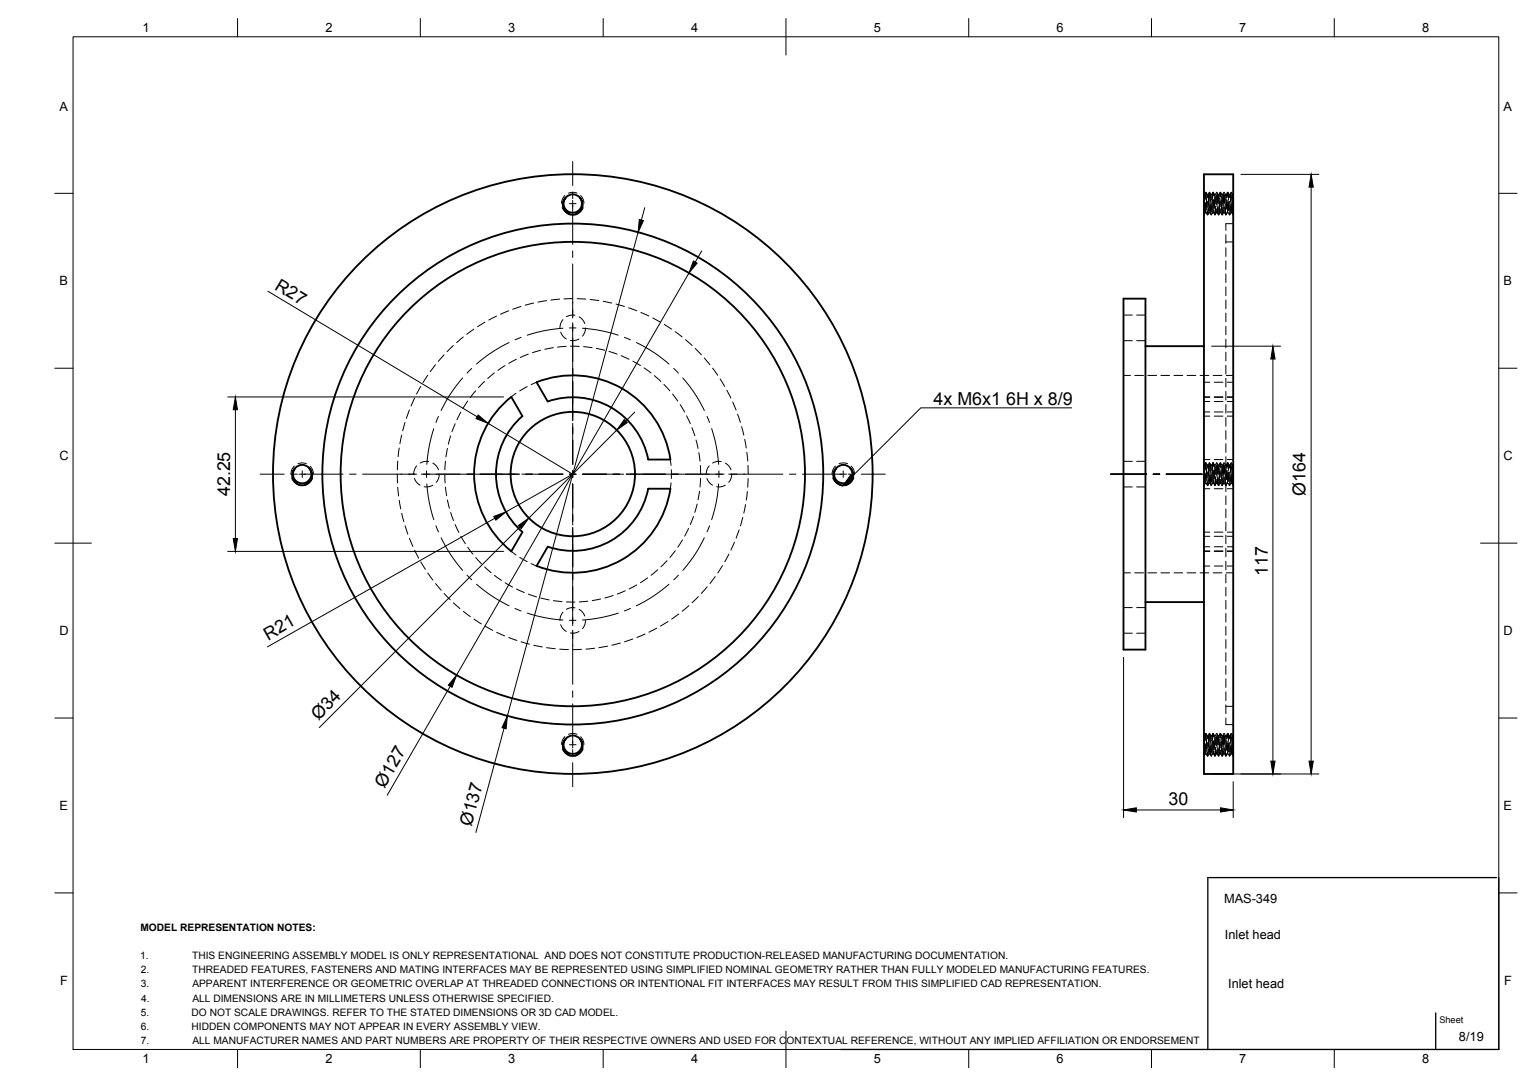
ISO-10303-21;
HEADER;
/* Generated by software containing ST-Developer
 * from STEP Tools, Inc. (www.steptools.com) 
 */

FILE_DESCRIPTION(
/* description */ ('Independent two-stage semi-open centrifugal-pump CAD. Shared impeller
s, open-machinable return casings, removable diaphragms, bronze wear/j
ournal rings, volume-preserving seal instances, retained keyed shaft, 
opposed mechanical face rings and partly threaded tie hardware. Native
 shaft rotation. Geometric topology/clearance only; flow/head/efficien
cy, pressure, cavitation, balance, preload, face loading and secondary
 seal fits/bonds, material/thermal/tolerance selection and life unassi
gned. External drive, coupling, anchors and piping bolts omitted.'),
/* implementation_level */ '2;1');

FILE_NAME(
/* name */ 'Inlet head.step',
/* time_stamp */ '2026-11-08T18:06:32-08:00',
/* author */ (''),
/* organization */ (''),
/* preprocessor_version */ 'ST-DEVELOPER v20.2',
/* originating_system */ 'Autodesk Translation Framework v15.17.0.0',
/* authorisation */ '');

FILE_SCHEMA (('AUTOMOTIVE_DESIGN { 1 0 10303 214 3 1 1 }'));
ENDSEC;

DATA;
#10=MECHANICAL_DESIGN_GEOMETRIC_PRESENTATION_REPRESENTATION('',(#397),#16687);
#138=B_SPLINE_SURFACE_WITH_KNOTS('',3,3,((#11457,#11458,#11459,#11460,#11461,
#11462,#11463,#11464,#11465,#11466,#11467,#11468,#11469,#11470,#11471,#11472,
#11473,#11474,#11475,#11476,#11477,#11478,#11479,#11480,#11481,#11482,#11483,
#11484,#11485,#11486,#11487,#11488,#11489,#11490,#11491,#11492,#11493,#11494,
#11495,#11496,#11497,#11498,#11499,#11500,#11501,#11502,#11503,#11504,#11505,
#11506,#11507,#11508,#11509,#11510,#11511,#11512),(#11513,#11514,#11515,
#11516,#11517,#11518,#11519,#11520,#11521,#11522,#11523,#11524,#11525,#11526,
#11527,#11528,#11529,#11530,#11531,#11532,#11533,#11534,#11535,#11536,#11537,
#11538,#11539,#11540,#11541,#11542,#11543,#11544,#11545,#11546,#11547,#11548,
#11549,#11550,#11551,#11552,#11553,#11554,#11555,#11556,#11557,#11558,#11559,
#11560,#11561,#11562,#11563,#11564,#11565,#11566,#11567,#11568),(#11569,
#11570,#11571,#11572,#11573,#11574,#11575,#11576,#11577,#11578,#11579,#11580,
#11581,#11582,#11583,#11584,#11585,#11586,#11587,#11588,#11589,#11590,#11591,
#11592,#11593,#11594,#11595,#11596,#11597,#11598,#11599,#11600,#11601,#11602,
#11603,#11604,#11605,#11606,#11607,#11608,#11609,#11610,#11611,#11612,#11613,
#11614,#11615,#11616,#11617,#11618,#11619,#11620,#11621,#11622,#11623,#11624),
(#11625,#11626,#11627,#11628,#11629,#11630,#11631,#11632,#11633,#11634,
#11635,#11636,#11637,#11638,#11639,#11640,#11641,#11642,#11643,#11644,#11645,
#11646,#11647,#11648,#11649,#11650,#11651,#11652,#11653,#11654,#11655,#11656,
#11657,#11658,#11659,#11660,#11661,#11662,#11663,#11664,#11665,#11666,#11667,
#11668,#11669,#11670,#11671,#11672,#11673,#11674,#11675,#11676,#11677,#11678,
#11679,#11680)),.UNSPECIFIED.,.F.,.F.,.F.,(4,4),(4,1,1,1,1,1,1,1,1,1,1,
1,1,1,1,1,1,1,1,1,1,1,1,1,1,1,1,1,1,1,1,1,1,1,1,1,1,1,1,1,1,1,1,1,1,1,1,
1,1,1,1,1,1,4),(0.,0.0642013499338864),(11.8589888623078,12.8454497557128,
13.8319106491178,14.8183715425228,15.8048324359278,16.7912933293328,17.7777542227378,
18.7642151161428,19.7506760095478,20.7371369029528,21.7235977963578,22.7100586897628,
23.6965195831678,24.6829804765729,25.6694413699779,26.6559022633829,27.6423631567879,
28.6288240501929,29.6152849435979,30.6017458370029,31.5882067304079,32.5746676238129,
33.5611285172179,34.5475894106229,35.5340503040279,36.5205111974329,37.5069720908379,
38.4934329842429,39.4798938776479,40.4663547710529,41.4528156644579,42.4392765578629,
43.4257374512679,44.4121983446729,45.3986592380779,46.3851201314829,47.3715810248879,
48.3580419182929,49.3445028116979,50.3309637051029,51.3174245985079,52.3038854919129,
53.2903463853179,54.2768072787229,55.2632681721279,56.2497290655329,57.2361899589379,
58.222650852343,59.209111745748,60.195572639153,61.182033532558,62.168494425963,
63.154955319368,64.141416212773),.UNSPECIFIED.);
#139=B_SPLINE_SURFACE_WITH_KNOTS('',3,3,((#11822,#11823,#11824,#11825,#11826,
#11827,#11828,#11829,#11830,#11831,#11832,#11833,#11834,#11835,#11836,#11837,
#11838,#11839,#11840,#11841,#11842,#11843,#11844,#11845,#11846,#11847,#11848,
#11849,#11850,#11851,#11852,#11853,#11854,#11855,#11856,#11857,#11858,#11859,
#11860,#11861,#11862,#11863,#11864,#11865,#11866,#11867,#11868,#11869,#11870,
#11871,#11872,#11873,#11874,#11875,#11876,#11877),(#11878,#11879,#11880,
#11881,#11882,#11883,#11884,#11885,#11886,#11887,#11888,#11889,#11890,#11891,
#11892,#11893,#11894,#11895,#11896,#11897,#11898,#11899,#11900,#11901,#11902,
#11903,#11904,#11905,#11906,#11907,#11908,#11909,#11910,#11911,#11912,#11913,
#11914,#11915,#11916,#11917,#11918,#11919,#11920,#11921,#11922,#11923,#11924,
#11925,#11926,#11927,#11928,#11929,#11930,#11931,#11932,#11933),(#11934,
#11935,#11936,#11937,#11938,#11939,#11940,#11941,#11942,#11943,#11944,#11945,
#11946,#11947,#11948,#11949,#11950,#11951,#11952,#11953,#11954,#11955,#11956,
#11957,#11958,#11959,#11960,#11961,#11962,#11963,#11964,#11965,#11966,#11967,
#11968,#11969,#11970,#11971,#11972,#11973,#11974,#11975,#11976,#11977,#11978,
#11979,#11980,#11981,#11982,#11983,#11984,#11985,#11986,#11987,#11988,#11989),
(#11990,#11991,#11992,#11993,#11994,#11995,#11996,#11997,#11998,#11999,
#12000,#12001,#12002,#12003,#12004,#12005,#12006,#12007,#12008,#12009,#12010,
#12011,#12012,#12013,#12014,#12015,#12016,#12017,#12018,#12019,#12020,#12021,
#12022,#12023,#12024,#12025,#12026,#12027,#12028,#12029,#12030,#12031,#12032,
#12033,#12034,#12035,#12036,#12037,#12038,#12039,#12040,#12041,#12042,#12043,
#12044,#12045)),.UNSPECIFIED.,.F.,.F.,.F.,(4,4),(4,1,1,1,1,1,1,1,1,1,1,
1,1,1,1,1,1,1,1,1,1,1,1,1,1,1,1,1,1,1,1,1,1,1,1,1,1,1,1,1,1,1,1,1,1,1,1,
1,1,1,1,1,1,4),(0.,0.0642013499338864),(14.3984001269718,15.3848610203768,
16.3713219137818,17.3577828071869,18.3442437005919,19.3307045939969,20.3171654874019,
21.3036263808069,22.2900872742119,23.2765481676169,24.2630090610219,25.2494699544269,
26.2359308478319,27.2223917412369,28.2088526346419,29.1953135280469,30.1817744214519,
31.1682353148569,32.1546962082619,33.1411571016669,34.1276179950719,35.1140788884769,
36.1005397818819,37.0870006752869,38.0734615686919,39.0599224620969,40.0463833555019,
41.0328442489069,42.0193051423119,43.0057660357169,43.9922269291219,44.9786878225269,
45.9651487159319,46.9516096093369,47.9380705027419,48.9245313961469,49.9109922895519,
50.8974531829569,51.8839140763619,52.8703749697669,53.856835863172,54.843296756577,
55.829757649982,56.816218543387,57.802679436792,58.789140330197,59.775601223602,
60.762062117007,61.748523010412,62.734983903817,63.721444797222,64.707905690627,
65.694366584032,66.680827477437),.UNSPECIFIED.);
#140=B_SPLINE_SURFACE_WITH_KNOTS('',3,3,((#12562,#12563,#12564,#12565,#12566,
#12567,#12568,#12569,#12570,#12571,#12572,#12573,#12574,#12575,#12576,#12577,
#12578,#12579,#12580,#12581,#12582,#12583,#12584,#12585,#12586,#12587,#12588,
#12589,#12590,#12591,#12592,#12593,#12594,#12595,#12596,#12597,#12598,#12599,
#12600,#12601,#12602,#12603,#12604,#12605,#12606,#12607,#12608,#12609,#12610,
#12611,#12612,#12613,#12614,#12615,#12616,#12617),(#12618,#12619,#12620,
#12621,#12622,#12623,#12624,#12625,#12626,#12627,#12628,#12629,#12630,#12631,
#12632,#12633,#12634,#12635,#12636,#12637,#12638,#12639,#12640,#12641,#12642,
#12643,#12644,#12645,#12646,#12647,#12648,#12649,#12650,#12651,#12652,#12653,
#12654,#12655,#12656,#12657,#12658,#12659,#12660,#12661,#12662,#12663,#12664,
#12665,#12666,#12667,#12668,#12669,#12670,#12671,#12672,#12673),(#12674,
#12675,#12676,#12677,#12678,#12679,#12680,#12681,#12682,#12683,#12684,#12685,
#12686,#12687,#12688,#12689,#12690,#12691,#12692,#12693,#12694,#12695,#12696,
#12697,#12698,#12699,#12700,#12701,#12702,#12703,#12704,#12705,#12706,#12707,
#12708,#12709,#12710,#12711,#12712,#12713,#12714,#12715,#12716,#12717,#12718,
#12719,#12720,#12721,#12722,#12723,#12724,#12725,#12726,#12727,#12728,#12729),
(#12730,#12731,#12732,#12733,#12734,#12735,#12736,#12737,#12738,#12739,
#12740,#12741,#12742,#12743,#12744,#12745,#12746,#12747,#12748,#12749,#12750,
#12751,#12752,#12753,#12754,#12755,#12756,#12757,#12758,#12759,#12760,#12761,
#12762,#12763,#12764,#12765,#12766,#12767,#12768,#12769,#12770,#12771,#12772,
#12773,#12774,#12775,#12776,#12777,#12778,#12779,#12780,#12781,#12782,#12783,
#12784,#12785)),.UNSPECIFIED.,.F.,.F.,.F.,(4,4),(4,1,1,1,1,1,1,1,1,1,1,
1,1,1,1,1,1,1,1,1,1,1,1,1,1,1,1,1,1,1,1,1,1,1,1,1,1,1,1,1,1,1,1,1,1,1,1,
1,1,1,1,1,1,4),(0.,0.0642013499338865),(11.8589888623078,12.8454497557128,
13.8319106491178,14.8183715425228,15.8048324359278,16.7912933293328,17.7777542227378,
18.7642151161428,19.7506760095478,20.7371369029528,21.7235977963578,22.7100586897628,
23.6965195831678,24.6829804765728,25.6694413699778,26.6559022633828,27.6423631567879,
28.6288240501929,29.6152849435979,30.6017458370029,31.5882067304079,32.5746676238129,
33.5611285172179,34.5475894106229,35.5340503040279,36.5205111974329,37.5069720908379,
38.4934329842429,39.4798938776479,40.4663547710529,41.4528156644579,42.4392765578629,
43.4257374512679,44.4121983446729,45.3986592380779,46.3851201314829,47.3715810248879,
48.3580419182929,49.3445028116979,50.3309637051029,51.3174245985079,52.3038854919129,
53.2903463853179,54.2768072787229,55.2632681721279,56.2497290655329,57.2361899589379,
58.2226508523429,59.2091117457479,60.1955726391529,61.1820335325579,62.1684944259629,
63.154955319368,64.141416212773),.UNSPECIFIED.);
#141=B_SPLINE_SURFACE_WITH_KNOTS('',3,3,((#12869,#12870,#12871,#12872,#12873,
#12874,#12875,#12876,#12877,#12878,#12879,#12880,#12881,#12882,#12883,#12884,
#12885,#12886,#12887,#12888,#12889,#12890,#12891,#12892,#12893,#12894,#12895,
#12896,#12897,#12898,#12899,#12900,#12901,#12902,#12903,#12904,#12905,#12906,
#12907,#12908,#12909,#12910,#12911,#12912,#12913,#12914,#12915,#12916,#12917,
#12918,#12919,#12920,#12921,#12922,#12923,#12924),(#12925,#12926,#12927,
#12928,#12929,#12930,#12931,#12932,#12933,#12934,#12935,#12936,#12937,#12938,
#12939,#12940,#12941,#12942,#12943,#12944,#12945,#12946,#12947,#12948,#12949,
#12950,#12951,#12952,#12953,#12954,#12955,#12956,#12957,#12958,#12959,#12960,
#12961,#12962,#12963,#12964,#12965,#12966,#12967,#12968,#12969,#12970,#12971,
#12972,#12973,#12974,#12975,#12976,#12977,#12978,#12979,#12980),(#12981,
#12982,#12983,#12984,#12985,#12986,#12987,#12988,#12989,#12990,#12991,#12992,
#12993,#12994,#12995,#12996,#12997,#12998,#12999,#13000,#13001,#13002,#13003,
#13004,#13005,#13006,#13007,#13008,#13009,#13010,#13011,#13012,#13013,#13014,
#13015,#13016,#13017,#13018,#13019,#13020,#13021,#13022,#13023,#13024,#13025,
#13026,#13027,#13028,#13029,#13030,#13031,#13032,#13033,#13034,#13035,#13036),
(#13037,#13038,#13039,#13040,#13041,#13042,#13043,#13044,#13045,#13046,
#13047,#13048,#13049,#13050,#13051,#13052,#13053,#13054,#13055,#13056,#13057,
#13058,#13059,#13060,#13061,#13062,#13063,#13064,#13065,#13066,#13067,#13068,
#13069,#13070,#13071,#13072,#13073,#13074,#13075,#13076,#13077,#13078,#13079,
#13080,#13081,#13082,#13083,#13084,#13085,#13086,#13087,#13088,#13089,#13090,
#13091,#13092)),.UNSPECIFIED.,.F.,.F.,.F.,(4,4),(4,1,1,1,1,1,1,1,1,1,1,
1,1,1,1,1,1,1,1,1,1,1,1,1,1,1,1,1,1,1,1,1,1,1,1,1,1,1,1,1,1,1,1,1,1,1,1,
1,1,1,1,1,1,4),(0.,0.0642013499338865),(14.3984001269718,15.3848610203768,
16.3713219137818,17.3577828071869,18.3442437005919,19.3307045939969,20.3171654874019,
21.3036263808069,22.2900872742119,23.2765481676169,24.2630090610219,25.2494699544269,
26.2359308478319,27.2223917412369,28.2088526346419,29.1953135280469,30.1817744214519,
31.1682353148569,32.1546962082619,33.1411571016669,34.1276179950719,35.1140788884769,
36.1005397818819,37.0870006752869,38.0734615686919,39.0599224620969,40.0463833555019,
41.0328442489069,42.0193051423119,43.0057660357169,43.9922269291219,44.9786878225269,
45.9651487159319,46.9516096093369,47.9380705027419,48.9245313961469,49.9109922895519,
50.8974531829569,51.8839140763619,52.8703749697669,53.8568358631719,54.8432967565769,
55.8297576499819,56.816218543387,57.802679436792,58.789140330197,59.775601223602,
60.762062117007,61.748523010412,62.734983903817,63.721444797222,64.707905690627,
65.694366584032,66.680827477437),.UNSPECIFIED.);
#142=B_SPLINE_SURFACE_WITH_KNOTS('',3,3,((#13198,#13199,#13200,#13201,#13202,
#13203,#13204,#13205,#13206,#13207,#13208,#13209,#13210,#13211,#13212,#13213,
#13214,#13215,#13216,#13217,#13218,#13219,#13220,#13221,#13222,#13223,#13224,
#13225,#13226,#13227,#13228,#13229,#13230,#13231,#13232,#13233,#13234,#13235,
#13236,#13237,#13238,#13239,#13240,#13241,#13242,#13243,#13244,#13245,#13246,
#13247,#13248,#13249,#13250,#13251,#13252,#13253),(#13254,#13255,#13256,
#13257,#13258,#13259,#13260,#13261,#13262,#13263,#13264,#13265,#13266,#13267,
#13268,#13269,#13270,#13271,#13272,#13273,#13274,#13275,#13276,#13277,#13278,
#13279,#13280,#13281,#13282,#13283,#13284,#13285,#13286,#13287,#13288,#13289,
#13290,#13291,#13292,#13293,#13294,#13295,#13296,#13297,#13298,#13299,#13300,
#13301,#13302,#13303,#13304,#13305,#13306,#13307,#13308,#13309),(#13310,
#13311,#13312,#13313,#13314,#13315,#13316,#13317,#13318,#13319,#13320,#13321,
#13322,#13323,#13324,#13325,#13326,#13327,#13328,#13329,#13330,#13331,#13332,
#13333,#13334,#13335,#13336,#13337,#13338,#13339,#13340,#13341,#13342,#13343,
#13344,#13345,#13346,#13347,#13348,#13349,#13350,#13351,#13352,#13353,#13354,
#13355,#13356,#13357,#13358,#13359,#13360,#13361,#13362,#13363,#13364,#13365),
(#13366,#13367,#13368,#13369,#13370,#13371,#13372,#13373,#13374,#13375,
#13376,#13377,#13378,#13379,#13380,#13381,#13382,#13383,#13384,#13385,#13386,
#13387,#13388,#13389,#13390,#13391,#13392,#13393,#13394,#13395,#13396,#13397,
#13398,#13399,#13400,#13401,#13402,#13403,#13404,#13405,#13406,#13407,#13408,
#13409,#13410,#13411,#13412,#13413,#13414,#13415,#13416,#13417,#13418,#13419,
#13420,#13421)),.UNSPECIFIED.,.F.,.F.,.F.,(4,4),(4,1,1,1,1,1,1,1,1,1,1,
1,1,1,1,1,1,1,1,1,1,1,1,1,1,1,1,1,1,1,1,1,1,1,1,1,1,1,1,1,1,1,1,1,1,1,1,
1,1,1,1,1,1,4),(0.,0.0642013499338865),(11.8589888623078,12.8454497557128,
13.8319106491178,14.8183715425228,15.8048324359278,16.7912933293328,17.7777542227378,
18.7642151161428,19.7506760095478,20.7371369029528,21.7235977963578,22.7100586897628,
23.6965195831678,24.6829804765728,25.6694413699778,26.6559022633828,27.6423631567879,
28.6288240501929,29.6152849435979,30.6017458370029,31.5882067304079,32.5746676238129,
33.5611285172179,34.5475894106229,35.5340503040279,36.5205111974329,37.5069720908379,
38.4934329842429,39.4798938776479,40.4663547710529,41.4528156644579,42.4392765578629,
43.4257374512679,44.4121983446729,45.3986592380779,46.3851201314829,47.3715810248879,
48.3580419182929,49.3445028116979,50.3309637051029,51.3174245985079,52.3038854919129,
53.2903463853179,54.2768072787229,55.2632681721279,56.2497290655329,57.2361899589379,
58.2226508523429,59.2091117457479,60.1955726391529,61.1820335325579,62.1684944259629,
63.154955319368,64.141416212773),.UNSPECIFIED.);
#143=B_SPLINE_SURFACE_WITH_KNOTS('',3,3,((#13505,#13506,#13507,#13508,#13509,
#13510,#13511,#13512,#13513,#13514,#13515,#13516,#13517,#13518,#13519,#13520,
#13521,#13522,#13523,#13524,#13525,#13526,#13527,#13528,#13529,#13530,#13531,
#13532,#13533,#13534,#13535,#13536,#13537,#13538,#13539,#13540,#13541,#13542,
#13543,#13544,#13545,#13546,#13547,#13548,#13549,#13550,#13551,#13552,#13553,
#13554,#13555,#13556,#13557,#13558,#13559,#13560),(#13561,#13562,#13563,
#13564,#13565,#13566,#13567,#13568,#13569,#13570,#13571,#13572,#13573,#13574,
#13575,#13576,#13577,#13578,#13579,#13580,#13581,#13582,#13583,#13584,#13585,
#13586,#13587,#13588,#13589,#13590,#13591,#13592,#13593,#13594,#13595,#13596,
#13597,#13598,#13599,#13600,#13601,#13602,#13603,#13604,#13605,#13606,#13607,
#13608,#13609,#13610,#13611,#13612,#13613,#13614,#13615,#13616),(#13617,
#13618,#13619,#13620,#13621,#13622,#13623,#13624,#13625,#13626,#13627,#13628,
#13629,#13630,#13631,#13632,#13633,#13634,#13635,#13636,#13637,#13638,#13639,
#13640,#13641,#13642,#13643,#13644,#13645,#13646,#13647,#13648,#13649,#13650,
#13651,#13652,#13653,#13654,#13655,#13656,#13657,#13658,#13659,#13660,#13661,
#13662,#13663,#13664,#13665,#13666,#13667,#13668,#13669,#13670,#13671,#13672),
(#13673,#13674,#13675,#13676,#13677,#13678,#13679,#13680,#13681,#13682,
#13683,#13684,#13685,#13686,#13687,#13688,#13689,#13690,#13691,#13692,#13693,
#13694,#13695,#13696,#13697,#13698,#13699,#13700,#13701,#13702,#13703,#13704,
#13705,#13706,#13707,#13708,#13709,#13710,#13711,#13712,#13713,#13714,#13715,
#13716,#13717,#13718,#13719,#13720,#13721,#13722,#13723,#13724,#13725,#13726,
#13727,#13728)),.UNSPECIFIED.,.F.,.F.,.F.,(4,4),(4,1,1,1,1,1,1,1,1,1,1,
1,1,1,1,1,1,1,1,1,1,1,1,1,1,1,1,1,1,1,1,1,1,1,1,1,1,1,1,1,1,1,1,1,1,1,1,
1,1,1,1,1,1,4),(0.,0.0642013499338865),(14.3984001269718,15.3848610203768,
16.3713219137818,17.3577828071869,18.3442437005919,19.3307045939969,20.3171654874019,
21.3036263808069,22.2900872742119,23.2765481676169,24.2630090610219,25.2494699544269,
26.2359308478319,27.2223917412369,28.2088526346419,29.1953135280469,30.1817744214519,
31.1682353148569,32.1546962082619,33.1411571016669,34.1276179950719,35.1140788884769,
36.1005397818819,37.0870006752869,38.0734615686919,39.0599224620969,40.0463833555019,
41.0328442489069,42.0193051423119,43.0057660357169,43.9922269291219,44.9786878225269,
45.9651487159319,46.9516096093369,47.9380705027419,48.9245313961469,49.9109922895519,
50.8974531829569,51.8839140763619,52.8703749697669,53.856835863172,54.843296756577,
55.829757649982,56.816218543387,57.802679436792,58.789140330197,59.775601223602,
60.762062117007,61.748523010412,62.734983903817,63.721444797222,64.707905690627,
65.694366584032,66.680827477437),.UNSPECIFIED.);
#144=B_SPLINE_SURFACE_WITH_KNOTS('',3,3,((#13834,#13835,#13836,#13837,#13838,
#13839,#13840,#13841,#13842,#13843,#13844,#13845,#13846,#13847,#13848,#13849,
#13850,#13851,#13852,#13853,#13854,#13855,#13856,#13857,#13858,#13859,#13860,
#13861,#13862,#13863,#13864,#13865,#13866,#13867,#13868,#13869,#13870,#13871,
#13872,#13873,#13874,#13875,#13876,#13877,#13878,#13879,#13880,#13881,#13882,
#13883,#13884,#13885,#13886,#13887,#13888,#13889),(#13890,#13891,#13892,
#13893,#13894,#13895,#13896,#13897,#13898,#13899,#13900,#13901,#13902,#13903,
#13904,#13905,#13906,#13907,#13908,#13909,#13910,#13911,#13912,#13913,#13914,
#13915,#13916,#13917,#13918,#13919,#13920,#13921,#13922,#13923,#13924,#13925,
#13926,#13927,#13928,#13929,#13930,#13931,#13932,#13933,#13934,#13935,#13936,
#13937,#13938,#13939,#13940,#13941,#13942,#13943,#13944,#13945),(#13946,
#13947,#13948,#13949,#13950,#13951,#13952,#13953,#13954,#13955,#13956,#13957,
#13958,#13959,#13960,#13961,#13962,#13963,#13964,#13965,#13966,#13967,#13968,
#13969,#13970,#13971,#13972,#13973,#13974,#13975,#13976,#13977,#13978,#13979,
#13980,#13981,#13982,#13983,#13984,#13985,#13986,#13987,#13988,#13989,#13990,
#13991,#13992,#13993,#13994,#13995,#13996,#13997,#13998,#13999,#14000,#14001),
(#14002,#14003,#14004,#14005,#14006,#14007,#14008,#14009,#14010,#14011,
#14012,#14013,#14014,#14015,#14016,#14017,#14018,#14019,#14020,#14021,#14022,
#14023,#14024,#14025,#14026,#14027,#14028,#14029,#14030,#14031,#14032,#14033,
#14034,#14035,#14036,#14037,#14038,#14039,#14040,#14041,#14042,#14043,#14044,
#14045,#14046,#14047,#14048,#14049,#14050,#14051,#14052,#14053,#14054,#14055,
#14056,#14057)),.UNSPECIFIED.,.F.,.F.,.F.,(4,4),(4,1,1,1,1,1,1,1,1,1,1,
1,1,1,1,1,1,1,1,1,1,1,1,1,1,1,1,1,1,1,1,1,1,1,1,1,1,1,1,1,1,1,1,1,1,1,1,
1,1,1,1,1,1,4),(0.,0.0642013499338864),(11.8589888623078,12.8454497557128,
13.8319106491178,14.8183715425228,15.8048324359278,16.7912933293328,17.7777542227378,
18.7642151161428,19.7506760095478,20.7371369029528,21.7235977963578,22.7100586897628,
23.6965195831678,24.6829804765729,25.6694413699779,26.6559022633829,27.6423631567879,
28.6288240501929,29.6152849435979,30.6017458370029,31.5882067304079,32.5746676238129,
33.5611285172179,34.5475894106229,35.5340503040279,36.5205111974329,37.5069720908379,
38.4934329842429,39.4798938776479,40.4663547710529,41.4528156644579,42.4392765578629,
43.4257374512679,44.4121983446729,45.3986592380779,46.3851201314829,47.3715810248879,
48.3580419182929,49.3445028116979,50.3309637051029,51.3174245985079,52.3038854919129,
53.2903463853179,54.2768072787229,55.2632681721279,56.2497290655329,57.2361899589379,
58.222650852343,59.209111745748,60.195572639153,61.182033532558,62.168494425963,
63.154955319368,64.141416212773),.UNSPECIFIED.);
#145=B_SPLINE_SURFACE_WITH_KNOTS('',3,3,((#14141,#14142,#14143,#14144,#14145,
#14146,#14147,#14148,#14149,#14150,#14151,#14152,#14153,#14154,#14155,#14156,
#14157,#14158,#14159,#14160,#14161,#14162,#14163,#14164,#14165,#14166,#14167,
#14168,#14169,#14170,#14171,#14172,#14173,#14174,#14175,#14176,#14177,#14178,
#14179,#14180,#14181,#14182,#14183,#14184,#14185,#14186,#14187,#14188,#14189,
#14190,#14191,#14192,#14193,#14194,#14195,#14196),(#14197,#14198,#14199,
#14200,#14201,#14202,#14203,#14204,#14205,#14206,#14207,#14208,#14209,#14210,
#14211,#14212,#14213,#14214,#14215,#14216,#14217,#14218,#14219,#14220,#14221,
#14222,#14223,#14224,#14225,#14226,#14227,#14228,#14229,#14230,#14231,#14232,
#14233,#14234,#14235,#14236,#14237,#14238,#14239,#14240,#14241,#14242,#14243,
#14244,#14245,#14246,#14247,#14248,#14249,#14250,#14251,#14252),(#14253,
#14254,#14255,#14256,#14257,#14258,#14259,#14260,#14261,#14262,#14263,#14264,
#14265,#14266,#14267,#14268,#14269,#14270,#14271,#14272,#14273,#14274,#14275,
#14276,#14277,#14278,#14279,#14280,#14281,#14282,#14283,#14284,#14285,#14286,
#14287,#14288,#14289,#14290,#14291,#14292,#14293,#14294,#14295,#14296,#14297,
#14298,#14299,#14300,#14301,#14302,#14303,#14304,#14305,#14306,#14307,#14308),
(#14309,#14310,#14311,#14312,#14313,#14314,#14315,#14316,#14317,#14318,
#14319,#14320,#14321,#14322,#14323,#14324,#14325,#14326,#14327,#14328,#14329,
#14330,#14331,#14332,#14333,#14334,#14335,#14336,#14337,#14338,#14339,#14340,
#14341,#14342,#14343,#14344,#14345,#14346,#14347,#14348,#14349,#14350,#14351,
#14352,#14353,#14354,#14355,#14356,#14357,#14358,#14359,#14360,#14361,#14362,
#14363,#14364)),.UNSPECIFIED.,.F.,.F.,.F.,(4,4),(4,1,1,1,1,1,1,1,1,1,1,
1,1,1,1,1,1,1,1,1,1,1,1,1,1,1,1,1,1,1,1,1,1,1,1,1,1,1,1,1,1,1,1,1,1,1,1,
1,1,1,1,1,1,4),(0.,0.0642013499338864),(14.3984001269718,15.3848610203768,
16.3713219137818,17.3577828071869,18.3442437005919,19.3307045939969,20.3171654874019,
21.3036263808069,22.2900872742119,23.2765481676169,24.2630090610219,25.2494699544269,
26.2359308478319,27.2223917412369,28.2088526346419,29.1953135280469,30.1817744214519,
31.1682353148569,32.1546962082619,33.1411571016669,34.1276179950719,35.1140788884769,
36.1005397818819,37.0870006752869,38.0734615686919,39.0599224620969,40.0463833555019,
41.0328442489069,42.0193051423119,43.0057660357169,43.9922269291219,44.9786878225269,
45.9651487159319,46.9516096093369,47.9380705027419,48.9245313961469,49.9109922895519,
50.8974531829569,51.8839140763619,52.8703749697669,53.856835863172,54.843296756577,
55.829757649982,56.816218543387,57.802679436792,58.789140330197,59.775601223602,
60.762062117007,61.748523010412,62.734983903817,63.721444797222,64.707905690627,
65.694366584032,66.680827477437),.UNSPECIFIED.);
#148=B_SPLINE_CURVE_WITH_KNOTS('',3,(#9202,#9203,#9204,#9205),
 .UNSPECIFIED.,.F.,.F.,(4,4),(51.5750455984138,52.2824273504652),
 .UNSPECIFIED.);
#149=B_SPLINE_CURVE_WITH_KNOTS('',3,(#9208,#9209,#9210,#9211,#9212,#9213,
#9214,#9215,#9216,#9217),.UNSPECIFIED.,.F.,.F.,(4,3,3,4),(-50.2654824574367,
-49.3230446702501,-48.3365837768451,-47.8312715558983),.UNSPECIFIED.);
#150=B_SPLINE_CURVE_WITH_KNOTS('',3,(#9222,#9223,#9224,#9225,#9226,#9227,
#9228,#9229,#9230,#9231,#9232,#9233,#9234,#9235,#9236,#9237,#9238,#9239,
#9240,#9241,#9242,#9243,#9244,#9245,#9246),.UNSPECIFIED.,.F.,.F.,(4,3,3,
3,3,3,3,3,4),(45.2918602912342,45.3772010966301,46.3636619900351,47.3501228834401,
48.3365837768451,49.3230446702501,50.3095055636551,51.2959664570601,51.5750455984138),
 .UNSPECIFIED.);
#151=B_SPLINE_CURVE_WITH_KNOTS('',3,(#9247,#9248,#9249,#9250,#9251,#9252,
#9253,#9254,#9255,#9256,#9257,#9258,#9259,#9260,#9261,#9262,#9263,#9264,
#9265,#9266,#9267,#9268),.UNSPECIFIED.,.F.,.F.,(4,3,3,3,3,3,3,4),(-47.8312715558983,
-47.3501228834401,-46.3636619900351,-45.3772010966301,-44.3907402032251,
-43.4042793098201,-42.4178184164151,-41.5480862487187),.UNSPECIFIED.);
#152=B_SPLINE_CURVE_WITH_KNOTS('',3,(#9273,#9274,#9275,#9276,#9277,#9278,
#9279,#9280,#9281,#9282,#9283,#9284,#9285,#9286,#9287,#9288,#9289,#9290,
#9291,#9292,#9293,#9294),.UNSPECIFIED.,.F.,.F.,(4,3,3,3,3,3,3,4),(39.0086749840546,
39.4584357362001,40.4448966296051,41.4313575230101,42.4178184164151,43.4042793098201,
44.3907402032251,45.2918602912342),.UNSPECIFIED.);
#153=B_SPLINE_CURVE_WITH_KNOTS('',3,(#9295,#9296,#9297,#9298,#9299,#9300,
#9301,#9302,#9303,#9304,#9305,#9306,#9307,#9308,#9309,#9310,#9311,#9312,
#9313,#9314,#9315,#9316,#9317,#9318,#9319),.UNSPECIFIED.,.F.,.F.,(4,3,3,
3,3,3,3,3,4),(-41.5480862487187,-41.4313575230101,-40.4448966296051,-39.4584357362001,
-38.4719748427951,-37.4855139493901,-36.4990530559851,-35.5125921625801,
-35.2649009415391),.UNSPECIFIED.);
#154=B_SPLINE_CURVE_WITH_KNOTS('',3,(#9324,#9325,#9326,#9327,#9328,#9329,
#9330,#9331,#9332,#9333,#9334,#9335,#9336,#9337,#9338,#9339,#9340,#9341,
#9342,#9343,#9344,#9345),.UNSPECIFIED.,.F.,.F.,(4,3,3,3,3,3,3,4),(32.725489676875,
33.5396703757701,34.5261312691751,35.5125921625801,36.4990530559851,37.4855139493901,
38.4719748427951,39.0086749840546),.UNSPECIFIED.);
#155=B_SPLINE_CURVE_WITH_KNOTS('',3,(#9346,#9347,#9348,#9349,#9350,#9351,
#9352,#9353,#9354,#9355,#9356,#9357,#9358,#9359,#9360,#9361,#9362,#9363,
#9364,#9365,#9366,#9367),.UNSPECIFIED.,.F.,.F.,(4,3,3,3,3,3,3,4),(-35.2649009415391,
-34.5261312691751,-33.5396703757701,-32.5532094823651,-31.5667485889601,
-30.5802876955551,-29.5938268021501,-28.9817156343595),.UNSPECIFIED.);
#156=B_SPLINE_CURVE_WITH_KNOTS('',3,(#9372,#9373,#9374,#9375,#9376,#9377,
#9378,#9379,#9380,#9381,#9382,#9383,#9384,#9385,#9386,#9387,#9388,#9389,
#9390,#9391,#9392,#9393,#9394,#9395,#9396),.UNSPECIFIED.,.F.,.F.,(4,3,3,
3,3,3,3,3,4),(26.4423043696954,26.6344441219351,27.6209050153401,28.6073659087451,
29.5938268021501,30.5802876955551,31.5667485889601,32.5532094823651,32.725489676875),
 .UNSPECIFIED.);
#157=B_SPLINE_CURVE_WITH_KNOTS('',3,(#9397,#9398,#9399,#9400,#9401,#9402,
#9403,#9404,#9405,#9406,#9407,#9408,#9409,#9410,#9411,#9412,#9413,#9414,
#9415,#9416,#9417,#9418),.UNSPECIFIED.,.F.,.F.,(4,3,3,3,3,3,3,4),(-28.9817156343595,
-28.6073659087451,-27.6209050153401,-26.6344441219351,-25.6479832285301,
-24.6615223351251,-23.6750614417201,-22.6985303271799),.UNSPECIFIED.);
#158=B_SPLINE_CURVE_WITH_KNOTS('',3,(#9423,#9424,#9425,#9426,#9427,#9428,
#9429,#9430,#9431,#9432,#9433,#9434,#9435,#9436,#9437,#9438,#9439,#9440,
#9441,#9442,#9443,#9444),.UNSPECIFIED.,.F.,.F.,(4,3,3,3,3,3,3,4),(20.1591190625159,
20.7156787615051,21.7021396549101,22.6886005483151,23.6750614417201,24.6615223351251,
25.6479832285301,26.4423043696954),.UNSPECIFIED.);
#159=B_SPLINE_CURVE_WITH_KNOTS('',3,(#9445,#9446,#9447,#9448,#9449,#9450,
#9451,#9452,#9453,#9454,#9455,#9456,#9457,#9458,#9459,#9460,#9461,#9462,
#9463,#9464,#9465,#9466,#9467,#9468,#9469),.UNSPECIFIED.,.F.,.F.,(4,3,3,
3,3,3,3,3,4),(-22.6985303271799,-22.6886005483151,-21.7021396549101,-20.7156787615051,
-19.7292178681001,-18.7427569746951,-17.75629608129,-16.7698351878851,-16.4153450200003),
 .UNSPECIFIED.);
#160=B_SPLINE_CURVE_WITH_KNOTS('',3,(#9474,#9475,#9476,#9477,#9478,#9479,
#9480,#9481,#9482,#9483,#9484,#9485,#9486,#9487,#9488,#9489,#9490,#9491,
#9492,#9493,#9494,#9495),.UNSPECIFIED.,.F.,.F.,(4,3,3,3,3,3,3,4),(13.8759337553363,
14.796913401075,15.78337429448,16.769835187885,17.75629608129,18.7427569746951,
19.7292178681001,20.1591190625159),.UNSPECIFIED.);
#161=B_SPLINE_CURVE_WITH_KNOTS('',3,(#9496,#9497,#9498,#9499,#9500,#9501,
#9502,#9503,#9504,#9505,#9506,#9507,#9508,#9509,#9510,#9511,#9512,#9513,
#9514,#9515,#9516,#9517),.UNSPECIFIED.,.F.,.F.,(4,3,3,3,3,3,3,4),(-16.4153450200003,
-15.78337429448,-14.796913401075,-13.81045250767,-12.823991614265,-11.83753072086,
-10.851069827455,-10.1321597128207),.UNSPECIFIED.);
#162=B_SPLINE_CURVE_WITH_KNOTS('',3,(#9523,#9524,#9525,#9526,#9527,#9528,
#9529,#9530,#9531,#9532,#9533,#9534,#9535),.UNSPECIFIED.,.F.,.F.,(4,3,3,
3,4),(-3.84897440564114,-2.95938268021501,-1.97292178681,-0.986460893405002,
0.),.UNSPECIFIED.);
#163=B_SPLINE_CURVE_WITH_KNOTS('',3,(#9538,#9539,#9540,#9541,#9542,#9543,
#9544,#9545,#9546,#9547,#9548,#9549,#9550,#9551,#9552,#9553,#9554,#9555,
#9556),.UNSPECIFIED.,.F.,.F.,(4,3,3,3,3,3,4),(2.01694489302845,2.95938268021501,
3.94584357362001,4.93230446702502,5.91876536043002,6.90522625383502,7.59274844815668),
 .UNSPECIFIED.);
#164=B_SPLINE_CURVE_WITH_KNOTS('',3,(#9562,#9563,#9564,#9565),
 .UNSPECIFIED.,.F.,.F.,(4,4),(51.5750455984138,52.2824273504652),
 .UNSPECIFIED.);
#165=B_SPLINE_CURVE_WITH_KNOTS('',3,(#9568,#9569,#9570,#9571,#9572,#9573,
#9574,#9575,#9576,#9577),.UNSPECIFIED.,.F.,.F.,(4,3,3,4),(-50.2654824574367,
-49.3230446702501,-48.3365837768451,-47.8312715558982),.UNSPECIFIED.);
#166=B_SPLINE_CURVE_WITH_KNOTS('',3,(#9582,#9583,#9584,#9585,#9586,#9587,
#9588,#9589,#9590,#9591,#9592,#9593,#9594,#9595,#9596,#9597,#9598,#9599,
#9600,#9601,#9602,#9603,#9604,#9605,#9606),.UNSPECIFIED.,.F.,.F.,(4,3,3,
3,3,3,3,3,4),(45.2918602912342,45.3772010966301,46.3636619900351,47.3501228834401,
48.3365837768451,49.3230446702501,50.3095055636551,51.2959664570602,51.5750455984138),
 .UNSPECIFIED.);
#167=B_SPLINE_CURVE_WITH_KNOTS('',3,(#9607,#9608,#9609,#9610,#9611,#9612,
#9613,#9614,#9615,#9616,#9617,#9618,#9619,#9620,#9621,#9622,#9623,#9624,
#9625,#9626,#9627,#9628),.UNSPECIFIED.,.F.,.F.,(4,3,3,3,3,3,3,4),(-47.8312715558982,
-47.3501228834401,-46.3636619900351,-45.3772010966301,-44.3907402032251,
-43.4042793098201,-42.4178184164151,-41.5480862487187),.UNSPECIFIED.);
#168=B_SPLINE_CURVE_WITH_KNOTS('',3,(#9633,#9634,#9635,#9636,#9637,#9638,
#9639,#9640,#9641,#9642,#9643,#9644,#9645,#9646,#9647,#9648,#9649,#9650,
#9651,#9652,#9653,#9654),.UNSPECIFIED.,.F.,.F.,(4,3,3,3,3,3,3,4),(39.0086749840546,
39.4584357362001,40.4448966296051,41.4313575230101,42.4178184164151,43.4042793098201,
44.3907402032251,45.2918602912342),.UNSPECIFIED.);
#169=B_SPLINE_CURVE_WITH_KNOTS('',3,(#9655,#9656,#9657,#9658,#9659,#9660,
#9661,#9662,#9663,#9664,#9665,#9666,#9667,#9668,#9669,#9670,#9671,#9672,
#9673,#9674,#9675,#9676,#9677,#9678,#9679),.UNSPECIFIED.,.F.,.F.,(4,3,3,
3,3,3,3,3,4),(-41.5480862487187,-41.4313575230101,-40.4448966296051,-39.4584357362001,
-38.4719748427951,-37.4855139493901,-36.4990530559851,-35.5125921625801,
-35.2649009415391),.UNSPECIFIED.);
#170=B_SPLINE_CURVE_WITH_KNOTS('',3,(#9684,#9685,#9686,#9687,#9688,#9689,
#9690,#9691,#9692,#9693,#9694,#9695,#9696,#9697,#9698,#9699,#9700,#9701,
#9702,#9703,#9704,#9705),.UNSPECIFIED.,.F.,.F.,(4,3,3,3,3,3,3,4),(32.725489676875,
33.5396703757701,34.5261312691751,35.5125921625801,36.4990530559851,37.4855139493901,
38.4719748427951,39.0086749840546),.UNSPECIFIED.);
#171=B_SPLINE_CURVE_WITH_KNOTS('',3,(#9706,#9707,#9708,#9709,#9710,#9711,
#9712,#9713,#9714,#9715,#9716,#9717,#9718,#9719,#9720,#9721,#9722,#9723,
#9724,#9725,#9726,#9727),.UNSPECIFIED.,.F.,.F.,(4,3,3,3,3,3,3,4),(-35.2649009415391,
-34.5261312691751,-33.5396703757701,-32.5532094823651,-31.5667485889601,
-30.5802876955551,-29.5938268021501,-28.9817156343595),.UNSPECIFIED.);
#172=B_SPLINE_CURVE_WITH_KNOTS('',3,(#9732,#9733,#9734,#9735,#9736,#9737,
#9738,#9739,#9740,#9741,#9742,#9743,#9744,#9745,#9746,#9747,#9748,#9749,
#9750,#9751,#9752,#9753,#9754,#9755,#9756),.UNSPECIFIED.,.F.,.F.,(4,3,3,
3,3,3,3,3,4),(26.4423043696954,26.6344441219351,27.6209050153401,28.6073659087451,
29.5938268021501,30.5802876955551,31.5667485889601,32.5532094823651,32.725489676875),
 .UNSPECIFIED.);
#173=B_SPLINE_CURVE_WITH_KNOTS('',3,(#9757,#9758,#9759,#9760,#9761,#9762,
#9763,#9764,#9765,#9766,#9767,#9768,#9769,#9770,#9771,#9772,#9773,#9774,
#9775,#9776,#9777,#9778),.UNSPECIFIED.,.F.,.F.,(4,3,3,3,3,3,3,4),(-28.9817156343595,
-28.6073659087451,-27.6209050153401,-26.6344441219351,-25.6479832285301,
-24.6615223351251,-23.6750614417201,-22.6985303271799),.UNSPECIFIED.);
#174=B_SPLINE_CURVE_WITH_KNOTS('',3,(#9783,#9784,#9785,#9786,#9787,#9788,
#9789,#9790,#9791,#9792,#9793,#9794,#9795,#9796,#9797,#9798,#9799,#9800,
#9801,#9802,#9803,#9804),.UNSPECIFIED.,.F.,.F.,(4,3,3,3,3,3,3,4),(20.1591190625158,
20.7156787615051,21.7021396549101,22.6886005483151,23.6750614417201,24.6615223351251,
25.6479832285301,26.4423043696954),.UNSPECIFIED.);
#175=B_SPLINE_CURVE_WITH_KNOTS('',3,(#9805,#9806,#9807,#9808,#9809,#9810,
#9811,#9812,#9813,#9814,#9815,#9816,#9817,#9818,#9819,#9820,#9821,#9822,
#9823,#9824,#9825,#9826,#9827,#9828,#9829),.UNSPECIFIED.,.F.,.F.,(4,3,3,
3,3,3,3,3,4),(-22.6985303271799,-22.6886005483151,-21.7021396549101,-20.7156787615051,
-19.7292178681001,-18.7427569746951,-17.75629608129,-16.7698351878851,-16.4153450200003),
 .UNSPECIFIED.);
#176=B_SPLINE_CURVE_WITH_KNOTS('',3,(#9834,#9835,#9836,#9837,#9838,#9839,
#9840,#9841,#9842,#9843,#9844,#9845,#9846,#9847,#9848,#9849,#9850,#9851,
#9852,#9853,#9854,#9855),.UNSPECIFIED.,.F.,.F.,(4,3,3,3,3,3,3,4),(13.8759337553363,
14.796913401075,15.78337429448,16.769835187885,17.7562960812901,18.742756974695,
19.7292178681001,20.1591190625158),.UNSPECIFIED.);
#177=B_SPLINE_CURVE_WITH_KNOTS('',3,(#9856,#9857,#9858,#9859,#9860,#9861,
#9862,#9863,#9864,#9865,#9866,#9867,#9868,#9869,#9870,#9871,#9872,#9873,
#9874,#9875,#9876,#9877),.UNSPECIFIED.,.F.,.F.,(4,3,3,3,3,3,3,4),(-16.4153450200003,
-15.78337429448,-14.796913401075,-13.81045250767,-12.823991614265,-11.83753072086,
-10.851069827455,-10.1321597128207),.UNSPECIFIED.);
#178=B_SPLINE_CURVE_WITH_KNOTS('',3,(#9883,#9884,#9885,#9886,#9887,#9888,
#9889,#9890,#9891,#9892,#9893,#9894,#9895),.UNSPECIFIED.,.F.,.F.,(4,3,3,
3,4),(-3.84897440564113,-2.95938268021501,-1.97292178681,-0.986460893405001,
0.),.UNSPECIFIED.);
#179=B_SPLINE_CURVE_WITH_KNOTS('',3,(#9898,#9899,#9900,#9901,#9902,#9903,
#9904,#9905,#9906,#9907,#9908,#9909,#9910,#9911,#9912,#9913,#9914,#9915,
#9916),.UNSPECIFIED.,.F.,.F.,(4,3,3,3,3,3,4),(2.01694489302843,2.95938268021501,
3.94584357362001,4.93230446702501,5.91876536043002,6.90522625383502,7.59274844815667),
 .UNSPECIFIED.);
#180=B_SPLINE_CURVE_WITH_KNOTS('',3,(#9922,#9923,#9924,#9925),
 .UNSPECIFIED.,.F.,.F.,(4,4),(51.5750455984138,52.2824273504651),
 .UNSPECIFIED.);
#181=B_SPLINE_CURVE_WITH_KNOTS('',3,(#9928,#9929,#9930,#9931,#9932,#9933,
#9934,#9935,#9936,#9937),.UNSPECIFIED.,.F.,.F.,(4,3,3,4),(-50.2654824574367,
-49.3230446702501,-48.3365837768451,-47.8312715558982),.UNSPECIFIED.);
#182=B_SPLINE_CURVE_WITH_KNOTS('',3,(#9942,#9943,#9944,#9945,#9946,#9947,
#9948,#9949,#9950,#9951,#9952,#9953,#9954,#9955,#9956,#9957,#9958,#9959,
#9960,#9961,#9962,#9963,#9964,#9965,#9966),.UNSPECIFIED.,.F.,.F.,(4,3,3,
3,3,3,3,3,4),(45.2918602912342,45.3772010966301,46.3636619900351,47.3501228834401,
48.3365837768451,49.3230446702501,50.3095055636552,51.2959664570602,51.5750455984138),
 .UNSPECIFIED.);
#183=B_SPLINE_CURVE_WITH_KNOTS('',3,(#9967,#9968,#9969,#9970,#9971,#9972,
#9973,#9974,#9975,#9976,#9977,#9978,#9979,#9980,#9981,#9982,#9983,#9984,
#9985,#9986,#9987,#9988),.UNSPECIFIED.,.F.,.F.,(4,3,3,3,3,3,3,4),(-47.8312715558982,
-47.3501228834401,-46.3636619900351,-45.3772010966301,-44.3907402032251,
-43.4042793098201,-42.4178184164151,-41.5480862487187),.UNSPECIFIED.);
#184=B_SPLINE_CURVE_WITH_KNOTS('',3,(#9993,#9994,#9995,#9996,#9997,#9998,
#9999,#10000,#10001,#10002,#10003,#10004,#10005,#10006,#10007,#10008,#10009,
#10010,#10011,#10012,#10013,#10014),.UNSPECIFIED.,.F.,.F.,(4,3,3,3,3,3,
3,4),(39.0086749840546,39.4584357362001,40.4448966296051,41.4313575230101,
42.4178184164151,43.4042793098201,44.3907402032251,45.2918602912342),
 .UNSPECIFIED.);
#185=B_SPLINE_CURVE_WITH_KNOTS('',3,(#10015,#10016,#10017,#10018,#10019,
#10020,#10021,#10022,#10023,#10024,#10025,#10026,#10027,#10028,#10029,#10030,
#10031,#10032,#10033,#10034,#10035,#10036,#10037,#10038,#10039),
 .UNSPECIFIED.,.F.,.F.,(4,3,3,3,3,3,3,3,4),(-41.5480862487187,-41.4313575230101,
-40.4448966296051,-39.4584357362001,-38.4719748427951,-37.4855139493901,
-36.4990530559851,-35.5125921625801,-35.2649009415391),.UNSPECIFIED.);
#186=B_SPLINE_CURVE_WITH_KNOTS('',3,(#10044,#10045,#10046,#10047,#10048,
#10049,#10050,#10051,#10052,#10053,#10054,#10055,#10056,#10057,#10058,#10059,
#10060,#10061,#10062,#10063,#10064,#10065),.UNSPECIFIED.,.F.,.F.,(4,3,3,
3,3,3,3,4),(32.725489676875,33.5396703757701,34.5261312691751,35.5125921625801,
36.4990530559851,37.4855139493901,38.4719748427951,39.0086749840546),
 .UNSPECIFIED.);
#187=B_SPLINE_CURVE_WITH_KNOTS('',3,(#10066,#10067,#10068,#10069,#10070,
#10071,#10072,#10073,#10074,#10075,#10076,#10077,#10078,#10079,#10080,#10081,
#10082,#10083,#10084,#10085,#10086,#10087),.UNSPECIFIED.,.F.,.F.,(4,3,3,
3,3,3,3,4),(-35.2649009415391,-34.5261312691751,-33.5396703757701,-32.5532094823651,
-31.5667485889601,-30.5802876955551,-29.5938268021501,-28.9817156343595),
 .UNSPECIFIED.);
#188=B_SPLINE_CURVE_WITH_KNOTS('',3,(#10092,#10093,#10094,#10095,#10096,
#10097,#10098,#10099,#10100,#10101,#10102,#10103,#10104,#10105,#10106,#10107,
#10108,#10109,#10110,#10111,#10112,#10113,#10114,#10115,#10116),
 .UNSPECIFIED.,.F.,.F.,(4,3,3,3,3,3,3,3,4),(26.4423043696954,26.6344441219351,
27.6209050153401,28.6073659087451,29.5938268021501,30.5802876955551,31.5667485889601,
32.5532094823651,32.725489676875),.UNSPECIFIED.);
#189=B_SPLINE_CURVE_WITH_KNOTS('',3,(#10117,#10118,#10119,#10120,#10121,
#10122,#10123,#10124,#10125,#10126,#10127,#10128,#10129,#10130,#10131,#10132,
#10133,#10134,#10135,#10136,#10137,#10138),.UNSPECIFIED.,.F.,.F.,(4,3,3,
3,3,3,3,4),(-28.9817156343595,-28.6073659087451,-27.6209050153401,-26.6344441219351,
-25.6479832285301,-24.6615223351251,-23.6750614417201,-22.6985303271799),
 .UNSPECIFIED.);
#190=B_SPLINE_CURVE_WITH_KNOTS('',3,(#10143,#10144,#10145,#10146,#10147,
#10148,#10149,#10150,#10151,#10152,#10153,#10154,#10155,#10156,#10157,#10158,
#10159,#10160,#10161,#10162,#10163,#10164),.UNSPECIFIED.,.F.,.F.,(4,3,3,
3,3,3,3,4),(20.1591190625158,20.7156787615051,21.7021396549101,22.6886005483151,
23.6750614417201,24.6615223351251,25.6479832285301,26.4423043696954),
 .UNSPECIFIED.);
#191=B_SPLINE_CURVE_WITH_KNOTS('',3,(#10165,#10166,#10167,#10168,#10169,
#10170,#10171,#10172,#10173,#10174,#10175,#10176,#10177,#10178,#10179,#10180,
#10181,#10182,#10183,#10184,#10185,#10186,#10187,#10188,#10189),
 .UNSPECIFIED.,.F.,.F.,(4,3,3,3,3,3,3,3,4),(-22.6985303271799,-22.6886005483151,
-21.7021396549101,-20.7156787615051,-19.7292178681001,-18.7427569746951,
-17.75629608129,-16.769835187885,-16.4153450200003),.UNSPECIFIED.);
#192=B_SPLINE_CURVE_WITH_KNOTS('',3,(#10194,#10195,#10196,#10197,#10198,
#10199,#10200,#10201,#10202,#10203,#10204,#10205,#10206,#10207,#10208,#10209,
#10210,#10211,#10212,#10213,#10214,#10215),.UNSPECIFIED.,.F.,.F.,(4,3,3,
3,3,3,3,4),(13.8759337553363,14.796913401075,15.78337429448,16.769835187885,
17.7562960812901,18.742756974695,19.7292178681001,20.1591190625158),
 .UNSPECIFIED.);
#193=B_SPLINE_CURVE_WITH_KNOTS('',3,(#10216,#10217,#10218,#10219,#10220,
#10221,#10222,#10223,#10224,#10225,#10226,#10227,#10228,#10229,#10230,#10231,
#10232,#10233,#10234,#10235,#10236,#10237),.UNSPECIFIED.,.F.,.F.,(4,3,3,
3,3,3,3,4),(-16.4153450200003,-15.78337429448,-14.796913401075,-13.81045250767,
-12.823991614265,-11.83753072086,-10.851069827455,-10.1321597128207),
 .UNSPECIFIED.);
#194=B_SPLINE_CURVE_WITH_KNOTS('',3,(#10243,#10244,#10245,#10246,#10247,
#10248,#10249,#10250,#10251,#10252,#10253,#10254,#10255),.UNSPECIFIED.,
 .F.,.F.,(4,3,3,3,4),(-3.84897440564114,-2.95938268021501,-1.97292178681001,
-0.986460893405003,0.),.UNSPECIFIED.);
#195=B_SPLINE_CURVE_WITH_KNOTS('',3,(#10258,#10259,#10260,#10261,#10262,
#10263,#10264,#10265,#10266,#10267,#10268,#10269,#10270,#10271,#10272,#10273,
#10274,#10275,#10276),.UNSPECIFIED.,.F.,.F.,(4,3,3,3,3,3,4),(2.01694489302845,
2.95938268021501,3.94584357362001,4.93230446702501,5.91876536043002,6.90522625383502,
7.59274844815667),.UNSPECIFIED.);
#196=B_SPLINE_CURVE_WITH_KNOTS('',3,(#10282,#10283,#10284,#10285),
 .UNSPECIFIED.,.F.,.F.,(4,4),(51.5750455984138,52.2824273504651),
 .UNSPECIFIED.);
#197=B_SPLINE_CURVE_WITH_KNOTS('',3,(#10288,#10289,#10290,#10291,#10292,
#10293,#10294,#10295,#10296,#10297),.UNSPECIFIED.,.F.,.F.,(4,3,3,4),(-50.2654824574367,
-49.3230446702501,-48.3365837768451,-47.8312715558982),.UNSPECIFIED.);
#198=B_SPLINE_CURVE_WITH_KNOTS('',3,(#10302,#10303,#10304,#10305,#10306,
#10307,#10308,#10309,#10310,#10311,#10312,#10313,#10314,#10315,#10316,#10317,
#10318,#10319,#10320,#10321,#10322,#10323,#10324,#10325,#10326),
 .UNSPECIFIED.,.F.,.F.,(4,3,3,3,3,3,3,3,4),(45.2918602912342,45.3772010966301,
46.3636619900351,47.3501228834401,48.3365837768451,49.3230446702501,50.3095055636551,
51.2959664570601,51.5750455984138),.UNSPECIFIED.);
#199=B_SPLINE_CURVE_WITH_KNOTS('',3,(#10327,#10328,#10329,#10330,#10331,
#10332,#10333,#10334,#10335,#10336,#10337,#10338,#10339,#10340,#10341,#10342,
#10343,#10344,#10345,#10346,#10347,#10348),.UNSPECIFIED.,.F.,.F.,(4,3,3,
3,3,3,3,4),(-47.8312715558982,-47.3501228834401,-46.3636619900351,-45.3772010966301,
-44.3907402032251,-43.4042793098201,-42.4178184164151,-41.5480862487187),
 .UNSPECIFIED.);
#200=B_SPLINE_CURVE_WITH_KNOTS('',3,(#10353,#10354,#10355,#10356,#10357,
#10358,#10359,#10360,#10361,#10362,#10363,#10364,#10365,#10366,#10367,#10368,
#10369,#10370,#10371,#10372,#10373,#10374),.UNSPECIFIED.,.F.,.F.,(4,3,3,
3,3,3,3,4),(39.0086749840546,39.4584357362001,40.4448966296051,41.4313575230101,
42.4178184164151,43.4042793098201,44.3907402032251,45.2918602912342),
 .UNSPECIFIED.);
#201=B_SPLINE_CURVE_WITH_KNOTS('',3,(#10375,#10376,#10377,#10378,#10379,
#10380,#10381,#10382,#10383,#10384,#10385,#10386,#10387,#10388,#10389,#10390,
#10391,#10392,#10393,#10394,#10395,#10396,#10397,#10398,#10399),
 .UNSPECIFIED.,.F.,.F.,(4,3,3,3,3,3,3,3,4),(-41.5480862487187,-41.4313575230101,
-40.4448966296051,-39.4584357362001,-38.4719748427951,-37.4855139493901,
-36.4990530559851,-35.5125921625801,-35.2649009415391),.UNSPECIFIED.);
#202=B_SPLINE_CURVE_WITH_KNOTS('',3,(#10404,#10405,#10406,#10407,#10408,
#10409,#10410,#10411,#10412,#10413,#10414,#10415,#10416,#10417,#10418,#10419,
#10420,#10421,#10422,#10423,#10424,#10425),.UNSPECIFIED.,.F.,.F.,(4,3,3,
3,3,3,3,4),(32.725489676875,33.5396703757701,34.5261312691751,35.5125921625801,
36.4990530559851,37.4855139493901,38.4719748427951,39.0086749840546),
 .UNSPECIFIED.);
#203=B_SPLINE_CURVE_WITH_KNOTS('',3,(#10426,#10427,#10428,#10429,#10430,
#10431,#10432,#10433,#10434,#10435,#10436,#10437,#10438,#10439,#10440,#10441,
#10442,#10443,#10444,#10445,#10446,#10447),.UNSPECIFIED.,.F.,.F.,(4,3,3,
3,3,3,3,4),(-35.2649009415391,-34.5261312691751,-33.5396703757701,-32.5532094823651,
-31.5667485889601,-30.5802876955551,-29.5938268021501,-28.9817156343595),
 .UNSPECIFIED.);
#204=B_SPLINE_CURVE_WITH_KNOTS('',3,(#10452,#10453,#10454,#10455,#10456,
#10457,#10458,#10459,#10460,#10461,#10462,#10463,#10464,#10465,#10466,#10467,
#10468,#10469,#10470,#10471,#10472,#10473,#10474,#10475,#10476),
 .UNSPECIFIED.,.F.,.F.,(4,3,3,3,3,3,3,3,4),(26.4423043696954,26.6344441219351,
27.6209050153401,28.6073659087451,29.5938268021501,30.5802876955551,31.5667485889601,
32.5532094823651,32.725489676875),.UNSPECIFIED.);
#205=B_SPLINE_CURVE_WITH_KNOTS('',3,(#10477,#10478,#10479,#10480,#10481,
#10482,#10483,#10484,#10485,#10486,#10487,#10488,#10489,#10490,#10491,#10492,
#10493,#10494,#10495,#10496,#10497,#10498),.UNSPECIFIED.,.F.,.F.,(4,3,3,
3,3,3,3,4),(-28.9817156343595,-28.6073659087451,-27.6209050153401,-26.6344441219351,
-25.6479832285301,-24.6615223351251,-23.6750614417201,-22.6985303271799),
 .UNSPECIFIED.);
#206=B_SPLINE_CURVE_WITH_KNOTS('',3,(#10503,#10504,#10505,#10506,#10507,
#10508,#10509,#10510,#10511,#10512,#10513,#10514,#10515,#10516,#10517,#10518,
#10519,#10520,#10521,#10522,#10523,#10524),.UNSPECIFIED.,.F.,.F.,(4,3,3,
3,3,3,3,4),(20.1591190625158,20.7156787615051,21.7021396549101,22.6886005483151,
23.6750614417201,24.6615223351251,25.6479832285301,26.4423043696954),
 .UNSPECIFIED.);
#207=B_SPLINE_CURVE_WITH_KNOTS('',3,(#10525,#10526,#10527,#10528,#10529,
#10530,#10531,#10532,#10533,#10534,#10535,#10536,#10537,#10538,#10539,#10540,
#10541,#10542,#10543,#10544,#10545,#10546,#10547,#10548,#10549),
 .UNSPECIFIED.,.F.,.F.,(4,3,3,3,3,3,3,3,4),(-22.6985303271799,-22.6886005483151,
-21.7021396549101,-20.7156787615051,-19.7292178681001,-18.7427569746951,
-17.75629608129,-16.769835187885,-16.4153450200003),.UNSPECIFIED.);
#208=B_SPLINE_CURVE_WITH_KNOTS('',3,(#10554,#10555,#10556,#10557,#10558,
#10559,#10560,#10561,#10562,#10563,#10564,#10565,#10566,#10567,#10568,#10569,
#10570,#10571,#10572,#10573,#10574,#10575),.UNSPECIFIED.,.F.,.F.,(4,3,3,
3,3,3,3,4),(13.8759337553363,14.796913401075,15.78337429448,16.769835187885,
17.7562960812901,18.742756974695,19.7292178681001,20.1591190625158),
 .UNSPECIFIED.);
#209=B_SPLINE_CURVE_WITH_KNOTS('',3,(#10576,#10577,#10578,#10579,#10580,
#10581,#10582,#10583,#10584,#10585,#10586,#10587,#10588,#10589,#10590,#10591,
#10592,#10593,#10594,#10595,#10596,#10597),.UNSPECIFIED.,.F.,.F.,(4,3,3,
3,3,3,3,4),(-16.4153450200003,-15.78337429448,-14.796913401075,-13.81045250767,
-12.823991614265,-11.83753072086,-10.851069827455,-10.1321597128207),
 .UNSPECIFIED.);
#210=B_SPLINE_CURVE_WITH_KNOTS('',3,(#10603,#10604,#10605,#10606,#10607,
#10608,#10609,#10610,#10611,#10612,#10613,#10614,#10615),.UNSPECIFIED.,
 .F.,.F.,(4,3,3,3,4),(-3.84897440564114,-2.95938268021501,-1.97292178681001,
-0.986460893405003,0.),.UNSPECIFIED.);
#211=B_SPLINE_CURVE_WITH_KNOTS('',3,(#10618,#10619,#10620,#10621,#10622,
#10623,#10624,#10625,#10626,#10627,#10628,#10629,#10630,#10631,#10632,#10633,
#10634,#10635,#10636),.UNSPECIFIED.,.F.,.F.,(4,3,3,3,3,3,4),(2.01694489302845,
2.95938268021501,3.94584357362001,4.93230446702501,5.91876536043002,6.90522625383502,
7.59274844815667),.UNSPECIFIED.);
#212=B_SPLINE_CURVE_WITH_KNOTS('',3,(#10642,#10643,#10644,#10645,#10646,
#10647,#10648,#10649),.UNSPECIFIED.,.F.,.F.,(4,1,1,1,1,4),(59.6902604182061,
60.195572639153,61.182033532558,62.168494425963,63.154955319368,64.141416212773),
 .UNSPECIFIED.);
#213=B_SPLINE_CURVE_WITH_KNOTS('',3,(#10652,#10653,#10654,#10655,#10656,
#10657,#10658,#10659,#10660),.UNSPECIFIED.,.F.,.F.,(4,1,1,1,1,1,4),(59.6902604182061,
59.775601223602,60.762062117007,61.748523010412,62.734983903817,63.721444797222,
64.6638825844085),.UNSPECIFIED.);
#214=B_SPLINE_CURVE_WITH_KNOTS('',3,(#10665,#10666,#10667,#10668,#10669,
#10670,#10671,#10672,#10673,#10674),.UNSPECIFIED.,.F.,.F.,(4,1,1,1,1,1,
1,4),(53.4070751110265,54.2768072787229,55.2632681721279,56.2497290655329,
57.2361899589379,58.222650852343,59.209111745748,59.6902604182061),
 .UNSPECIFIED.);
#215=B_SPLINE_CURVE_WITH_KNOTS('',3,(#10675,#10676,#10677,#10678,#10679,
#10680,#10681,#10682,#10683,#10684),.UNSPECIFIED.,.F.,.F.,(4,1,1,1,1,1,
1,4),(53.4070751110265,53.856835863172,54.843296756577,55.829757649982,
56.816218543387,57.802679436792,58.789140330197,59.6902604182061),
 .UNSPECIFIED.);
#216=B_SPLINE_CURVE_WITH_KNOTS('',3,(#10689,#10690,#10691,#10692,#10693,
#10694,#10695,#10696,#10697,#10698,#10699),.UNSPECIFIED.,.F.,.F.,(4,1,1,
1,1,1,1,1,4),(47.1238898038469,47.3715810248879,48.3580419182929,49.3445028116979,
50.3309637051029,51.3174245985079,52.3038854919129,53.2903463853179,53.4070751110265),
 .UNSPECIFIED.);
#217=B_SPLINE_CURVE_WITH_KNOTS('',3,(#10700,#10701,#10702,#10703,#10704,
#10705,#10706,#10707,#10708,#10709),.UNSPECIFIED.,.F.,.F.,(4,1,1,1,1,1,
1,4),(47.1238898038469,47.9380705027419,48.9245313961469,49.9109922895519,
50.8974531829569,51.8839140763619,52.8703749697669,53.4070751110265),
 .UNSPECIFIED.);
#218=B_SPLINE_CURVE_WITH_KNOTS('',3,(#10714,#10715,#10716,#10717,#10718,
#10719,#10720,#10721,#10722,#10723),.UNSPECIFIED.,.F.,.F.,(4,1,1,1,1,1,
1,4),(40.8407044966673,41.4528156644579,42.4392765578629,43.4257374512679,
44.4121983446729,45.3986592380779,46.3851201314829,47.1238898038469),
 .UNSPECIFIED.);
#219=B_SPLINE_CURVE_WITH_KNOTS('',3,(#10724,#10725,#10726,#10727,#10728,
#10729,#10730,#10731,#10732,#10733,#10734),.UNSPECIFIED.,.F.,.F.,(4,1,1,
1,1,1,1,1,4),(40.8407044966673,41.0328442489069,42.0193051423119,43.0057660357169,
43.9922269291219,44.9786878225269,45.9651487159319,46.9516096093369,47.1238898038469),
 .UNSPECIFIED.);
#220=B_SPLINE_CURVE_WITH_KNOTS('',3,(#10739,#10740,#10741,#10742,#10743,
#10744,#10745,#10746,#10747,#10748),.UNSPECIFIED.,.F.,.F.,(4,1,1,1,1,1,
1,4),(34.5575191894877,35.5340503040279,36.5205111974329,37.5069720908379,
38.4934329842429,39.4798938776479,40.4663547710529,40.8407044966673),
 .UNSPECIFIED.);
#221=B_SPLINE_CURVE_WITH_KNOTS('',3,(#10749,#10750,#10751,#10752,#10753,
#10754,#10755,#10756,#10757,#10758),.UNSPECIFIED.,.F.,.F.,(4,1,1,1,1,1,
1,4),(34.5575191894877,35.1140788884769,36.1005397818819,37.0870006752869,
38.0734615686919,39.0599224620969,40.0463833555019,40.8407044966673),
 .UNSPECIFIED.);
#222=B_SPLINE_CURVE_WITH_KNOTS('',3,(#10763,#10764,#10765,#10766,#10767,
#10768,#10769,#10770,#10771,#10772,#10773),.UNSPECIFIED.,.F.,.F.,(4,1,1,
1,1,1,1,1,4),(28.2743338823081,28.6288240501929,29.6152849435979,30.6017458370029,
31.5882067304079,32.5746676238129,33.5611285172179,34.5475894106229,34.5575191894877),
 .UNSPECIFIED.);
#223=B_SPLINE_CURVE_WITH_KNOTS('',3,(#10774,#10775,#10776,#10777,#10778,
#10779,#10780,#10781,#10782,#10783),.UNSPECIFIED.,.F.,.F.,(4,1,1,1,1,1,
1,4),(28.2743338823081,29.1953135280469,30.1817744214519,31.1682353148569,
32.1546962082619,33.1411571016669,34.1276179950719,34.5575191894877),
 .UNSPECIFIED.);
#224=B_SPLINE_CURVE_WITH_KNOTS('',3,(#10788,#10789,#10790,#10791,#10792,
#10793,#10794,#10795,#10796,#10797),.UNSPECIFIED.,.F.,.F.,(4,1,1,1,1,1,
1,4),(21.9911485751285,22.7100586897628,23.6965195831678,24.6829804765729,
25.6694413699779,26.6559022633829,27.6423631567879,28.2743338823081),
 .UNSPECIFIED.);
#225=B_SPLINE_CURVE_WITH_KNOTS('',3,(#10798,#10799,#10800,#10801,#10802,
#10803,#10804,#10805,#10806,#10807,#10808),.UNSPECIFIED.,.F.,.F.,(4,1,1,
1,1,1,1,1,4),(21.9911485751285,22.2900872742119,23.2765481676169,24.2630090610219,
25.2494699544269,26.2359308478319,27.2223917412369,28.2088526346419,28.2743338823081),
 .UNSPECIFIED.);
#226=B_SPLINE_CURVE_WITH_KNOTS('',3,(#10814,#10815,#10816,#10817,#10818),
 .UNSPECIFIED.,.F.,.F.,(4,1,4),(14.3984001269718,15.3848610203768,15.7079632679489),
 .UNSPECIFIED.);
#227=B_SPLINE_CURVE_WITH_KNOTS('',3,(#10821,#10822,#10823,#10824,#10825),
 .UNSPECIFIED.,.F.,.F.,(4,1,4),(13.8759337553363,14.8183715425228,15.7079632679489),
 .UNSPECIFIED.);
#228=B_SPLINE_CURVE_WITH_KNOTS('',3,(#10831,#10832,#10833,#10834,#10835,
#10836,#10837,#10838),.UNSPECIFIED.,.F.,.F.,(4,1,1,1,1,4),(59.6902604182061,
60.1955726391529,61.1820335325579,62.1684944259629,63.154955319368,64.141416212773),
 .UNSPECIFIED.);
#229=B_SPLINE_CURVE_WITH_KNOTS('',3,(#10841,#10842,#10843,#10844,#10845,
#10846,#10847,#10848,#10849),.UNSPECIFIED.,.F.,.F.,(4,1,1,1,1,1,4),(59.6902604182061,
59.775601223602,60.762062117007,61.748523010412,62.734983903817,63.721444797222,
64.6638825844085),.UNSPECIFIED.);
#230=B_SPLINE_CURVE_WITH_KNOTS('',3,(#10854,#10855,#10856,#10857,#10858,
#10859,#10860,#10861,#10862,#10863),.UNSPECIFIED.,.F.,.F.,(4,1,1,1,1,1,
1,4),(53.4070751110265,54.2768072787229,55.2632681721279,56.2497290655329,
57.2361899589379,58.2226508523429,59.2091117457479,59.6902604182061),
 .UNSPECIFIED.);
#231=B_SPLINE_CURVE_WITH_KNOTS('',3,(#10864,#10865,#10866,#10867,#10868,
#10869,#10870,#10871,#10872,#10873),.UNSPECIFIED.,.F.,.F.,(4,1,1,1,1,1,
1,4),(53.4070751110265,53.856835863172,54.843296756577,55.829757649982,
56.816218543387,57.802679436792,58.789140330197,59.6902604182061),
 .UNSPECIFIED.);
#232=B_SPLINE_CURVE_WITH_KNOTS('',3,(#10878,#10879,#10880,#10881,#10882,
#10883,#10884,#10885,#10886,#10887,#10888),.UNSPECIFIED.,.F.,.F.,(4,1,1,
1,1,1,1,1,4),(47.1238898038469,47.3715810248879,48.3580419182929,49.3445028116979,
50.3309637051029,51.3174245985079,52.3038854919129,53.2903463853179,53.4070751110265),
 .UNSPECIFIED.);
#233=B_SPLINE_CURVE_WITH_KNOTS('',3,(#10889,#10890,#10891,#10892,#10893,
#10894,#10895,#10896,#10897,#10898),.UNSPECIFIED.,.F.,.F.,(4,1,1,1,1,1,
1,4),(47.1238898038469,47.9380705027419,48.9245313961469,49.9109922895519,
50.8974531829569,51.8839140763619,52.8703749697669,53.4070751110265),
 .UNSPECIFIED.);
#234=B_SPLINE_CURVE_WITH_KNOTS('',3,(#10903,#10904,#10905,#10906,#10907,
#10908,#10909,#10910,#10911,#10912),.UNSPECIFIED.,.F.,.F.,(4,1,1,1,1,1,
1,4),(40.8407044966673,41.4528156644579,42.4392765578629,43.4257374512679,
44.4121983446729,45.3986592380779,46.3851201314829,47.1238898038469),
 .UNSPECIFIED.);
#235=B_SPLINE_CURVE_WITH_KNOTS('',3,(#10913,#10914,#10915,#10916,#10917,
#10918,#10919,#10920,#10921,#10922,#10923),.UNSPECIFIED.,.F.,.F.,(4,1,1,
1,1,1,1,1,4),(40.8407044966673,41.0328442489069,42.0193051423119,43.0057660357169,
43.9922269291219,44.9786878225269,45.9651487159319,46.9516096093369,47.1238898038469),
 .UNSPECIFIED.);
#236=B_SPLINE_CURVE_WITH_KNOTS('',3,(#10928,#10929,#10930,#10931,#10932,
#10933,#10934,#10935,#10936,#10937),.UNSPECIFIED.,.F.,.F.,(4,1,1,1,1,1,
1,4),(34.5575191894877,35.5340503040279,36.5205111974329,37.5069720908379,
38.4934329842429,39.4798938776479,40.4663547710529,40.8407044966673),
 .UNSPECIFIED.);
#237=B_SPLINE_CURVE_WITH_KNOTS('',3,(#10938,#10939,#10940,#10941,#10942,
#10943,#10944,#10945,#10946,#10947),.UNSPECIFIED.,.F.,.F.,(4,1,1,1,1,1,
1,4),(34.5575191894877,35.1140788884769,36.1005397818819,37.0870006752869,
38.0734615686919,39.0599224620969,40.0463833555019,40.8407044966673),
 .UNSPECIFIED.);
#238=B_SPLINE_CURVE_WITH_KNOTS('',3,(#10952,#10953,#10954,#10955,#10956,
#10957,#10958,#10959,#10960,#10961,#10962),.UNSPECIFIED.,.F.,.F.,(4,1,1,
1,1,1,1,1,4),(28.2743338823081,28.6288240501929,29.6152849435979,30.6017458370029,
31.5882067304079,32.5746676238129,33.5611285172179,34.5475894106229,34.5575191894877),
 .UNSPECIFIED.);
#239=B_SPLINE_CURVE_WITH_KNOTS('',3,(#10963,#10964,#10965,#10966,#10967,
#10968,#10969,#10970,#10971,#10972),.UNSPECIFIED.,.F.,.F.,(4,1,1,1,1,1,
1,4),(28.2743338823081,29.1953135280469,30.1817744214519,31.1682353148569,
32.1546962082619,33.1411571016669,34.1276179950719,34.5575191894877),
 .UNSPECIFIED.);
#240=B_SPLINE_CURVE_WITH_KNOTS('',3,(#10977,#10978,#10979,#10980,#10981,
#10982,#10983,#10984,#10985,#10986),.UNSPECIFIED.,.F.,.F.,(4,1,1,1,1,1,
1,4),(21.9911485751285,22.7100586897628,23.6965195831678,24.6829804765728,
25.6694413699778,26.6559022633828,27.6423631567879,28.2743338823081),
 .UNSPECIFIED.);
#241=B_SPLINE_CURVE_WITH_KNOTS('',3,(#10987,#10988,#10989,#10990,#10991,
#10992,#10993,#10994,#10995,#10996,#10997),.UNSPECIFIED.,.F.,.F.,(4,1,1,
1,1,1,1,1,4),(21.9911485751285,22.2900872742119,23.2765481676169,24.2630090610219,
25.2494699544269,26.2359308478319,27.2223917412369,28.2088526346419,28.2743338823081),
 .UNSPECIFIED.);
#242=B_SPLINE_CURVE_WITH_KNOTS('',3,(#11003,#11004,#11005,#11006,#11007),
 .UNSPECIFIED.,.F.,.F.,(4,1,4),(14.3984001269718,15.3848610203768,15.7079632679489),
 .UNSPECIFIED.);
#243=B_SPLINE_CURVE_WITH_KNOTS('',3,(#11010,#11011,#11012,#11013,#11014),
 .UNSPECIFIED.,.F.,.F.,(4,1,4),(13.8759337553363,14.8183715425228,15.7079632679489),
 .UNSPECIFIED.);
#244=B_SPLINE_CURVE_WITH_KNOTS('',3,(#11020,#11021,#11022,#11023,#11024,
#11025,#11026,#11027),.UNSPECIFIED.,.F.,.F.,(4,1,1,1,1,4),(59.6902604182061,
60.1955726391529,61.1820335325579,62.1684944259629,63.154955319368,64.141416212773),
 .UNSPECIFIED.);
#245=B_SPLINE_CURVE_WITH_KNOTS('',3,(#11030,#11031,#11032,#11033,#11034,
#11035,#11036,#11037,#11038),.UNSPECIFIED.,.F.,.F.,(4,1,1,1,1,1,4),(59.6902604182061,
59.775601223602,60.762062117007,61.748523010412,62.734983903817,63.721444797222,
64.6638825844085),.UNSPECIFIED.);
#246=B_SPLINE_CURVE_WITH_KNOTS('',3,(#11043,#11044,#11045,#11046,#11047,
#11048,#11049,#11050,#11051,#11052),.UNSPECIFIED.,.F.,.F.,(4,1,1,1,1,1,
1,4),(53.4070751110265,54.2768072787229,55.2632681721279,56.2497290655329,
57.2361899589379,58.2226508523429,59.2091117457479,59.6902604182061),
 .UNSPECIFIED.);
#247=B_SPLINE_CURVE_WITH_KNOTS('',3,(#11053,#11054,#11055,#11056,#11057,
#11058,#11059,#11060,#11061,#11062),.UNSPECIFIED.,.F.,.F.,(4,1,1,1,1,1,
1,4),(53.4070751110265,53.8568358631719,54.8432967565769,55.8297576499819,
56.816218543387,57.802679436792,58.789140330197,59.6902604182061),
 .UNSPECIFIED.);
#248=B_SPLINE_CURVE_WITH_KNOTS('',3,(#11067,#11068,#11069,#11070,#11071,
#11072,#11073,#11074,#11075,#11076,#11077),.UNSPECIFIED.,.F.,.F.,(4,1,1,
1,1,1,1,1,4),(47.1238898038469,47.3715810248879,48.3580419182929,49.3445028116979,
50.3309637051029,51.3174245985079,52.3038854919129,53.2903463853179,53.4070751110265),
 .UNSPECIFIED.);
#249=B_SPLINE_CURVE_WITH_KNOTS('',3,(#11078,#11079,#11080,#11081,#11082,
#11083,#11084,#11085,#11086,#11087),.UNSPECIFIED.,.F.,.F.,(4,1,1,1,1,1,
1,4),(47.1238898038469,47.9380705027419,48.9245313961469,49.9109922895519,
50.8974531829569,51.8839140763619,52.8703749697669,53.4070751110265),
 .UNSPECIFIED.);
#250=B_SPLINE_CURVE_WITH_KNOTS('',3,(#11092,#11093,#11094,#11095,#11096,
#11097,#11098,#11099,#11100,#11101),.UNSPECIFIED.,.F.,.F.,(4,1,1,1,1,1,
1,4),(40.8407044966673,41.4528156644579,42.4392765578629,43.4257374512679,
44.4121983446729,45.3986592380779,46.3851201314829,47.1238898038469),
 .UNSPECIFIED.);
#251=B_SPLINE_CURVE_WITH_KNOTS('',3,(#11102,#11103,#11104,#11105,#11106,
#11107,#11108,#11109,#11110,#11111,#11112),.UNSPECIFIED.,.F.,.F.,(4,1,1,
1,1,1,1,1,4),(40.8407044966673,41.0328442489069,42.0193051423119,43.0057660357169,
43.9922269291219,44.9786878225269,45.9651487159319,46.9516096093369,47.1238898038469),
 .UNSPECIFIED.);
#252=B_SPLINE_CURVE_WITH_KNOTS('',3,(#11117,#11118,#11119,#11120,#11121,
#11122,#11123,#11124,#11125,#11126),.UNSPECIFIED.,.F.,.F.,(4,1,1,1,1,1,
1,4),(34.5575191894877,35.5340503040279,36.5205111974329,37.5069720908379,
38.4934329842429,39.4798938776479,40.4663547710529,40.8407044966673),
 .UNSPECIFIED.);
#253=B_SPLINE_CURVE_WITH_KNOTS('',3,(#11127,#11128,#11129,#11130,#11131,
#11132,#11133,#11134,#11135,#11136),.UNSPECIFIED.,.F.,.F.,(4,1,1,1,1,1,
1,4),(34.5575191894877,35.1140788884769,36.1005397818819,37.0870006752869,
38.0734615686919,39.0599224620969,40.0463833555019,40.8407044966673),
 .UNSPECIFIED.);
#254=B_SPLINE_CURVE_WITH_KNOTS('',3,(#11141,#11142,#11143,#11144,#11145,
#11146,#11147,#11148,#11149,#11150,#11151),.UNSPECIFIED.,.F.,.F.,(4,1,1,
1,1,1,1,1,4),(28.2743338823081,28.6288240501929,29.6152849435979,30.6017458370029,
31.5882067304079,32.5746676238129,33.5611285172179,34.5475894106229,34.5575191894877),
 .UNSPECIFIED.);
#255=B_SPLINE_CURVE_WITH_KNOTS('',3,(#11152,#11153,#11154,#11155,#11156,
#11157,#11158,#11159,#11160,#11161),.UNSPECIFIED.,.F.,.F.,(4,1,1,1,1,1,
1,4),(28.2743338823081,29.1953135280469,30.1817744214519,31.1682353148569,
32.1546962082619,33.1411571016669,34.1276179950719,34.5575191894877),
 .UNSPECIFIED.);
#256=B_SPLINE_CURVE_WITH_KNOTS('',3,(#11166,#11167,#11168,#11169,#11170,
#11171,#11172,#11173,#11174,#11175),.UNSPECIFIED.,.F.,.F.,(4,1,1,1,1,1,
1,4),(21.9911485751285,22.7100586897628,23.6965195831678,24.6829804765728,
25.6694413699778,26.6559022633828,27.6423631567879,28.2743338823081),
 .UNSPECIFIED.);
#257=B_SPLINE_CURVE_WITH_KNOTS('',3,(#11176,#11177,#11178,#11179,#11180,
#11181,#11182,#11183,#11184,#11185,#11186),.UNSPECIFIED.,.F.,.F.,(4,1,1,
1,1,1,1,1,4),(21.9911485751285,22.2900872742119,23.2765481676169,24.2630090610219,
25.2494699544269,26.2359308478319,27.2223917412369,28.2088526346419,28.2743338823081),
 .UNSPECIFIED.);
#258=B_SPLINE_CURVE_WITH_KNOTS('',3,(#11192,#11193,#11194,#11195,#11196),
 .UNSPECIFIED.,.F.,.F.,(4,1,4),(14.3984001269718,15.3848610203768,15.7079632679489),
 .UNSPECIFIED.);
#259=B_SPLINE_CURVE_WITH_KNOTS('',3,(#11199,#11200,#11201,#11202,#11203),
 .UNSPECIFIED.,.F.,.F.,(4,1,4),(13.8759337553363,14.8183715425228,15.7079632679489),
 .UNSPECIFIED.);
#260=B_SPLINE_CURVE_WITH_KNOTS('',3,(#11209,#11210,#11211,#11212,#11213,
#11214,#11215,#11216),.UNSPECIFIED.,.F.,.F.,(4,1,1,1,1,4),(59.6902604182061,
60.195572639153,61.182033532558,62.168494425963,63.154955319368,64.141416212773),
 .UNSPECIFIED.);
#261=B_SPLINE_CURVE_WITH_KNOTS('',3,(#11219,#11220,#11221,#11222,#11223,
#11224,#11225,#11226,#11227),.UNSPECIFIED.,.F.,.F.,(4,1,1,1,1,1,4),(59.6902604182061,
59.775601223602,60.762062117007,61.748523010412,62.734983903817,63.721444797222,
64.6638825844085),.UNSPECIFIED.);
#262=B_SPLINE_CURVE_WITH_KNOTS('',3,(#11232,#11233,#11234,#11235,#11236,
#11237,#11238,#11239,#11240,#11241),.UNSPECIFIED.,.F.,.F.,(4,1,1,1,1,1,
1,4),(53.4070751110265,54.2768072787229,55.2632681721279,56.2497290655329,
57.2361899589379,58.222650852343,59.209111745748,59.6902604182061),
 .UNSPECIFIED.);
#263=B_SPLINE_CURVE_WITH_KNOTS('',3,(#11242,#11243,#11244,#11245,#11246,
#11247,#11248,#11249,#11250,#11251),.UNSPECIFIED.,.F.,.F.,(4,1,1,1,1,1,
1,4),(53.4070751110265,53.856835863172,54.843296756577,55.829757649982,
56.816218543387,57.802679436792,58.789140330197,59.6902604182061),
 .UNSPECIFIED.);
#264=B_SPLINE_CURVE_WITH_KNOTS('',3,(#11256,#11257,#11258,#11259,#11260,
#11261,#11262,#11263,#11264,#11265,#11266),.UNSPECIFIED.,.F.,.F.,(4,1,1,
1,1,1,1,1,4),(47.1238898038469,47.3715810248879,48.3580419182929,49.3445028116979,
50.3309637051029,51.3174245985079,52.3038854919129,53.2903463853179,53.4070751110265),
 .UNSPECIFIED.);
#265=B_SPLINE_CURVE_WITH_KNOTS('',3,(#11267,#11268,#11269,#11270,#11271,
#11272,#11273,#11274,#11275,#11276),.UNSPECIFIED.,.F.,.F.,(4,1,1,1,1,1,
1,4),(47.1238898038469,47.9380705027419,48.9245313961469,49.9109922895519,
50.8974531829569,51.8839140763619,52.8703749697669,53.4070751110265),
 .UNSPECIFIED.);
#266=B_SPLINE_CURVE_WITH_KNOTS('',3,(#11281,#11282,#11283,#11284,#11285,
#11286,#11287,#11288,#11289,#11290),.UNSPECIFIED.,.F.,.F.,(4,1,1,1,1,1,
1,4),(40.8407044966673,41.4528156644579,42.4392765578629,43.4257374512679,
44.4121983446729,45.3986592380779,46.3851201314829,47.1238898038469),
 .UNSPECIFIED.);
#267=B_SPLINE_CURVE_WITH_KNOTS('',3,(#11291,#11292,#11293,#11294,#11295,
#11296,#11297,#11298,#11299,#11300,#11301),.UNSPECIFIED.,.F.,.F.,(4,1,1,
1,1,1,1,1,4),(40.8407044966673,41.0328442489069,42.0193051423119,43.0057660357169,
43.9922269291219,44.9786878225269,45.9651487159319,46.9516096093369,47.1238898038469),
 .UNSPECIFIED.);
#268=B_SPLINE_CURVE_WITH_KNOTS('',3,(#11306,#11307,#11308,#11309,#11310,
#11311,#11312,#11313,#11314,#11315),.UNSPECIFIED.,.F.,.F.,(4,1,1,1,1,1,
1,4),(34.5575191894877,35.5340503040279,36.5205111974329,37.5069720908379,
38.4934329842429,39.4798938776479,40.4663547710529,40.8407044966673),
 .UNSPECIFIED.);
#269=B_SPLINE_CURVE_WITH_KNOTS('',3,(#11316,#11317,#11318,#11319,#11320,
#11321,#11322,#11323,#11324,#11325),.UNSPECIFIED.,.F.,.F.,(4,1,1,1,1,1,
1,4),(34.5575191894877,35.1140788884769,36.1005397818819,37.0870006752869,
38.0734615686919,39.0599224620969,40.0463833555019,40.8407044966673),
 .UNSPECIFIED.);
#270=B_SPLINE_CURVE_WITH_KNOTS('',3,(#11330,#11331,#11332,#11333,#11334,
#11335,#11336,#11337,#11338,#11339,#11340),.UNSPECIFIED.,.F.,.F.,(4,1,1,
1,1,1,1,1,4),(28.2743338823081,28.6288240501929,29.6152849435979,30.6017458370029,
31.5882067304079,32.5746676238129,33.5611285172179,34.5475894106229,34.5575191894877),
 .UNSPECIFIED.);
#271=B_SPLINE_CURVE_WITH_KNOTS('',3,(#11341,#11342,#11343,#11344,#11345,
#11346,#11347,#11348,#11349,#11350),.UNSPECIFIED.,.F.,.F.,(4,1,1,1,1,1,
1,4),(28.2743338823081,29.1953135280469,30.1817744214519,31.1682353148569,
32.1546962082619,33.1411571016669,34.1276179950719,34.5575191894877),
 .UNSPECIFIED.);
#272=B_SPLINE_CURVE_WITH_KNOTS('',3,(#11355,#11356,#11357,#11358,#11359,
#11360,#11361,#11362,#11363,#11364),.UNSPECIFIED.,.F.,.F.,(4,1,1,1,1,1,
1,4),(21.9911485751285,22.7100586897628,23.6965195831678,24.6829804765729,
25.6694413699779,26.6559022633829,27.6423631567879,28.2743338823081),
 .UNSPECIFIED.);
#273=B_SPLINE_CURVE_WITH_KNOTS('',3,(#11365,#11366,#11367,#11368,#11369,
#11370,#11371,#11372,#11373,#11374,#11375),.UNSPECIFIED.,.F.,.F.,(4,1,1,
1,1,1,1,1,4),(21.9911485751285,22.2900872742119,23.2765481676169,24.2630090610219,
25.2494699544269,26.2359308478319,27.2223917412369,28.2088526346419,28.2743338823081),
 .UNSPECIFIED.);
#274=B_SPLINE_CURVE_WITH_KNOTS('',3,(#11381,#11382,#11383,#11384,#11385),
 .UNSPECIFIED.,.F.,.F.,(4,1,4),(14.3984001269718,15.3848610203768,15.7079632679489),
 .UNSPECIFIED.);
#275=B_SPLINE_CURVE_WITH_KNOTS('',3,(#11388,#11389,#11390,#11391,#11392),
 .UNSPECIFIED.,.F.,.F.,(4,1,4),(13.8759337553363,14.8183715425228,15.7079632679489),
 .UNSPECIFIED.);
#276=B_SPLINE_CURVE_WITH_KNOTS('',3,(#11436,#11437,#11438,#11439,#11440,
#11441,#11442,#11443,#11444,#11445,#11446),.UNSPECIFIED.,.F.,.F.,(4,1,1,
1,1,1,1,1,4),(15.7079632679489,15.8048324359278,16.7912933293328,17.7777542227378,
18.7642151161428,19.7506760095478,20.7371369029528,21.7235977963578,21.9911485751285),
 .UNSPECIFIED.);
#277=B_SPLINE_CURVE_WITH_KNOTS('',3,(#11447,#11448,#11449,#11450,#11451,
#11452,#11453,#11454,#11455,#11456),.UNSPECIFIED.,.F.,.F.,(4,1,1,1,1,1,
1,4),(15.7079632679489,16.3713219137818,17.3577828071869,18.3442437005919,
19.3307045939969,20.3171654874019,21.3036263808069,21.9911485751285),
 .UNSPECIFIED.);
#278=B_SPLINE_CURVE_WITH_KNOTS('',3,(#11681,#11682,#11683,#11684,#11685,
#11686,#11687,#11688,#11689,#11690,#11691,#11692,#11693,#11694,#11695,#11696,
#11697,#11698,#11699,#11700,#11701,#11702,#11703,#11704,#11705,#11706,#11707,
#11708,#11709,#11710,#11711,#11712,#11713,#11714,#11715,#11716,#11717,#11718,
#11719,#11720,#11721,#11722,#11723,#11724,#11725,#11726,#11727,#11728,#11729,
#11730,#11731,#11732,#11733,#11734,#11735,#11736,#11737,#11738),
 .UNSPECIFIED.,.F.,.F.,(4,3,3,3,3,3,3,3,3,3,3,3,3,3,3,3,3,3,3,4),(0.,0.0537021066009618,
0.0886282712367795,0.116609657471856,0.130919531620276,0.183454585359957,
0.216479690566366,0.230600805996023,0.244062534102707,0.292277144780104,
0.326690169730343,0.340044241140144,0.353800608199824,0.404857015795524,
0.431543783542484,0.447172905557772,0.495211581766649,0.520020647218237,
0.558026238582625,0.569248610399476),.UNSPECIFIED.);
#279=B_SPLINE_CURVE_WITH_KNOTS('',3,(#11739,#11740,#11741,#11742,#11743,
#11744,#11745,#11746,#11747,#11748,#11749,#11750,#11751,#11752,#11753,#11754,
#11755,#11756,#11757,#11758,#11759,#11760,#11761,#11762,#11763,#11764,#11765,
#11766,#11767,#11768,#11769,#11770,#11771,#11772,#11773,#11774,#11775,#11776,
#11777,#11778,#11779,#11780,#11781,#11782,#11783,#11784,#11785,#11786,#11787,
#11788,#11789,#11790,#11791,#11792,#11793,#11794,#11795,#11796),
 .UNSPECIFIED.,.F.,.F.,(4,3,3,3,3,3,3,3,3,3,3,3,3,3,3,3,3,3,3,4),(0.,0.0459570110526893,
0.0870590917386331,0.100825848951598,0.150050223978594,0.184086031790598,
0.203261017512761,0.21625650674859,0.263711469126828,0.302873338429799,
0.321032900850433,0.372046336254313,0.401845514967729,0.421231290172383,
0.435656368584207,0.474812416163248,0.492789265029642,0.5115498830849,0.553331205445793,
0.566847306048074),.UNSPECIFIED.);
#280=B_SPLINE_CURVE_WITH_KNOTS('',3,(#11797,#11798,#11799,#11800,#11801,
#11802,#11803,#11804,#11805,#11806,#11807,#11808,#11809,#11810,#11811,#11812,
#11813,#11814,#11815,#11816,#11817,#11818,#11819,#11820,#11821),
 .UNSPECIFIED.,.F.,.F.,(4,3,3,3,3,3,3,3,4),(-10.1321597128207,-9.86460893405003,
-8.87814804064502,-7.89168714724002,-6.90522625383502,-5.91876536043002,
-4.93230446702501,-3.94584357362001,-3.84897440564114),.UNSPECIFIED.);
#281=B_SPLINE_CURVE_WITH_KNOTS('',3,(#12046,#12047,#12048,#12049,#12050,
#12051,#12052,#12053,#12054,#12055,#12056,#12057,#12058,#12059,#12060,#12061,
#12062,#12063,#12064,#12065,#12066,#12067,#12068,#12069,#12070,#12071,#12072,
#12073,#12074,#12075,#12076,#12077,#12078,#12079,#12080,#12081,#12082,#12083,
#12084,#12085,#12086,#12087,#12088,#12089,#12090,#12091,#12092,#12093,#12094,
#12095,#12096,#12097,#12098,#12099,#12100,#12101,#12102,#12103),
 .UNSPECIFIED.,.F.,.F.,(4,3,3,3,3,3,3,3,3,3,3,3,3,3,3,3,3,3,3,4),(0.,0.0459569891390547,
0.0870591697117697,0.100825884142283,0.15005024998693,0.18408602471011,
0.203261079338359,0.216256514601739,0.263711469126829,0.302873340900277,
0.321032901451889,0.372046348770768,0.401845543858265,0.421231416110189,
0.435656634965766,0.474812764874804,0.492785320751935,0.511549417457807,
0.553331205445803,0.566847306048085),.UNSPECIFIED.);
#282=B_SPLINE_CURVE_WITH_KNOTS('',3,(#12104,#12105,#12106,#12107,#12108,
#12109,#12110,#12111,#12112,#12113,#12114,#12115,#12116,#12117,#12118,#12119,
#12120,#12121,#12122,#12123,#12124,#12125,#12126,#12127,#12128),
 .UNSPECIFIED.,.F.,.F.,(4,3,3,3,3,3,3,3,4),(7.59274844815668,7.89168714724002,
8.87814804064503,9.86460893405003,10.851069827455,11.83753072086,12.823991614265,
13.81045250767,13.8759337553363),.UNSPECIFIED.);
#283=B_SPLINE_CURVE_WITH_KNOTS('',3,(#12129,#12130,#12131,#12132,#12133,
#12134,#12135,#12136,#12137,#12138,#12139,#12140,#12141,#12142,#12143,#12144,
#12145,#12146,#12147,#12148,#12149,#12150,#12151,#12152,#12153,#12154,#12155,
#12156,#12157,#12158,#12159,#12160,#12161,#12162,#12163,#12164,#12165,#12166,
#12167,#12168,#12169,#12170,#12171,#12172,#12173,#12174,#12175,#12176,#12177,
#12178,#12179,#12180,#12181,#12182,#12183,#12184,#12185,#12186),
 .UNSPECIFIED.,.F.,.F.,(4,3,3,3,3,3,3,3,3,3,3,3,3,3,3,3,3,3,3,4),(0.,0.0537020933595249,
0.0886282312348469,0.116609505884768,0.130919504019768,0.183454564110696,
0.216479685514756,0.230600804284864,0.244062532276618,0.292277144780091,
0.326690174005652,0.34004425312577,0.353800612122922,0.404857018737847,
0.43154388809724,0.447172964606455,0.495211643185621,0.520020637237826,
0.558026238582621,0.569248610399474),.UNSPECIFIED.);
#284=B_SPLINE_CURVE_WITH_KNOTS('',3,(#12192,#12193,#12194,#12195,#12196,
#12197,#12198,#12199,#12200,#12201,#12202,#12203,#12204,#12205,#12206,#12207,
#12208,#12209,#12210,#12211,#12212,#12213,#12214,#12215,#12216,#12217,#12218,
#12219,#12220,#12221,#12222,#12223,#12224,#12225,#12226,#12227,#12228,#12229,
#12230,#12231,#12232,#12233,#12234,#12235,#12236,#12237,#12238,#12239,#12240,
#12241,#12242,#12243,#12244,#12245,#12246,#12247,#12248,#12249),
 .UNSPECIFIED.,.F.,.F.,(4,3,3,3,3,3,3,3,3,3,3,3,3,3,3,3,3,3,3,4),(0.,0.0459569597282421,
0.0870592743507417,0.100825931397392,0.150050284916509,0.184086015212499,
0.203261162306881,0.216256525140977,0.26371146912684,0.302873344212067,
0.321032902271426,0.372046365582263,0.401845582658033,0.421231585204367,
0.435656992651154,0.474813233102554,0.492780040699884,0.511548795880393,
0.553331205445832,0.566847306048113),.UNSPECIFIED.);
#285=B_SPLINE_CURVE_WITH_KNOTS('',3,(#12250,#12251,#12252,#12253,#12254,
#12255,#12256,#12257,#12258,#12259,#12260,#12261,#12262,#12263,#12264,#12265,
#12266,#12267,#12268,#12269,#12270,#12271,#12272,#12273,#12274,#12275,#12276,
#12277,#12278,#12279,#12280,#12281,#12282,#12283,#12284,#12285,#12286,#12287,
#12288,#12289,#12290,#12291,#12292,#12293,#12294,#12295,#12296,#12297,#12298,
#12299,#12300,#12301,#12302,#12303,#12304,#12305,#12306,#12307),
 .UNSPECIFIED.,.F.,.F.,(4,3,3,3,3,3,3,3,3,3,3,3,3,3,3,3,3,3,3,4),(0.,0.0537021278608587,
0.0886283354605565,0.116609900845683,0.130919575937586,0.183454619477383,
0.216479698675332,0.230600808889542,0.244062537057827,0.29227714478008,
0.326690162862484,0.340044221965521,0.353800601915901,0.404857011082572,
0.431543615670486,0.447172810805832,0.495211483201289,0.520020663253885,
0.558026238582585,0.569248610399439),.UNSPECIFIED.);
#286=B_SPLINE_CURVE_WITH_KNOTS('',3,(#12308,#12309,#12310,#12311,#12312,
#12313,#12314,#12315,#12316,#12317,#12318,#12319,#12320,#12321,#12322,#12323,
#12324,#12325,#12326,#12327,#12328,#12329,#12330,#12331,#12332,#12333,#12334,
#12335,#12336,#12337,#12338,#12339,#12340,#12341,#12342,#12343,#12344,#12345,
#12346,#12347,#12348,#12349,#12350,#12351,#12352,#12353,#12354,#12355,#12356,
#12357,#12358,#12359,#12360,#12361,#12362,#12363,#12364,#12365),
 .UNSPECIFIED.,.F.,.F.,(4,3,3,3,3,3,3,3,3,3,3,3,3,3,3,3,3,3,3,4),(0.,0.0459570233578969,
0.0870590479590349,0.100825829183884,0.150050209366866,0.184086035766608,
0.203260982741087,0.216256502330382,0.263711469126837,0.302873337041598,
0.321032900518168,0.372046329231869,0.40184549875999,0.421231219525568,
0.435656219182855,0.474812220578677,0.49279148193987,0.511550145279393,
0.553331205445819,0.566847306048101),.UNSPECIFIED.);
#287=B_SPLINE_CURVE_WITH_KNOTS('',3,(#12366,#12367,#12368,#12369,#12370,
#12371,#12372,#12373,#12374,#12375,#12376,#12377,#12378,#12379,#12380,#12381,
#12382,#12383,#12384,#12385,#12386,#12387,#12388,#12389,#12390,#12391,#12392,
#12393,#12394,#12395,#12396,#12397,#12398,#12399,#12400,#12401,#12402,#12403,
#12404,#12405,#12406,#12407,#12408,#12409,#12410,#12411,#12412,#12413,#12414,
#12415,#12416,#12417,#12418,#12419,#12420,#12421,#12422,#12423),
 .UNSPECIFIED.,.F.,.F.,(4,3,3,3,3,3,3,3,3,3,3,3,3,3,3,3,3,3,3,4),(0.,0.0537021066010595,
0.0886282712341201,0.116609657460836,0.130919531618635,0.18345458535817,
0.2164796905666,0.230600806130634,0.244062534124687,0.292277144780059,0.32669016973023,
0.340044241170799,0.35380060820706,0.40485701580094,0.431543783567626,0.447172905584617,
0.495211581792678,0.520020647237742,0.558026238582582,0.569248610399435),
 .UNSPECIFIED.);
#288=B_SPLINE_CURVE_WITH_KNOTS('',3,(#12424,#12425,#12426,#12427,#12428,
#12429,#12430,#12431,#12432,#12433,#12434,#12435,#12436,#12437,#12438,#12439,
#12440,#12441,#12442,#12443,#12444,#12445,#12446,#12447,#12448,#12449,#12450,
#12451,#12452,#12453,#12454,#12455,#12456,#12457,#12458,#12459,#12460,#12461,
#12462,#12463,#12464,#12465,#12466,#12467,#12468,#12469,#12470,#12471,#12472,
#12473,#12474,#12475,#12476,#12477,#12478,#12479,#12480,#12481),
 .UNSPECIFIED.,.F.,.F.,(4,3,3,3,3,3,3,3,3,3,3,3,3,3,3,3,3,3,3,4),(0.,0.0459569597282773,
0.0870592743559632,0.100825931391171,0.150050284910477,0.184086015212479,
0.203261162453712,0.216256525163335,0.263711469126836,0.302873344213503,
0.321032902268873,0.372046365578727,0.401845582651689,0.42123158516634,
0.435656992617324,0.474813233058503,0.492780041036963,0.511548795921555,
0.553331205445815,0.566847306048093),.UNSPECIFIED.);
#289=B_SPLINE_CURVE_WITH_KNOTS('',3,(#12482,#12483,#12484,#12485,#12486,
#12487,#12488,#12489,#12490,#12491,#12492,#12493,#12494,#12495,#12496,#12497,
#12498,#12499,#12500,#12501,#12502,#12503,#12504,#12505,#12506,#12507,#12508,
#12509,#12510,#12511,#12512,#12513,#12514,#12515,#12516,#12517,#12518,#12519,
#12520,#12521,#12522,#12523,#12524,#12525,#12526,#12527,#12528,#12529,#12530,
#12531,#12532,#12533,#12534,#12535,#12536,#12537,#12538,#12539),
 .UNSPECIFIED.,.F.,.F.,(4,3,3,3,3,3,3,3,3,3,3,3,3,3,3,3,3,3,3,4),(0.,0.0537021520206258,
0.0886284084442469,0.11661017742178,0.130919626307606,0.183454658252522,
0.216479707884859,0.230600812010997,0.244062540387362,0.292277144780059,
0.326690155053379,0.340044200114974,0.353800594757874,0.404857005714051,
0.43154342480673,0.447172703114038,0.495211371169167,0.520020681489528,
0.558026238582582,0.569248610399435),.UNSPECIFIED.);
#290=B_SPLINE_CURVE_WITH_KNOTS('',3,(#12541,#12542,#12543,#12544,#12545,
#12546,#12547,#12548,#12549,#12550,#12551),.UNSPECIFIED.,.F.,.F.,(4,1,1,
1,1,1,1,1,4),(15.7079632679489,15.8048324359278,16.7912933293328,17.7777542227378,
18.7642151161428,19.7506760095478,20.7371369029528,21.7235977963578,21.9911485751285),
 .UNSPECIFIED.);
#291=B_SPLINE_CURVE_WITH_KNOTS('',3,(#12552,#12553,#12554,#12555,#12556,
#12557,#12558,#12559,#12560,#12561),.UNSPECIFIED.,.F.,.F.,(4,1,1,1,1,1,
1,4),(15.7079632679489,16.3713219137818,17.3577828071869,18.3442437005919,
19.3307045939969,20.3171654874019,21.3036263808069,21.9911485751285),
 .UNSPECIFIED.);
#292=B_SPLINE_CURVE_WITH_KNOTS('',3,(#12786,#12787,#12788,#12789,#12790,
#12791,#12792,#12793,#12794,#12795,#12796,#12797,#12798,#12799,#12800,#12801,
#12802,#12803,#12804,#12805,#12806,#12807,#12808,#12809,#12810,#12811,#12812,
#12813,#12814,#12815,#12816,#12817,#12818,#12819,#12820,#12821,#12822,#12823,
#12824,#12825,#12826,#12827,#12828,#12829,#12830,#12831,#12832,#12833,#12834,
#12835,#12836,#12837,#12838,#12839,#12840,#12841,#12842,#12843),
 .UNSPECIFIED.,.F.,.F.,(4,3,3,3,3,3,3,3,3,3,3,3,3,3,3,3,3,3,3,4),(0.,0.0459570862230108,
0.087058824279425,0.100825728205661,0.150050134723767,0.184086056072108,
0.203260805225187,0.216256479777388,0.263711469126848,0.302873329947912,
0.321032898752379,0.372046293267176,0.401845415752178,0.421230857758822,
0.435655454101214,0.474811219031992,0.492802884326938,0.511551499405496,
0.553331205445843,0.566847306048125),.UNSPECIFIED.);
#293=B_SPLINE_CURVE_WITH_KNOTS('',3,(#12844,#12845,#12846,#12847,#12848,
#12849,#12850,#12851,#12852,#12853,#12854,#12855,#12856,#12857,#12858,#12859,
#12860,#12861,#12862,#12863,#12864,#12865,#12866,#12867,#12868),
 .UNSPECIFIED.,.F.,.F.,(4,3,3,3,3,3,3,3,4),(-10.1321597128207,-9.86460893405003,
-8.87814804064502,-7.89168714724002,-6.90522625383502,-5.91876536043002,
-4.93230446702501,-3.94584357362001,-3.84897440564114),.UNSPECIFIED.);
#294=B_SPLINE_CURVE_WITH_KNOTS('',3,(#13093,#13094,#13095,#13096,#13097,
#13098,#13099,#13100,#13101,#13102,#13103,#13104,#13105,#13106,#13107,#13108,
#13109,#13110,#13111,#13112,#13113,#13114,#13115,#13116,#13117),
 .UNSPECIFIED.,.F.,.F.,(4,3,3,3,3,3,3,3,4),(7.59274844815667,7.89168714724002,
8.87814804064503,9.86460893405003,10.851069827455,11.83753072086,12.823991614265,
13.81045250767,13.8759337553363),.UNSPECIFIED.);
#295=B_SPLINE_CURVE_WITH_KNOTS('',3,(#13118,#13119,#13120,#13121,#13122,
#13123,#13124,#13125,#13126,#13127,#13128,#13129,#13130,#13131,#13132,#13133,
#13134,#13135,#13136,#13137,#13138,#13139,#13140,#13141,#13142,#13143,#13144,
#13145,#13146,#13147,#13148,#13149,#13150,#13151,#13152,#13153,#13154,#13155,
#13156,#13157,#13158,#13159,#13160,#13161,#13162,#13163,#13164,#13165,#13166,
#13167,#13168,#13169,#13170,#13171,#13172,#13173,#13174,#13175),
 .UNSPECIFIED.,.F.,.F.,(4,3,3,3,3,3,3,3,3,3,3,3,3,3,3,3,3,3,3,4),(0.,0.0537020755871833,
0.0886281775480827,0.116609302441915,0.130919466980084,0.183454535593745,
0.216479678733881,0.230600801897488,0.244062529810022,0.292277144780066,
0.326690179741516,0.340044269166468,0.353800617376193,0.404857022677782,
0.431544028354177,0.447173043816862,0.495211725573931,0.52002062383812,
0.558026238582546,0.569248610399397),.UNSPECIFIED.);
#296=B_SPLINE_CURVE_WITH_KNOTS('',3,(#13177,#13178,#13179,#13180,#13181,
#13182,#13183,#13184,#13185,#13186,#13187),.UNSPECIFIED.,.F.,.F.,(4,1,1,
1,1,1,1,1,4),(15.7079632679489,15.8048324359278,16.7912933293328,17.7777542227378,
18.7642151161428,19.7506760095478,20.7371369029528,21.7235977963578,21.9911485751285),
 .UNSPECIFIED.);
#297=B_SPLINE_CURVE_WITH_KNOTS('',3,(#13188,#13189,#13190,#13191,#13192,
#13193,#13194,#13195,#13196,#13197),.UNSPECIFIED.,.F.,.F.,(4,1,1,1,1,1,
1,4),(15.7079632679489,16.3713219137818,17.3577828071869,18.3442437005919,
19.3307045939969,20.3171654874019,21.3036263808069,21.9911485751285),
 .UNSPECIFIED.);
#298=B_SPLINE_CURVE_WITH_KNOTS('',3,(#13422,#13423,#13424,#13425,#13426,
#13427,#13428,#13429,#13430,#13431,#13432,#13433,#13434,#13435,#13436,#13437,
#13438,#13439,#13440,#13441,#13442,#13443,#13444,#13445,#13446,#13447,#13448,
#13449,#13450,#13451,#13452,#13453,#13454,#13455,#13456,#13457,#13458,#13459,
#13460,#13461,#13462,#13463,#13464,#13465,#13466,#13467,#13468,#13469,#13470,
#13471,#13472,#13473,#13474,#13475,#13476,#13477,#13478,#13479),
 .UNSPECIFIED.,.F.,.F.,(4,3,3,3,3,3,3,3,3,3,3,3,3,3,3,3,3,3,3,4),(0.,0.0459570110528117,
0.0870590917382537,0.100825848948781,0.150050223975658,0.18408603179036,
0.203261017504252,0.216256506747385,0.263711469126848,0.302873338429924,
0.3210329008499,0.37204633625366,0.401845514966252,0.421231290165854,0.435656368582237,
0.47481241616036,0.492789265129085,0.511549883096662,0.553331205445843,
0.566847306048125),.UNSPECIFIED.);
#299=B_SPLINE_CURVE_WITH_KNOTS('',3,(#13480,#13481,#13482,#13483,#13484,
#13485,#13486,#13487,#13488,#13489,#13490,#13491,#13492,#13493,#13494,#13495,
#13496,#13497,#13498,#13499,#13500,#13501,#13502,#13503,#13504),
 .UNSPECIFIED.,.F.,.F.,(4,3,3,3,3,3,3,3,4),(-10.1321597128207,-9.86460893405003,
-8.87814804064502,-7.89168714724002,-6.90522625383502,-5.91876536043002,
-4.93230446702501,-3.94584357362001,-3.84897440564114),.UNSPECIFIED.);
#300=B_SPLINE_CURVE_WITH_KNOTS('',3,(#13729,#13730,#13731,#13732,#13733,
#13734,#13735,#13736,#13737,#13738,#13739,#13740,#13741,#13742,#13743,#13744,
#13745,#13746,#13747,#13748,#13749,#13750,#13751,#13752,#13753),
 .UNSPECIFIED.,.F.,.F.,(4,3,3,3,3,3,3,3,4),(7.59274844815667,7.89168714724002,
8.87814804064503,9.86460893405003,10.851069827455,11.83753072086,12.823991614265,
13.81045250767,13.8759337553363),.UNSPECIFIED.);
#301=B_SPLINE_CURVE_WITH_KNOTS('',3,(#13754,#13755,#13756,#13757,#13758,
#13759,#13760,#13761,#13762,#13763,#13764,#13765,#13766,#13767,#13768,#13769,
#13770,#13771,#13772,#13773,#13774,#13775,#13776,#13777,#13778,#13779,#13780,
#13781,#13782,#13783,#13784,#13785,#13786,#13787,#13788,#13789,#13790,#13791,
#13792,#13793,#13794,#13795,#13796,#13797,#13798,#13799,#13800,#13801,#13802,
#13803,#13804,#13805,#13806,#13807,#13808,#13809,#13810,#13811),
 .UNSPECIFIED.,.F.,.F.,(4,3,3,3,3,3,3,3,3,3,3,3,3,3,3,3,3,3,3,4),(0.,0.053702114036519,
0.0886282936969937,0.116609742583596,0.130919547118421,0.18345459729122,
0.216479693402787,0.230600807019328,0.244062535138244,0.292277144780066,
0.326690167328717,0.340044234449132,0.353800606005677,0.404857014149894,
0.431543724850428,0.447172872441803,0.495211547318113,0.520020652828403,
0.558026238582546,0.569248610399397),.UNSPECIFIED.);
#302=B_SPLINE_CURVE_WITH_KNOTS('',3,(#13813,#13814,#13815,#13816,#13817,
#13818,#13819,#13820,#13821,#13822,#13823),.UNSPECIFIED.,.F.,.F.,(4,1,1,
1,1,1,1,1,4),(15.7079632679489,15.8048324359278,16.7912933293328,17.7777542227378,
18.7642151161428,19.7506760095478,20.7371369029528,21.7235977963578,21.9911485751285),
 .UNSPECIFIED.);
#303=B_SPLINE_CURVE_WITH_KNOTS('',3,(#13824,#13825,#13826,#13827,#13828,
#13829,#13830,#13831,#13832,#13833),.UNSPECIFIED.,.F.,.F.,(4,1,1,1,1,1,
1,4),(15.7079632679489,16.3713219137818,17.3577828071869,18.3442437005919,
19.3307045939969,20.3171654874019,21.3036263808069,21.9911485751285),
 .UNSPECIFIED.);
#304=B_SPLINE_CURVE_WITH_KNOTS('',3,(#14058,#14059,#14060,#14061,#14062,
#14063,#14064,#14065,#14066,#14067,#14068,#14069,#14070,#14071,#14072,#14073,
#14074,#14075,#14076,#14077,#14078,#14079,#14080,#14081,#14082,#14083,#14084,
#14085,#14086,#14087,#14088,#14089,#14090,#14091,#14092,#14093,#14094,#14095,
#14096,#14097,#14098,#14099,#14100,#14101,#14102,#14103,#14104,#14105,#14106,
#14107,#14108,#14109,#14110,#14111,#14112,#14113,#14114,#14115),
 .UNSPECIFIED.,.F.,.F.,(4,3,3,3,3,3,3,3,3,3,3,3,3,3,3,3,3,3,3,4),(0.,0.0459570462372587,
0.0870589665518601,0.100825792431561,0.150050182199626,0.184086043156091,
0.203260918169112,0.216256494127592,0.263711469126833,0.302873334461669,
0.321032899868711,0.372046316136279,0.401845468535358,0.421231087805859,
0.435655940588184,0.474811855885159,0.492795623998078,0.511550636110964,
0.553331205445823,0.566847306048107),.UNSPECIFIED.);
#305=B_SPLINE_CURVE_WITH_KNOTS('',3,(#14116,#14117,#14118,#14119,#14120,
#14121,#14122,#14123,#14124,#14125,#14126,#14127,#14128,#14129,#14130,#14131,
#14132,#14133,#14134,#14135,#14136,#14137,#14138,#14139,#14140),
 .UNSPECIFIED.,.F.,.F.,(4,3,3,3,3,3,3,3,4),(-10.1321597128207,-9.86460893405003,
-8.87814804064502,-7.89168714724003,-6.90522625383502,-5.91876536043002,
-4.93230446702501,-3.94584357362001,-3.84897440564113),.UNSPECIFIED.);
#306=B_SPLINE_CURVE_WITH_KNOTS('',3,(#14365,#14366,#14367,#14368,#14369,
#14370,#14371,#14372,#14373,#14374,#14375,#14376,#14377,#14378,#14379,#14380,
#14381,#14382,#14383,#14384,#14385,#14386,#14387,#14388,#14389),
 .UNSPECIFIED.,.F.,.F.,(4,3,3,3,3,3,3,3,4),(7.59274844815667,7.89168714724002,
8.87814804064502,9.86460893405003,10.851069827455,11.83753072086,12.823991614265,
13.81045250767,13.8759337553363),.UNSPECIFIED.);
#307=B_SPLINE_CURVE_WITH_KNOTS('',3,(#14390,#14391,#14392,#14393,#14394,
#14395,#14396,#14397,#14398,#14399,#14400,#14401,#14402,#14403,#14404,#14405,
#14406,#14407,#14408,#14409,#14410,#14411,#14412,#14413,#14414,#14415,#14416,
#14417,#14418,#14419,#14420,#14421,#14422,#14423,#14424,#14425,#14426,#14427,
#14428,#14429,#14430,#14431,#14432,#14433,#14434,#14435,#14436,#14437,#14438,
#14439,#14440,#14441,#14442,#14443,#14444,#14445,#14446,#14447),
 .UNSPECIFIED.,.F.,.F.,(4,3,3,3,3,3,3,3,3,3,3,3,3,3,3,3,3,3,3,4),(0.,0.0537020755872334,
0.088628177548111,0.116609302442254,0.130919466980116,0.183454535593798,
0.216479678733695,0.230600801901911,0.244062529810737,0.292277144780056,
0.326690179741613,0.340044269176976,0.353800617378764,0.40485702267971,
0.431544028358992,0.447173043821804,0.495211725577524,0.520020623835711,
0.558026238582547,0.5692486103994),.UNSPECIFIED.);
#359=SHAPE_REPRESENTATION_RELATIONSHIP('SRR','None',#16768,#378);
#378=ADVANCED_BREP_SHAPE_REPRESENTATION('',(#416),#16672);
#397=STYLED_ITEM('',(#16869),#416);
#416=MANIFOLD_SOLID_BREP('Body1',#6116);
#477=FACE_BOUND('',#1256,.T.);
#478=FACE_BOUND('',#1258,.T.);
#479=FACE_BOUND('',#1259,.T.);
#480=FACE_BOUND('',#1260,.T.);
#481=FACE_BOUND('',#1261,.T.);
#482=FACE_BOUND('',#1266,.T.);
#483=FACE_BOUND('',#1267,.T.);
#484=FACE_BOUND('',#1268,.T.);
#485=FACE_BOUND('',#1269,.T.);
#486=FACE_BOUND('',#1270,.T.);
#487=FACE_BOUND('',#1289,.T.);
#488=FACE_BOUND('',#1290,.T.);
#489=FACE_BOUND('',#1291,.T.);
#490=FACE_BOUND('',#1292,.T.);
#491=FACE_BOUND('',#1293,.T.);
#492=FACE_BOUND('',#1296,.T.);
#493=FACE_BOUND('',#1297,.T.);
#494=FACE_BOUND('',#1298,.T.);
#495=FACE_BOUND('',#1299,.T.);
#496=FACE_BOUND('',#1300,.T.);
#497=FACE_BOUND('',#1308,.T.);
#498=FACE_BOUND('',#1315,.T.);
#499=FACE_BOUND('',#1316,.T.);
#500=FACE_BOUND('',#1317,.T.);
#501=FACE_BOUND('',#1318,.T.);
#502=FACE_BOUND('',#1319,.T.);
#614=PLANE('',#6649);
#615=PLANE('',#6650);
#616=PLANE('',#6660);
#617=PLANE('',#6682);
#618=PLANE('',#6687);
#619=PLANE('',#6690);
#620=PLANE('',#6691);
#621=PLANE('',#6692);
#622=PLANE('',#6693);
#623=PLANE('',#6698);
#624=PLANE('',#6707);
#625=PLANE('',#6708);
#626=PLANE('',#6710);
#796=FACE_OUTER_BOUND('',#1189,.T.);
#797=FACE_OUTER_BOUND('',#1190,.T.);
#798=FACE_OUTER_BOUND('',#1191,.T.);
#799=FACE_OUTER_BOUND('',#1192,.T.);
#800=FACE_OUTER_BOUND('',#1193,.T.);
#801=FACE_OUTER_BOUND('',#1194,.T.);
#802=FACE_OUTER_BOUND('',#1195,.T.);
#803=FACE_OUTER_BOUND('',#1196,.T.);
#804=FACE_OUTER_BOUND('',#1197,.T.);
#805=FACE_OUTER_BOUND('',#1198,.T.);
#806=FACE_OUTER_BOUND('',#1199,.T.);
#807=FACE_OUTER_BOUND('',#1200,.T.);
#808=FACE_OUTER_BOUND('',#1201,.T.);
#809=FACE_OUTER_BOUND('',#1202,.T.);
#810=FACE_OUTER_BOUND('',#1203,.T.);
#811=FACE_OUTER_BOUND('',#1204,.T.);
#812=FACE_OUTER_BOUND('',#1205,.T.);
#813=FACE_OUTER_BOUND('',#1206,.T.);
#814=FACE_OUTER_BOUND('',#1207,.T.);
#815=FACE_OUTER_BOUND('',#1208,.T.);
#816=FACE_OUTER_BOUND('',#1209,.T.);
#817=FACE_OUTER_BOUND('',#1210,.T.);
#818=FACE_OUTER_BOUND('',#1211,.T.);
#819=FACE_OUTER_BOUND('',#1212,.T.);
#820=FACE_OUTER_BOUND('',#1213,.T.);
#821=FACE_OUTER_BOUND('',#1214,.T.);
#822=FACE_OUTER_BOUND('',#1215,.T.);
#823=FACE_OUTER_BOUND('',#1216,.T.);
#824=FACE_OUTER_BOUND('',#1217,.T.);
#825=FACE_OUTER_BOUND('',#1218,.T.);
#826=FACE_OUTER_BOUND('',#1219,.T.);
#827=FACE_OUTER_BOUND('',#1220,.T.);
#828=FACE_OUTER_BOUND('',#1221,.T.);
#829=FACE_OUTER_BOUND('',#1222,.T.);
#830=FACE_OUTER_BOUND('',#1223,.T.);
#831=FACE_OUTER_BOUND('',#1224,.T.);
#832=FACE_OUTER_BOUND('',#1225,.T.);
#833=FACE_OUTER_BOUND('',#1226,.T.);
#834=FACE_OUTER_BOUND('',#1227,.T.);
#835=FACE_OUTER_BOUND('',#1228,.T.);
#836=FACE_OUTER_BOUND('',#1229,.T.);
#837=FACE_OUTER_BOUND('',#1230,.T.);
#838=FACE_OUTER_BOUND('',#1231,.T.);
#839=FACE_OUTER_BOUND('',#1232,.T.);
#840=FACE_OUTER_BOUND('',#1233,.T.);
#841=FACE_OUTER_BOUND('',#1234,.T.);
#842=FACE_OUTER_BOUND('',#1235,.T.);
#843=FACE_OUTER_BOUND('',#1236,.T.);
#844=FACE_OUTER_BOUND('',#1237,.T.);
#845=FACE_OUTER_BOUND('',#1238,.T.);
#846=FACE_OUTER_BOUND('',#1239,.T.);
#847=FACE_OUTER_BOUND('',#1240,.T.);
#848=FACE_OUTER_BOUND('',#1241,.T.);
#849=FACE_OUTER_BOUND('',#1242,.T.);
#850=FACE_OUTER_BOUND('',#1243,.T.);
#851=FACE_OUTER_BOUND('',#1244,.T.);
#852=FACE_OUTER_BOUND('',#1245,.T.);
#853=FACE_OUTER_BOUND('',#1246,.T.);
#854=FACE_OUTER_BOUND('',#1247,.T.);
#855=FACE_OUTER_BOUND('',#1248,.T.);
#856=FACE_OUTER_BOUND('',#1249,.T.);
#857=FACE_OUTER_BOUND('',#1250,.T.);
#858=FACE_OUTER_BOUND('',#1251,.T.);
#859=FACE_OUTER_BOUND('',#1252,.T.);
#860=FACE_OUTER_BOUND('',#1253,.T.);
#861=FACE_OUTER_BOUND('',#1254,.T.);
#862=FACE_OUTER_BOUND('',#1255,.T.);
#863=FACE_OUTER_BOUND('',#1257,.T.);
#864=FACE_OUTER_BOUND('',#1262,.T.);
#865=FACE_OUTER_BOUND('',#1263,.T.);
#866=FACE_OUTER_BOUND('',#1264,.T.);
#867=FACE_OUTER_BOUND('',#1265,.T.);
#868=FACE_OUTER_BOUND('',#1271,.T.);
#869=FACE_OUTER_BOUND('',#1272,.T.);
#870=FACE_OUTER_BOUND('',#1273,.T.);
#871=FACE_OUTER_BOUND('',#1274,.T.);
#872=FACE_OUTER_BOUND('',#1275,.T.);
#873=FACE_OUTER_BOUND('',#1276,.T.);
#874=FACE_OUTER_BOUND('',#1277,.T.);
#875=FACE_OUTER_BOUND('',#1278,.T.);
#876=FACE_OUTER_BOUND('',#1279,.T.);
#877=FACE_OUTER_BOUND('',#1280,.T.);
#878=FACE_OUTER_BOUND('',#1281,.T.);
#879=FACE_OUTER_BOUND('',#1282,.T.);
#880=FACE_OUTER_BOUND('',#1283,.T.);
#881=FACE_OUTER_BOUND('',#1284,.T.);
#882=FACE_OUTER_BOUND('',#1285,.T.);
#883=FACE_OUTER_BOUND('',#1286,.T.);
#884=FACE_OUTER_BOUND('',#1287,.T.);
#885=FACE_OUTER_BOUND('',#1288,.T.);
#886=FACE_OUTER_BOUND('',#1294,.T.);
#887=FACE_OUTER_BOUND('',#1295,.T.);
#888=FACE_OUTER_BOUND('',#1301,.T.);
#889=FACE_OUTER_BOUND('',#1302,.T.);
#890=FACE_OUTER_BOUND('',#1303,.T.);
#891=FACE_OUTER_BOUND('',#1304,.T.);
#892=FACE_OUTER_BOUND('',#1305,.T.);
#893=FACE_OUTER_BOUND('',#1306,.T.);
#894=FACE_OUTER_BOUND('',#1307,.T.);
#895=FACE_OUTER_BOUND('',#1309,.T.);
#896=FACE_OUTER_BOUND('',#1310,.T.);
#897=FACE_OUTER_BOUND('',#1311,.T.);
#898=FACE_OUTER_BOUND('',#1312,.T.);
#899=FACE_OUTER_BOUND('',#1313,.T.);
#900=FACE_OUTER_BOUND('',#1314,.T.);
#901=FACE_OUTER_BOUND('',#1320,.T.);
#902=FACE_OUTER_BOUND('',#1321,.T.);
#1189=EDGE_LOOP('',(#4407,#4408,#4409,#4410));
#1190=EDGE_LOOP('',(#4411,#4412,#4413,#4414));
#1191=EDGE_LOOP('',(#4415,#4416,#4417,#4418));
#1192=EDGE_LOOP('',(#4419,#4420,#4421,#4422));
#1193=EDGE_LOOP('',(#4423,#4424,#4425,#4426));
#1194=EDGE_LOOP('',(#4427,#4428,#4429,#4430));
#1195=EDGE_LOOP('',(#4431,#4432,#4433,#4434));
#1196=EDGE_LOOP('',(#4435,#4436,#4437,#4438));
#1197=EDGE_LOOP('',(#4439,#4440,#4441,#4442));
#1198=EDGE_LOOP('',(#4443,#4444,#4445,#4446));
#1199=EDGE_LOOP('',(#4447,#4448,#4449,#4450));
#1200=EDGE_LOOP('',(#4451,#4452,#4453,#4454));
#1201=EDGE_LOOP('',(#4455,#4456,#4457,#4458));
#1202=EDGE_LOOP('',(#4459,#4460,#4461,#4462));
#1203=EDGE_LOOP('',(#4463,#4464,#4465,#4466));
#1204=EDGE_LOOP('',(#4467,#4468,#4469,#4470));
#1205=EDGE_LOOP('',(#4471,#4472,#4473,#4474));
#1206=EDGE_LOOP('',(#4475,#4476,#4477,#4478));
#1207=EDGE_LOOP('',(#4479,#4480,#4481,#4482));
#1208=EDGE_LOOP('',(#4483,#4484,#4485,#4486));
#1209=EDGE_LOOP('',(#4487,#4488,#4489,#4490));
#1210=EDGE_LOOP('',(#4491,#4492,#4493,#4494));
#1211=EDGE_LOOP('',(#4495,#4496,#4497,#4498));
#1212=EDGE_LOOP('',(#4499,#4500,#4501,#4502));
#1213=EDGE_LOOP('',(#4503,#4504,#4505,#4506));
#1214=EDGE_LOOP('',(#4507,#4508,#4509,#4510));
#1215=EDGE_LOOP('',(#4511,#4512,#4513,#4514));
#1216=EDGE_LOOP('',(#4515,#4516,#4517,#4518));
#1217=EDGE_LOOP('',(#4519,#4520,#4521,#4522));
#1218=EDGE_LOOP('',(#4523,#4524,#4525,#4526));
#1219=EDGE_LOOP('',(#4527,#4528,#4529,#4530));
#1220=EDGE_LOOP('',(#4531,#4532,#4533,#4534));
#1221=EDGE_LOOP('',(#4535,#4536,#4537,#4538));
#1222=EDGE_LOOP('',(#4539,#4540,#4541,#4542));
#1223=EDGE_LOOP('',(#4543,#4544,#4545,#4546));
#1224=EDGE_LOOP('',(#4547,#4548,#4549,#4550));
#1225=EDGE_LOOP('',(#4551,#4552,#4553,#4554));
#1226=EDGE_LOOP('',(#4555,#4556,#4557,#4558));
#1227=EDGE_LOOP('',(#4559,#4560,#4561,#4562));
#1228=EDGE_LOOP('',(#4563,#4564,#4565,#4566));
#1229=EDGE_LOOP('',(#4567,#4568,#4569,#4570));
#1230=EDGE_LOOP('',(#4571,#4572,#4573,#4574));
#1231=EDGE_LOOP('',(#4575,#4576,#4577,#4578));
#1232=EDGE_LOOP('',(#4579,#4580,#4581,#4582));
#1233=EDGE_LOOP('',(#4583,#4584,#4585,#4586));
#1234=EDGE_LOOP('',(#4587,#4588,#4589,#4590));
#1235=EDGE_LOOP('',(#4591,#4592,#4593,#4594));
#1236=EDGE_LOOP('',(#4595,#4596,#4597,#4598));
#1237=EDGE_LOOP('',(#4599,#4600,#4601,#4602));
#1238=EDGE_LOOP('',(#4603,#4604,#4605,#4606));
#1239=EDGE_LOOP('',(#4607,#4608,#4609,#4610));
#1240=EDGE_LOOP('',(#4611,#4612,#4613,#4614));
#1241=EDGE_LOOP('',(#4615,#4616,#4617,#4618));
#1242=EDGE_LOOP('',(#4619,#4620,#4621,#4622));
#1243=EDGE_LOOP('',(#4623,#4624,#4625,#4626));
#1244=EDGE_LOOP('',(#4627,#4628,#4629,#4630));
#1245=EDGE_LOOP('',(#4631,#4632,#4633,#4634));
#1246=EDGE_LOOP('',(#4635,#4636,#4637,#4638));
#1247=EDGE_LOOP('',(#4639,#4640,#4641,#4642));
#1248=EDGE_LOOP('',(#4643,#4644,#4645,#4646));
#1249=EDGE_LOOP('',(#4647,#4648,#4649,#4650));
#1250=EDGE_LOOP('',(#4651,#4652,#4653,#4654));
#1251=EDGE_LOOP('',(#4655,#4656,#4657,#4658));
#1252=EDGE_LOOP('',(#4659,#4660,#4661,#4662));
#1253=EDGE_LOOP('',(#4663,#4664,#4665,#4666));
#1254=EDGE_LOOP('',(#4667,#4668,#4669,#4670));
#1255=EDGE_LOOP('',(#4671));
#1256=EDGE_LOOP('',(#4672));
#1257=EDGE_LOOP('',(#4673));
#1258=EDGE_LOOP('',(#4674,#4675,#4676,#4677,#4678));
#1259=EDGE_LOOP('',(#4679,#4680,#4681,#4682));
#1260=EDGE_LOOP('',(#4683,#4684,#4685,#4686));
#1261=EDGE_LOOP('',(#4687));
#1262=EDGE_LOOP('',(#4688,#4689,#4690,#4691));
#1263=EDGE_LOOP('',(#4692,#4693,#4694,#4695,#4696,#4697,#4698,#4699,#4700,
#4701,#4702,#4703,#4704,#4705,#4706,#4707,#4708,#4709,#4710,#4711));
#1264=EDGE_LOOP('',(#4712,#4713,#4714,#4715,#4716,#4717,#4718,#4719,#4720,
#4721,#4722,#4723,#4724,#4725,#4726,#4727,#4728,#4729,#4730,#4731));
#1265=EDGE_LOOP('',(#4732));
#1266=EDGE_LOOP('',(#4733));
#1267=EDGE_LOOP('',(#4734,#4735,#4736,#4737));
#1268=EDGE_LOOP('',(#4738,#4739,#4740,#4741));
#1269=EDGE_LOOP('',(#4742,#4743,#4744,#4745));
#1270=EDGE_LOOP('',(#4746,#4747,#4748,#4749));
#1271=EDGE_LOOP('',(#4750,#4751,#4752,#4753));
#1272=EDGE_LOOP('',(#4754,#4755,#4756,#4757,#4758,#4759,#4760,#4761,#4762,
#4763,#4764,#4765,#4766,#4767,#4768,#4769,#4770,#4771,#4772,#4773));
#1273=EDGE_LOOP('',(#4774,#4775,#4776,#4777,#4778,#4779,#4780,#4781,#4782,
#4783,#4784,#4785,#4786,#4787,#4788,#4789,#4790,#4791,#4792,#4793));
#1274=EDGE_LOOP('',(#4794,#4795,#4796,#4797));
#1275=EDGE_LOOP('',(#4798,#4799,#4800,#4801,#4802,#4803,#4804,#4805,#4806,
#4807,#4808,#4809,#4810,#4811,#4812,#4813,#4814,#4815,#4816,#4817));
#1276=EDGE_LOOP('',(#4818,#4819,#4820,#4821,#4822,#4823,#4824,#4825,#4826,
#4827,#4828,#4829,#4830,#4831,#4832,#4833,#4834,#4835,#4836,#4837));
#1277=EDGE_LOOP('',(#4838,#4839,#4840,#4841));
#1278=EDGE_LOOP('',(#4842,#4843,#4844,#4845,#4846,#4847,#4848,#4849,#4850,
#4851,#4852,#4853,#4854,#4855,#4856,#4857,#4858,#4859,#4860,#4861));
#1279=EDGE_LOOP('',(#4862,#4863,#4864,#4865,#4866,#4867,#4868,#4869,#4870,
#4871,#4872,#4873,#4874,#4875,#4876,#4877,#4878,#4879,#4880,#4881));
#1280=EDGE_LOOP('',(#4882,#4883,#4884,#4885));
#1281=EDGE_LOOP('',(#4886,#4887,#4888,#4889));
#1282=EDGE_LOOP('',(#4890,#4891,#4892,#4893));
#1283=EDGE_LOOP('',(#4894,#4895,#4896,#4897));
#1284=EDGE_LOOP('',(#4898,#4899,#4900,#4901));
#1285=EDGE_LOOP('',(#4902,#4903,#4904,#4905));
#1286=EDGE_LOOP('',(#4906,#4907,#4908,#4909));
#1287=EDGE_LOOP('',(#4910,#4911,#4912,#4913));
#1288=EDGE_LOOP('',(#4914));
#1289=EDGE_LOOP('',(#4915));
#1290=EDGE_LOOP('',(#4916));
#1291=EDGE_LOOP('',(#4917));
#1292=EDGE_LOOP('',(#4918));
#1293=EDGE_LOOP('',(#4919));
#1294=EDGE_LOOP('',(#4920,#4921,#4922,#4923));
#1295=EDGE_LOOP('',(#4924));
#1296=EDGE_LOOP('',(#4925));
#1297=EDGE_LOOP('',(#4926));
#1298=EDGE_LOOP('',(#4927));
#1299=EDGE_LOOP('',(#4928));
#1300=EDGE_LOOP('',(#4929));
#1301=EDGE_LOOP('',(#4930,#4931,#4932,#4933));
#1302=EDGE_LOOP('',(#4934,#4935,#4936,#4937));
#1303=EDGE_LOOP('',(#4938,#4939,#4940,#4941));
#1304=EDGE_LOOP('',(#4942,#4943,#4944,#4945));
#1305=EDGE_LOOP('',(#4946,#4947,#4948,#4949));
#1306=EDGE_LOOP('',(#4950,#4951,#4952,#4953,#4954,#4955,#4956,#4957,#4958,
#4959,#4960,#4961,#4962,#4963,#4964,#4965));
#1307=EDGE_LOOP('',(#4966,#4967,#4968,#4969,#4970,#4971,#4972,#4973,#4974,
#4975,#4976,#4977));
#1308=EDGE_LOOP('',(#4978));
#1309=EDGE_LOOP('',(#4979,#4980,#4981,#4982));
#1310=EDGE_LOOP('',(#4983,#4984,#4985,#4986));
#1311=EDGE_LOOP('',(#4987,#4988,#4989,#4990));
#1312=EDGE_LOOP('',(#4991,#4992,#4993,#4994));
#1313=EDGE_LOOP('',(#4995,#4996,#4997,#4998));
#1314=EDGE_LOOP('',(#4999));
#1315=EDGE_LOOP('',(#5000,#5001,#5002,#5003));
#1316=EDGE_LOOP('',(#5004,#5005,#5006,#5007));
#1317=EDGE_LOOP('',(#5008,#5009,#5010,#5011));
#1318=EDGE_LOOP('',(#5012,#5013,#5014,#5015));
#1319=EDGE_LOOP('',(#5016));
#1320=EDGE_LOOP('',(#5017,#5018,#5019,#5020));
#1321=EDGE_LOOP('',(#5021,#5022,#5023,#5024));
#1654=LINE('',#9200,#2023);
#1655=LINE('',#9221,#2024);
#1656=LINE('',#9272,#2025);
#1657=LINE('',#9323,#2026);
#1658=LINE('',#9371,#2027);
#1659=LINE('',#9422,#2028);
#1660=LINE('',#9473,#2029);
#1661=LINE('',#9521,#2030);
#1662=LINE('',#9560,#2031);
#1663=LINE('',#9581,#2032);
#1664=LINE('',#9632,#2033);
#1665=LINE('',#9683,#2034);
#1666=LINE('',#9731,#2035);
#1667=LINE('',#9782,#2036);
#1668=LINE('',#9833,#2037);
#1669=LINE('',#9881,#2038);
#1670=LINE('',#9920,#2039);
#1671=LINE('',#9941,#2040);
#1672=LINE('',#9992,#2041);
#1673=LINE('',#10043,#2042);
#1674=LINE('',#10091,#2043);
#1675=LINE('',#10142,#2044);
#1676=LINE('',#10193,#2045);
#1677=LINE('',#10241,#2046);
#1678=LINE('',#10280,#2047);
#1679=LINE('',#10301,#2048);
#1680=LINE('',#10352,#2049);
#1681=LINE('',#10403,#2050);
#1682=LINE('',#10451,#2051);
#1683=LINE('',#10502,#2052);
#1684=LINE('',#10553,#2053);
#1685=LINE('',#10601,#2054);
#1686=LINE('',#10640,#2055);
#1687=LINE('',#10664,#2056);
#1688=LINE('',#10688,#2057);
#1689=LINE('',#10713,#2058);
#1690=LINE('',#10738,#2059);
#1691=LINE('',#10762,#2060);
#1692=LINE('',#10787,#2061);
#1693=LINE('',#10812,#2062);
#1694=LINE('',#10829,#2063);
#1695=LINE('',#10853,#2064);
#1696=LINE('',#10877,#2065);
#1697=LINE('',#10902,#2066);
#1698=LINE('',#10927,#2067);
#1699=LINE('',#10951,#2068);
#1700=LINE('',#10976,#2069);
#1701=LINE('',#11001,#2070);
#1702=LINE('',#11018,#2071);
#1703=LINE('',#11042,#2072);
#1704=LINE('',#11066,#2073);
#1705=LINE('',#11091,#2074);
#1706=LINE('',#11116,#2075);
#1707=LINE('',#11140,#2076);
#1708=LINE('',#11165,#2077);
#1709=LINE('',#11190,#2078);
#1710=LINE('',#11207,#2079);
#1711=LINE('',#11231,#2080);
#1712=LINE('',#11255,#2081);
#1713=LINE('',#11280,#2082);
#1714=LINE('',#11305,#2083);
#1715=LINE('',#11329,#2084);
#1716=LINE('',#11354,#2085);
#1717=LINE('',#11379,#2086);
#1718=LINE('',#11397,#2087);
#1719=LINE('',#11403,#2088);
#1720=LINE('',#11413,#2089);
#1721=LINE('',#11416,#2090);
#1722=LINE('',#11421,#2091);
#1723=LINE('',#11424,#2092);
#1724=LINE('',#11427,#2093);
#1725=LINE('',#11431,#2094);
#1726=LINE('',#14456,#2095);
#1727=LINE('',#14462,#2096);
#1728=LINE('',#14468,#2097);
#1729=LINE('',#14474,#2098);
#1730=LINE('',#14483,#2099);
#1731=LINE('',#14489,#2100);
#1732=LINE('',#14492,#2101);
#1733=LINE('',#14494,#2102);
#1734=LINE('',#14495,#2103);
#1735=LINE('',#14498,#2104);
#1736=LINE('',#14500,#2105);
#1737=LINE('',#14501,#2106);
#1738=LINE('',#14504,#2107);
#1739=LINE('',#14506,#2108);
#1740=LINE('',#14507,#2109);
#1741=LINE('',#14510,#2110);
#1742=LINE('',#14512,#2111);
#1743=LINE('',#14513,#2112);
#1744=LINE('',#14516,#2113);
#1745=LINE('',#14519,#2114);
#1746=LINE('',#14521,#2115);
#1747=LINE('',#14525,#2116);
#1748=LINE('',#14530,#2117);
#1749=LINE('',#14534,#2118);
#1750=LINE('',#14537,#2119);
#1751=LINE('',#14539,#2120);
#1752=LINE('',#14546,#2121);
#2023=VECTOR('',#7586,0.3);
#2024=VECTOR('',#7591,0.3);
#2025=VECTOR('',#7594,0.3);
#2026=VECTOR('',#7597,0.3);
#2027=VECTOR('',#7600,0.3);
#2028=VECTOR('',#7603,0.3);
#2029=VECTOR('',#7606,0.3);
#2030=VECTOR('',#7609,0.3);
#2031=VECTOR('',#7614,0.3);
#2032=VECTOR('',#7619,0.3);
#2033=VECTOR('',#7622,0.3);
#2034=VECTOR('',#7625,0.3);
#2035=VECTOR('',#7628,0.3);
#2036=VECTOR('',#7631,0.3);
#2037=VECTOR('',#7634,0.3);
#2038=VECTOR('',#7637,0.3);
#2039=VECTOR('',#7642,0.3);
#2040=VECTOR('',#7647,0.3);
#2041=VECTOR('',#7650,0.3);
#2042=VECTOR('',#7653,0.3);
#2043=VECTOR('',#7656,0.3);
#2044=VECTOR('',#7659,0.3);
#2045=VECTOR('',#7662,0.3);
#2046=VECTOR('',#7665,0.3);
#2047=VECTOR('',#7670,0.3);
#2048=VECTOR('',#7675,0.3);
#2049=VECTOR('',#7678,0.3);
#2050=VECTOR('',#7681,0.3);
#2051=VECTOR('',#7684,0.3);
#2052=VECTOR('',#7687,0.3);
#2053=VECTOR('',#7690,0.3);
#2054=VECTOR('',#7693,0.3);
#2055=VECTOR('',#7698,0.30735);
#2056=VECTOR('',#7703,0.30735);
#2057=VECTOR('',#7706,0.30735);
#2058=VECTOR('',#7709,0.30735);
#2059=VECTOR('',#7712,0.30735);
#2060=VECTOR('',#7715,0.30735);
#2061=VECTOR('',#7718,0.30735);
#2062=VECTOR('',#7721,0.30735);
#2063=VECTOR('',#7726,0.30735);
#2064=VECTOR('',#7731,0.30735);
#2065=VECTOR('',#7734,0.30735);
#2066=VECTOR('',#7737,0.30735);
#2067=VECTOR('',#7740,0.30735);
#2068=VECTOR('',#7743,0.30735);
#2069=VECTOR('',#7746,0.30735);
#2070=VECTOR('',#7749,0.30735);
#2071=VECTOR('',#7754,0.30735);
#2072=VECTOR('',#7759,0.30735);
#2073=VECTOR('',#7762,0.30735);
#2074=VECTOR('',#7765,0.30735);
#2075=VECTOR('',#7768,0.30735);
#2076=VECTOR('',#7771,0.30735);
#2077=VECTOR('',#7774,0.30735);
#2078=VECTOR('',#7777,0.30735);
#2079=VECTOR('',#7782,0.30735);
#2080=VECTOR('',#7787,0.30735);
#2081=VECTOR('',#7790,0.30735);
#2082=VECTOR('',#7793,0.30735);
#2083=VECTOR('',#7796,0.30735);
#2084=VECTOR('',#7799,0.30735);
#2085=VECTOR('',#7802,0.30735);
#2086=VECTOR('',#7805,0.30735);
#2087=VECTOR('',#7812,6.35);
#2088=VECTOR('',#7819,6.85);
#2089=VECTOR('',#7830,1.);
#2090=VECTOR('',#7833,1.);
#2091=VECTOR('',#7836,1.);
#2092=VECTOR('',#7839,1.);
#2093=VECTOR('',#7840,1.);
#2094=VECTOR('',#7843,1.);
#2095=VECTOR('',#7874,0.35);
#2096=VECTOR('',#7881,0.35);
#2097=VECTOR('',#7888,0.35);
#2098=VECTOR('',#7895,0.35);
#2099=VECTOR('',#7906,4.8);
#2100=VECTOR('',#7915,3.5);
#2101=VECTOR('',#7918,1.);
#2102=VECTOR('',#7919,1.);
#2103=VECTOR('',#7920,1.);
#2104=VECTOR('',#7923,1.);
#2105=VECTOR('',#7924,1.);
#2106=VECTOR('',#7925,1.);
#2107=VECTOR('',#7928,1.);
#2108=VECTOR('',#7929,1.);
#2109=VECTOR('',#7930,1.);
#2110=VECTOR('',#7933,1.);
#2111=VECTOR('',#7934,1.);
#2112=VECTOR('',#7935,1.);
#2113=VECTOR('',#7938,1.);
#2114=VECTOR('',#7941,1.);
#2115=VECTOR('',#7944,2.7);
#2116=VECTOR('',#7949,1.);
#2117=VECTOR('',#7956,1.);
#2118=VECTOR('',#7961,1.);
#2119=VECTOR('',#7966,1.7);
#2120=VECTOR('',#7969,1.);
#2121=VECTOR('',#7980,8.2);
#2346=CIRCLE('',#6564,0.25175);
#2347=CIRCLE('',#6572,0.25175);
#2348=CIRCLE('',#6574,0.25175);
#2349=CIRCLE('',#6582,0.25175);
#2350=CIRCLE('',#6584,0.25175);
#2351=CIRCLE('',#6592,0.25175);
#2352=CIRCLE('',#6594,0.25175);
#2353=CIRCLE('',#6602,0.25175);
#2354=CIRCLE('',#6604,0.30735);
#2355=CIRCLE('',#6612,0.30735);
#2356=CIRCLE('',#6614,0.30735);
#2357=CIRCLE('',#6622,0.30735);
#2358=CIRCLE('',#6624,0.30735);
#2359=CIRCLE('',#6632,0.30735);
#2360=CIRCLE('',#6634,0.30735);
#2361=CIRCLE('',#6642,0.30735);
#2362=CIRCLE('',#6644,6.35);
#2363=CIRCLE('',#6645,6.35);
#2364=CIRCLE('',#6647,6.85);
#2365=CIRCLE('',#6648,6.85);
#2366=CIRCLE('',#6651,2.7);
#2367=CIRCLE('',#6652,2.7);
#2368=CIRCLE('',#6653,2.1);
#2369=CIRCLE('',#6654,2.7);
#2370=CIRCLE('',#6655,2.1);
#2371=CIRCLE('',#6656,2.1);
#2372=CIRCLE('',#6657,2.7);
#2373=CIRCLE('',#6658,1.7);
#2374=CIRCLE('',#6661,8.2);
#2375=CIRCLE('',#6662,3.5);
#2376=CIRCLE('',#6671,0.35);
#2377=CIRCLE('',#6672,0.35);
#2378=CIRCLE('',#6674,0.35);
#2379=CIRCLE('',#6675,0.35);
#2380=CIRCLE('',#6677,0.35);
#2381=CIRCLE('',#6678,0.35);
#2382=CIRCLE('',#6680,0.35);
#2383=CIRCLE('',#6681,0.35);
#2384=CIRCLE('',#6683,4.8);
#2385=CIRCLE('',#6684,3.5);
#2386=CIRCLE('',#6686,4.8);
#2387=CIRCLE('',#6688,2.7);
#2388=CIRCLE('',#6695,2.7);
#2389=CIRCLE('',#6696,2.7);
#2390=CIRCLE('',#6697,2.7);
#2391=CIRCLE('',#6699,2.1);
#2392=CIRCLE('',#6700,2.1);
#2393=CIRCLE('',#6701,2.1);
#2394=CIRCLE('',#6702,1.7);
#2395=CIRCLE('',#6709,8.2);
#2671=VERTEX_POINT('',#9198);
#2672=VERTEX_POINT('',#9199);
#2673=VERTEX_POINT('',#9201);
#2674=VERTEX_POINT('',#9206);
#2675=VERTEX_POINT('',#9219);
#2676=VERTEX_POINT('',#9220);
#2677=VERTEX_POINT('',#9270);
#2678=VERTEX_POINT('',#9271);
#2679=VERTEX_POINT('',#9321);
#2680=VERTEX_POINT('',#9322);
#2681=VERTEX_POINT('',#9369);
#2682=VERTEX_POINT('',#9370);
#2683=VERTEX_POINT('',#9420);
#2684=VERTEX_POINT('',#9421);
#2685=VERTEX_POINT('',#9471);
#2686=VERTEX_POINT('',#9472);
#2687=VERTEX_POINT('',#9519);
#2688=VERTEX_POINT('',#9520);
#2689=VERTEX_POINT('',#9522);
#2690=VERTEX_POINT('',#9536);
#2691=VERTEX_POINT('',#9558);
#2692=VERTEX_POINT('',#9559);
#2693=VERTEX_POINT('',#9561);
#2694=VERTEX_POINT('',#9566);
#2695=VERTEX_POINT('',#9579);
#2696=VERTEX_POINT('',#9580);
#2697=VERTEX_POINT('',#9630);
#2698=VERTEX_POINT('',#9631);
#2699=VERTEX_POINT('',#9681);
#2700=VERTEX_POINT('',#9682);
#2701=VERTEX_POINT('',#9729);
#2702=VERTEX_POINT('',#9730);
#2703=VERTEX_POINT('',#9780);
#2704=VERTEX_POINT('',#9781);
#2705=VERTEX_POINT('',#9831);
#2706=VERTEX_POINT('',#9832);
#2707=VERTEX_POINT('',#9879);
#2708=VERTEX_POINT('',#9880);
#2709=VERTEX_POINT('',#9882);
#2710=VERTEX_POINT('',#9896);
#2711=VERTEX_POINT('',#9918);
#2712=VERTEX_POINT('',#9919);
#2713=VERTEX_POINT('',#9921);
#2714=VERTEX_POINT('',#9926);
#2715=VERTEX_POINT('',#9939);
#2716=VERTEX_POINT('',#9940);
#2717=VERTEX_POINT('',#9990);
#2718=VERTEX_POINT('',#9991);
#2719=VERTEX_POINT('',#10041);
#2720=VERTEX_POINT('',#10042);
#2721=VERTEX_POINT('',#10089);
#2722=VERTEX_POINT('',#10090);
#2723=VERTEX_POINT('',#10140);
#2724=VERTEX_POINT('',#10141);
#2725=VERTEX_POINT('',#10191);
#2726=VERTEX_POINT('',#10192);
#2727=VERTEX_POINT('',#10239);
#2728=VERTEX_POINT('',#10240);
#2729=VERTEX_POINT('',#10242);
#2730=VERTEX_POINT('',#10256);
#2731=VERTEX_POINT('',#10278);
#2732=VERTEX_POINT('',#10279);
#2733=VERTEX_POINT('',#10281);
#2734=VERTEX_POINT('',#10286);
#2735=VERTEX_POINT('',#10299);
#2736=VERTEX_POINT('',#10300);
#2737=VERTEX_POINT('',#10350);
#2738=VERTEX_POINT('',#10351);
#2739=VERTEX_POINT('',#10401);
#2740=VERTEX_POINT('',#10402);
#2741=VERTEX_POINT('',#10449);
#2742=VERTEX_POINT('',#10450);
#2743=VERTEX_POINT('',#10500);
#2744=VERTEX_POINT('',#10501);
#2745=VERTEX_POINT('',#10551);
#2746=VERTEX_POINT('',#10552);
#2747=VERTEX_POINT('',#10599);
#2748=VERTEX_POINT('',#10600);
#2749=VERTEX_POINT('',#10602);
#2750=VERTEX_POINT('',#10616);
#2751=VERTEX_POINT('',#10638);
#2752=VERTEX_POINT('',#10639);
#2753=VERTEX_POINT('',#10641);
#2754=VERTEX_POINT('',#10650);
#2755=VERTEX_POINT('',#10662);
#2756=VERTEX_POINT('',#10663);
#2757=VERTEX_POINT('',#10686);
#2758=VERTEX_POINT('',#10687);
#2759=VERTEX_POINT('',#10711);
#2760=VERTEX_POINT('',#10712);
#2761=VERTEX_POINT('',#10736);
#2762=VERTEX_POINT('',#10737);
#2763=VERTEX_POINT('',#10760);
#2764=VERTEX_POINT('',#10761);
#2765=VERTEX_POINT('',#10785);
#2766=VERTEX_POINT('',#10786);
#2767=VERTEX_POINT('',#10810);
#2768=VERTEX_POINT('',#10811);
#2769=VERTEX_POINT('',#10813);
#2770=VERTEX_POINT('',#10819);
#2771=VERTEX_POINT('',#10827);
#2772=VERTEX_POINT('',#10828);
#2773=VERTEX_POINT('',#10830);
#2774=VERTEX_POINT('',#10839);
#2775=VERTEX_POINT('',#10851);
#2776=VERTEX_POINT('',#10852);
#2777=VERTEX_POINT('',#10875);
#2778=VERTEX_POINT('',#10876);
#2779=VERTEX_POINT('',#10900);
#2780=VERTEX_POINT('',#10901);
#2781=VERTEX_POINT('',#10925);
#2782=VERTEX_POINT('',#10926);
#2783=VERTEX_POINT('',#10949);
#2784=VERTEX_POINT('',#10950);
#2785=VERTEX_POINT('',#10974);
#2786=VERTEX_POINT('',#10975);
#2787=VERTEX_POINT('',#10999);
#2788=VERTEX_POINT('',#11000);
#2789=VERTEX_POINT('',#11002);
#2790=VERTEX_POINT('',#11008);
#2791=VERTEX_POINT('',#11016);
#2792=VERTEX_POINT('',#11017);
#2793=VERTEX_POINT('',#11019);
#2794=VERTEX_POINT('',#11028);
#2795=VERTEX_POINT('',#11040);
#2796=VERTEX_POINT('',#11041);
#2797=VERTEX_POINT('',#11064);
#2798=VERTEX_POINT('',#11065);
#2799=VERTEX_POINT('',#11089);
#2800=VERTEX_POINT('',#11090);
#2801=VERTEX_POINT('',#11114);
#2802=VERTEX_POINT('',#11115);
#2803=VERTEX_POINT('',#11138);
#2804=VERTEX_POINT('',#11139);
#2805=VERTEX_POINT('',#11163);
#2806=VERTEX_POINT('',#11164);
#2807=VERTEX_POINT('',#11188);
#2808=VERTEX_POINT('',#11189);
#2809=VERTEX_POINT('',#11191);
#2810=VERTEX_POINT('',#11197);
#2811=VERTEX_POINT('',#11205);
#2812=VERTEX_POINT('',#11206);
#2813=VERTEX_POINT('',#11208);
#2814=VERTEX_POINT('',#11217);
#2815=VERTEX_POINT('',#11229);
#2816=VERTEX_POINT('',#11230);
#2817=VERTEX_POINT('',#11253);
#2818=VERTEX_POINT('',#11254);
#2819=VERTEX_POINT('',#11278);
#2820=VERTEX_POINT('',#11279);
#2821=VERTEX_POINT('',#11303);
#2822=VERTEX_POINT('',#11304);
#2823=VERTEX_POINT('',#11327);
#2824=VERTEX_POINT('',#11328);
#2825=VERTEX_POINT('',#11352);
#2826=VERTEX_POINT('',#11353);
#2827=VERTEX_POINT('',#11377);
#2828=VERTEX_POINT('',#11378);
#2829=VERTEX_POINT('',#11380);
#2830=VERTEX_POINT('',#11386);
#2831=VERTEX_POINT('',#11394);
#2832=VERTEX_POINT('',#11396);
#2833=VERTEX_POINT('',#11400);
#2834=VERTEX_POINT('',#11402);
#2835=VERTEX_POINT('',#11407);
#2836=VERTEX_POINT('',#11408);
#2837=VERTEX_POINT('',#11410);
#2838=VERTEX_POINT('',#11412);
#2839=VERTEX_POINT('',#11414);
#2840=VERTEX_POINT('',#11417);
#2841=VERTEX_POINT('',#11418);
#2842=VERTEX_POINT('',#11420);
#2843=VERTEX_POINT('',#11422);
#2844=VERTEX_POINT('',#11425);
#2845=VERTEX_POINT('',#11426);
#2846=VERTEX_POINT('',#11428);
#2847=VERTEX_POINT('',#11430);
#2848=VERTEX_POINT('',#11433);
#2849=VERTEX_POINT('',#12188);
#2850=VERTEX_POINT('',#12190);
#2851=VERTEX_POINT('',#14453);
#2852=VERTEX_POINT('',#14455);
#2853=VERTEX_POINT('',#14459);
#2854=VERTEX_POINT('',#14461);
#2855=VERTEX_POINT('',#14465);
#2856=VERTEX_POINT('',#14467);
#2857=VERTEX_POINT('',#14471);
#2858=VERTEX_POINT('',#14473);
#2859=VERTEX_POINT('',#14477);
#2860=VERTEX_POINT('',#14479);
#2861=VERTEX_POINT('',#14482);
#2862=VERTEX_POINT('',#14486);
#2863=VERTEX_POINT('',#14491);
#2864=VERTEX_POINT('',#14493);
#2865=VERTEX_POINT('',#14497);
#2866=VERTEX_POINT('',#14499);
#2867=VERTEX_POINT('',#14503);
#2868=VERTEX_POINT('',#14505);
#2869=VERTEX_POINT('',#14509);
#2870=VERTEX_POINT('',#14511);
#2871=VERTEX_POINT('',#14515);
#2872=VERTEX_POINT('',#14517);
#2873=VERTEX_POINT('',#14524);
#2874=VERTEX_POINT('',#14528);
#2875=VERTEX_POINT('',#14531);
#2876=VERTEX_POINT('',#14542);
#3313=EDGE_CURVE('',#2671,#2672,#1654,.T.);
#3314=EDGE_CURVE('',#2672,#2673,#148,.T.);
#3315=EDGE_CURVE('',#2674,#2673,#2346,.F.);
#3316=EDGE_CURVE('',#2674,#2671,#149,.T.);
#3317=EDGE_CURVE('',#2675,#2676,#1655,.T.);
#3318=EDGE_CURVE('',#2676,#2672,#150,.T.);
#3319=EDGE_CURVE('',#2671,#2675,#151,.T.);
#3320=EDGE_CURVE('',#2677,#2678,#1656,.T.);
#3321=EDGE_CURVE('',#2678,#2676,#152,.T.);
#3322=EDGE_CURVE('',#2675,#2677,#153,.T.);
#3323=EDGE_CURVE('',#2679,#2680,#1657,.T.);
#3324=EDGE_CURVE('',#2680,#2678,#154,.T.);
#3325=EDGE_CURVE('',#2677,#2679,#155,.T.);
#3326=EDGE_CURVE('',#2681,#2682,#1658,.T.);
#3327=EDGE_CURVE('',#2682,#2680,#156,.T.);
#3328=EDGE_CURVE('',#2679,#2681,#157,.T.);
#3329=EDGE_CURVE('',#2683,#2684,#1659,.T.);
#3330=EDGE_CURVE('',#2684,#2682,#158,.T.);
#3331=EDGE_CURVE('',#2681,#2683,#159,.T.);
#3332=EDGE_CURVE('',#2685,#2686,#1660,.T.);
#3333=EDGE_CURVE('',#2686,#2684,#160,.T.);
#3334=EDGE_CURVE('',#2683,#2685,#161,.T.);
#3335=EDGE_CURVE('',#2687,#2688,#1661,.T.);
#3336=EDGE_CURVE('',#2687,#2689,#162,.T.);
#3337=EDGE_CURVE('',#2690,#2689,#2347,.T.);
#3338=EDGE_CURVE('',#2690,#2688,#163,.T.);
#3339=EDGE_CURVE('',#2691,#2692,#1662,.T.);
#3340=EDGE_CURVE('',#2692,#2693,#164,.T.);
#3341=EDGE_CURVE('',#2694,#2693,#2348,.F.);
#3342=EDGE_CURVE('',#2694,#2691,#165,.T.);
#3343=EDGE_CURVE('',#2695,#2696,#1663,.T.);
#3344=EDGE_CURVE('',#2696,#2692,#166,.T.);
#3345=EDGE_CURVE('',#2691,#2695,#167,.T.);
#3346=EDGE_CURVE('',#2697,#2698,#1664,.T.);
#3347=EDGE_CURVE('',#2698,#2696,#168,.T.);
#3348=EDGE_CURVE('',#2695,#2697,#169,.T.);
#3349=EDGE_CURVE('',#2699,#2700,#1665,.T.);
#3350=EDGE_CURVE('',#2700,#2698,#170,.T.);
#3351=EDGE_CURVE('',#2697,#2699,#171,.T.);
#3352=EDGE_CURVE('',#2701,#2702,#1666,.T.);
#3353=EDGE_CURVE('',#2702,#2700,#172,.T.);
#3354=EDGE_CURVE('',#2699,#2701,#173,.T.);
#3355=EDGE_CURVE('',#2703,#2704,#1667,.T.);
#3356=EDGE_CURVE('',#2704,#2702,#174,.T.);
#3357=EDGE_CURVE('',#2701,#2703,#175,.T.);
#3358=EDGE_CURVE('',#2705,#2706,#1668,.T.);
#3359=EDGE_CURVE('',#2706,#2704,#176,.T.);
#3360=EDGE_CURVE('',#2703,#2705,#177,.T.);
#3361=EDGE_CURVE('',#2707,#2708,#1669,.T.);
#3362=EDGE_CURVE('',#2707,#2709,#178,.T.);
#3363=EDGE_CURVE('',#2710,#2709,#2349,.T.);
#3364=EDGE_CURVE('',#2710,#2708,#179,.T.);
#3365=EDGE_CURVE('',#2711,#2712,#1670,.T.);
#3366=EDGE_CURVE('',#2712,#2713,#180,.T.);
#3367=EDGE_CURVE('',#2714,#2713,#2350,.F.);
#3368=EDGE_CURVE('',#2714,#2711,#181,.T.);
#3369=EDGE_CURVE('',#2715,#2716,#1671,.T.);
#3370=EDGE_CURVE('',#2716,#2712,#182,.T.);
#3371=EDGE_CURVE('',#2711,#2715,#183,.T.);
#3372=EDGE_CURVE('',#2717,#2718,#1672,.T.);
#3373=EDGE_CURVE('',#2718,#2716,#184,.T.);
#3374=EDGE_CURVE('',#2715,#2717,#185,.T.);
#3375=EDGE_CURVE('',#2719,#2720,#1673,.T.);
#3376=EDGE_CURVE('',#2720,#2718,#186,.T.);
#3377=EDGE_CURVE('',#2717,#2719,#187,.T.);
#3378=EDGE_CURVE('',#2721,#2722,#1674,.T.);
#3379=EDGE_CURVE('',#2722,#2720,#188,.T.);
#3380=EDGE_CURVE('',#2719,#2721,#189,.T.);
#3381=EDGE_CURVE('',#2723,#2724,#1675,.T.);
#3382=EDGE_CURVE('',#2724,#2722,#190,.T.);
#3383=EDGE_CURVE('',#2721,#2723,#191,.T.);
#3384=EDGE_CURVE('',#2725,#2726,#1676,.T.);
#3385=EDGE_CURVE('',#2726,#2724,#192,.T.);
#3386=EDGE_CURVE('',#2723,#2725,#193,.T.);
#3387=EDGE_CURVE('',#2727,#2728,#1677,.T.);
#3388=EDGE_CURVE('',#2727,#2729,#194,.T.);
#3389=EDGE_CURVE('',#2730,#2729,#2351,.T.);
#3390=EDGE_CURVE('',#2730,#2728,#195,.T.);
#3391=EDGE_CURVE('',#2731,#2732,#1678,.T.);
#3392=EDGE_CURVE('',#2732,#2733,#196,.T.);
#3393=EDGE_CURVE('',#2734,#2733,#2352,.F.);
#3394=EDGE_CURVE('',#2734,#2731,#197,.T.);
#3395=EDGE_CURVE('',#2735,#2736,#1679,.T.);
#3396=EDGE_CURVE('',#2736,#2732,#198,.T.);
#3397=EDGE_CURVE('',#2731,#2735,#199,.T.);
#3398=EDGE_CURVE('',#2737,#2738,#1680,.T.);
#3399=EDGE_CURVE('',#2738,#2736,#200,.T.);
#3400=EDGE_CURVE('',#2735,#2737,#201,.T.);
#3401=EDGE_CURVE('',#2739,#2740,#1681,.T.);
#3402=EDGE_CURVE('',#2740,#2738,#202,.T.);
#3403=EDGE_CURVE('',#2737,#2739,#203,.T.);
#3404=EDGE_CURVE('',#2741,#2742,#1682,.T.);
#3405=EDGE_CURVE('',#2742,#2740,#204,.T.);
#3406=EDGE_CURVE('',#2739,#2741,#205,.T.);
#3407=EDGE_CURVE('',#2743,#2744,#1683,.T.);
#3408=EDGE_CURVE('',#2744,#2742,#206,.T.);
#3409=EDGE_CURVE('',#2741,#2743,#207,.T.);
#3410=EDGE_CURVE('',#2745,#2746,#1684,.T.);
#3411=EDGE_CURVE('',#2746,#2744,#208,.T.);
#3412=EDGE_CURVE('',#2743,#2745,#209,.T.);
#3413=EDGE_CURVE('',#2747,#2748,#1685,.T.);
#3414=EDGE_CURVE('',#2747,#2749,#210,.T.);
#3415=EDGE_CURVE('',#2750,#2749,#2353,.T.);
#3416=EDGE_CURVE('',#2750,#2748,#211,.T.);
#3417=EDGE_CURVE('',#2751,#2752,#1686,.T.);
#3418=EDGE_CURVE('',#2752,#2753,#212,.T.);
#3419=EDGE_CURVE('',#2754,#2753,#2354,.T.);
#3420=EDGE_CURVE('',#2751,#2754,#213,.T.);
#3421=EDGE_CURVE('',#2755,#2756,#1687,.T.);
#3422=EDGE_CURVE('',#2756,#2752,#214,.T.);
#3423=EDGE_CURVE('',#2755,#2751,#215,.T.);
#3424=EDGE_CURVE('',#2757,#2758,#1688,.T.);
#3425=EDGE_CURVE('',#2758,#2756,#216,.T.);
#3426=EDGE_CURVE('',#2757,#2755,#217,.T.);
#3427=EDGE_CURVE('',#2759,#2760,#1689,.T.);
#3428=EDGE_CURVE('',#2760,#2758,#218,.T.);
#3429=EDGE_CURVE('',#2759,#2757,#219,.T.);
#3430=EDGE_CURVE('',#2761,#2762,#1690,.T.);
#3431=EDGE_CURVE('',#2762,#2760,#220,.T.);
#3432=EDGE_CURVE('',#2761,#2759,#221,.T.);
#3433=EDGE_CURVE('',#2763,#2764,#1691,.T.);
#3434=EDGE_CURVE('',#2764,#2762,#222,.T.);
#3435=EDGE_CURVE('',#2763,#2761,#223,.T.);
#3436=EDGE_CURVE('',#2765,#2766,#1692,.T.);
#3437=EDGE_CURVE('',#2766,#2764,#224,.T.);
#3438=EDGE_CURVE('',#2765,#2763,#225,.T.);
#3439=EDGE_CURVE('',#2767,#2768,#1693,.T.);
#3440=EDGE_CURVE('',#2769,#2767,#226,.T.);
#3441=EDGE_CURVE('',#2770,#2769,#2355,.T.);
#3442=EDGE_CURVE('',#2770,#2768,#227,.T.);
#3443=EDGE_CURVE('',#2771,#2772,#1694,.T.);
#3444=EDGE_CURVE('',#2772,#2773,#228,.T.);
#3445=EDGE_CURVE('',#2774,#2773,#2356,.T.);
#3446=EDGE_CURVE('',#2771,#2774,#229,.T.);
#3447=EDGE_CURVE('',#2775,#2776,#1695,.T.);
#3448=EDGE_CURVE('',#2776,#2772,#230,.T.);
#3449=EDGE_CURVE('',#2775,#2771,#231,.T.);
#3450=EDGE_CURVE('',#2777,#2778,#1696,.T.);
#3451=EDGE_CURVE('',#2778,#2776,#232,.T.);
#3452=EDGE_CURVE('',#2777,#2775,#233,.T.);
#3453=EDGE_CURVE('',#2779,#2780,#1697,.T.);
#3454=EDGE_CURVE('',#2780,#2778,#234,.T.);
#3455=EDGE_CURVE('',#2779,#2777,#235,.T.);
#3456=EDGE_CURVE('',#2781,#2782,#1698,.T.);
#3457=EDGE_CURVE('',#2782,#2780,#236,.T.);
#3458=EDGE_CURVE('',#2781,#2779,#237,.T.);
#3459=EDGE_CURVE('',#2783,#2784,#1699,.T.);
#3460=EDGE_CURVE('',#2784,#2782,#238,.T.);
#3461=EDGE_CURVE('',#2783,#2781,#239,.T.);
#3462=EDGE_CURVE('',#2785,#2786,#1700,.T.);
#3463=EDGE_CURVE('',#2786,#2784,#240,.T.);
#3464=EDGE_CURVE('',#2785,#2783,#241,.T.);
#3465=EDGE_CURVE('',#2787,#2788,#1701,.T.);
#3466=EDGE_CURVE('',#2789,#2787,#242,.T.);
#3467=EDGE_CURVE('',#2790,#2789,#2357,.T.);
#3468=EDGE_CURVE('',#2790,#2788,#243,.T.);
#3469=EDGE_CURVE('',#2791,#2792,#1702,.T.);
#3470=EDGE_CURVE('',#2792,#2793,#244,.T.);
#3471=EDGE_CURVE('',#2794,#2793,#2358,.T.);
#3472=EDGE_CURVE('',#2791,#2794,#245,.T.);
#3473=EDGE_CURVE('',#2795,#2796,#1703,.T.);
#3474=EDGE_CURVE('',#2796,#2792,#246,.T.);
#3475=EDGE_CURVE('',#2795,#2791,#247,.T.);
#3476=EDGE_CURVE('',#2797,#2798,#1704,.T.);
#3477=EDGE_CURVE('',#2798,#2796,#248,.T.);
#3478=EDGE_CURVE('',#2797,#2795,#249,.T.);
#3479=EDGE_CURVE('',#2799,#2800,#1705,.T.);
#3480=EDGE_CURVE('',#2800,#2798,#250,.T.);
#3481=EDGE_CURVE('',#2799,#2797,#251,.T.);
#3482=EDGE_CURVE('',#2801,#2802,#1706,.T.);
#3483=EDGE_CURVE('',#2802,#2800,#252,.T.);
#3484=EDGE_CURVE('',#2801,#2799,#253,.T.);
#3485=EDGE_CURVE('',#2803,#2804,#1707,.T.);
#3486=EDGE_CURVE('',#2804,#2802,#254,.T.);
#3487=EDGE_CURVE('',#2803,#2801,#255,.T.);
#3488=EDGE_CURVE('',#2805,#2806,#1708,.T.);
#3489=EDGE_CURVE('',#2806,#2804,#256,.T.);
#3490=EDGE_CURVE('',#2805,#2803,#257,.T.);
#3491=EDGE_CURVE('',#2807,#2808,#1709,.T.);
#3492=EDGE_CURVE('',#2809,#2807,#258,.T.);
#3493=EDGE_CURVE('',#2810,#2809,#2359,.T.);
#3494=EDGE_CURVE('',#2810,#2808,#259,.T.);
#3495=EDGE_CURVE('',#2811,#2812,#1710,.T.);
#3496=EDGE_CURVE('',#2812,#2813,#260,.T.);
#3497=EDGE_CURVE('',#2814,#2813,#2360,.T.);
#3498=EDGE_CURVE('',#2811,#2814,#261,.T.);
#3499=EDGE_CURVE('',#2815,#2816,#1711,.T.);
#3500=EDGE_CURVE('',#2816,#2812,#262,.T.);
#3501=EDGE_CURVE('',#2815,#2811,#263,.T.);
#3502=EDGE_CURVE('',#2817,#2818,#1712,.T.);
#3503=EDGE_CURVE('',#2818,#2816,#264,.T.);
#3504=EDGE_CURVE('',#2817,#2815,#265,.T.);
#3505=EDGE_CURVE('',#2819,#2820,#1713,.T.);
#3506=EDGE_CURVE('',#2820,#2818,#266,.T.);
#3507=EDGE_CURVE('',#2819,#2817,#267,.T.);
#3508=EDGE_CURVE('',#2821,#2822,#1714,.T.);
#3509=EDGE_CURVE('',#2822,#2820,#268,.T.);
#3510=EDGE_CURVE('',#2821,#2819,#269,.T.);
#3511=EDGE_CURVE('',#2823,#2824,#1715,.T.);
#3512=EDGE_CURVE('',#2824,#2822,#270,.T.);
#3513=EDGE_CURVE('',#2823,#2821,#271,.T.);
#3514=EDGE_CURVE('',#2825,#2826,#1716,.T.);
#3515=EDGE_CURVE('',#2826,#2824,#272,.T.);
#3516=EDGE_CURVE('',#2825,#2823,#273,.T.);
#3517=EDGE_CURVE('',#2827,#2828,#1717,.T.);
#3518=EDGE_CURVE('',#2829,#2827,#274,.T.);
#3519=EDGE_CURVE('',#2830,#2829,#2361,.T.);
#3520=EDGE_CURVE('',#2830,#2828,#275,.T.);
#3521=EDGE_CURVE('',#2831,#2831,#2362,.T.);
#3522=EDGE_CURVE('',#2831,#2832,#1718,.T.);
#3523=EDGE_CURVE('',#2832,#2832,#2363,.T.);
#3524=EDGE_CURVE('',#2833,#2833,#2364,.T.);
#3525=EDGE_CURVE('',#2833,#2834,#1719,.T.);
#3526=EDGE_CURVE('',#2834,#2834,#2365,.T.);
#3527=EDGE_CURVE('',#2835,#2836,#2366,.T.);
#3528=EDGE_CURVE('',#2836,#2837,#2367,.T.);
#3529=EDGE_CURVE('',#2837,#2838,#1720,.T.);
#3530=EDGE_CURVE('',#2838,#2839,#2368,.T.);
#3531=EDGE_CURVE('',#2839,#2835,#1721,.T.);
#3532=EDGE_CURVE('',#2840,#2841,#2369,.T.);
#3533=EDGE_CURVE('',#2841,#2842,#1722,.T.);
#3534=EDGE_CURVE('',#2842,#2843,#2370,.T.);
#3535=EDGE_CURVE('',#2843,#2840,#1723,.T.);
#3536=EDGE_CURVE('',#2844,#2845,#1724,.T.);
#3537=EDGE_CURVE('',#2845,#2846,#2371,.T.);
#3538=EDGE_CURVE('',#2846,#2847,#1725,.T.);
#3539=EDGE_CURVE('',#2847,#2844,#2372,.T.);
#3540=EDGE_CURVE('',#2848,#2848,#2373,.T.);
#3541=EDGE_CURVE('',#2828,#2826,#276,.T.);
#3542=EDGE_CURVE('',#2827,#2825,#277,.T.);
#3543=EDGE_CURVE('',#2813,#2674,#278,.T.);
#3544=EDGE_CURVE('',#2689,#2830,#279,.T.);
#3545=EDGE_CURVE('',#2685,#2687,#280,.T.);
#3546=EDGE_CURVE('',#2673,#2814,#281,.T.);
#3547=EDGE_CURVE('',#2688,#2686,#282,.T.);
#3548=EDGE_CURVE('',#2829,#2690,#283,.T.);
#3549=EDGE_CURVE('',#2849,#2849,#2374,.T.);
#3550=EDGE_CURVE('',#2850,#2850,#2375,.T.);
#3551=EDGE_CURVE('',#2693,#2754,#284,.T.);
#3552=EDGE_CURVE('',#2753,#2694,#285,.T.);
#3553=EDGE_CURVE('',#2713,#2774,#286,.T.);
#3554=EDGE_CURVE('',#2773,#2714,#287,.T.);
#3555=EDGE_CURVE('',#2733,#2794,#288,.T.);
#3556=EDGE_CURVE('',#2793,#2734,#289,.T.);
#3557=EDGE_CURVE('',#2808,#2806,#290,.T.);
#3558=EDGE_CURVE('',#2807,#2805,#291,.T.);
#3559=EDGE_CURVE('',#2749,#2810,#292,.T.);
#3560=EDGE_CURVE('',#2745,#2747,#293,.T.);
#3561=EDGE_CURVE('',#2748,#2746,#294,.T.);
#3562=EDGE_CURVE('',#2809,#2750,#295,.T.);
#3563=EDGE_CURVE('',#2788,#2786,#296,.T.);
#3564=EDGE_CURVE('',#2787,#2785,#297,.T.);
#3565=EDGE_CURVE('',#2729,#2790,#298,.T.);
#3566=EDGE_CURVE('',#2725,#2727,#299,.T.);
#3567=EDGE_CURVE('',#2728,#2726,#300,.T.);
#3568=EDGE_CURVE('',#2789,#2730,#301,.T.);
#3569=EDGE_CURVE('',#2768,#2766,#302,.T.);
#3570=EDGE_CURVE('',#2767,#2765,#303,.T.);
#3571=EDGE_CURVE('',#2709,#2770,#304,.T.);
#3572=EDGE_CURVE('',#2705,#2707,#305,.T.);
#3573=EDGE_CURVE('',#2708,#2706,#306,.T.);
#3574=EDGE_CURVE('',#2769,#2710,#307,.T.);
#3575=EDGE_CURVE('',#2851,#2851,#2376,.T.);
#3576=EDGE_CURVE('',#2851,#2852,#1726,.T.);
#3577=EDGE_CURVE('',#2852,#2852,#2377,.T.);
#3578=EDGE_CURVE('',#2853,#2853,#2378,.T.);
#3579=EDGE_CURVE('',#2853,#2854,#1727,.T.);
#3580=EDGE_CURVE('',#2854,#2854,#2379,.T.);
#3581=EDGE_CURVE('',#2855,#2855,#2380,.T.);
#3582=EDGE_CURVE('',#2855,#2856,#1728,.T.);
#3583=EDGE_CURVE('',#2856,#2856,#2381,.T.);
#3584=EDGE_CURVE('',#2857,#2857,#2382,.T.);
#3585=EDGE_CURVE('',#2857,#2858,#1729,.T.);
#3586=EDGE_CURVE('',#2858,#2858,#2383,.T.);
#3587=EDGE_CURVE('',#2859,#2859,#2384,.T.);
#3588=EDGE_CURVE('',#2860,#2860,#2385,.T.);
#3589=EDGE_CURVE('',#2859,#2861,#1730,.T.);
#3590=EDGE_CURVE('',#2861,#2861,#2386,.T.);
#3591=EDGE_CURVE('',#2862,#2862,#2387,.T.);
#3592=EDGE_CURVE('',#2850,#2860,#1731,.T.);
#3593=EDGE_CURVE('',#2835,#2863,#1732,.T.);
#3594=EDGE_CURVE('',#2864,#2839,#1733,.T.);
#3595=EDGE_CURVE('',#2864,#2863,#1734,.T.);
#3596=EDGE_CURVE('',#2865,#2844,#1735,.T.);
#3597=EDGE_CURVE('',#2865,#2866,#1736,.T.);
#3598=EDGE_CURVE('',#2845,#2866,#1737,.T.);
#3599=EDGE_CURVE('',#2840,#2867,#1738,.T.);
#3600=EDGE_CURVE('',#2868,#2843,#1739,.T.);
#3601=EDGE_CURVE('',#2868,#2867,#1740,.T.);
#3602=EDGE_CURVE('',#2869,#2837,#1741,.T.);
#3603=EDGE_CURVE('',#2869,#2870,#1742,.T.);
#3604=EDGE_CURVE('',#2838,#2870,#1743,.T.);
#3605=EDGE_CURVE('',#2847,#2871,#1744,.T.);
#3606=EDGE_CURVE('',#2872,#2871,#2388,.T.);
#3607=EDGE_CURVE('',#2872,#2841,#1745,.T.);
#3608=EDGE_CURVE('',#2869,#2867,#2389,.T.);
#3609=EDGE_CURVE('',#2836,#2862,#1746,.T.);
#3610=EDGE_CURVE('',#2865,#2863,#2390,.T.);
#3611=EDGE_CURVE('',#2873,#2871,#1747,.T.);
#3612=EDGE_CURVE('',#2866,#2873,#2391,.T.);
#3613=EDGE_CURVE('',#2870,#2864,#2392,.T.);
#3614=EDGE_CURVE('',#2874,#2868,#2393,.T.);
#3615=EDGE_CURVE('',#2872,#2874,#1748,.T.);
#3616=EDGE_CURVE('',#2875,#2875,#2394,.T.);
#3617=EDGE_CURVE('',#2874,#2842,#1749,.T.);
#3618=EDGE_CURVE('',#2848,#2875,#1750,.T.);
#3619=EDGE_CURVE('',#2846,#2873,#1751,.T.);
#3620=EDGE_CURVE('',#2876,#2876,#2395,.T.);
#3621=EDGE_CURVE('',#2876,#2849,#1752,.T.);
#4407=ORIENTED_EDGE('',*,*,#3313,.T.);
#4408=ORIENTED_EDGE('',*,*,#3314,.T.);
#4409=ORIENTED_EDGE('',*,*,#3315,.F.);
#4410=ORIENTED_EDGE('',*,*,#3316,.T.);
#4411=ORIENTED_EDGE('',*,*,#3317,.T.);
#4412=ORIENTED_EDGE('',*,*,#3318,.T.);
#4413=ORIENTED_EDGE('',*,*,#3313,.F.);
#4414=ORIENTED_EDGE('',*,*,#3319,.T.);
#4415=ORIENTED_EDGE('',*,*,#3320,.T.);
#4416=ORIENTED_EDGE('',*,*,#3321,.T.);
#4417=ORIENTED_EDGE('',*,*,#3317,.F.);
#4418=ORIENTED_EDGE('',*,*,#3322,.T.);
#4419=ORIENTED_EDGE('',*,*,#3323,.T.);
#4420=ORIENTED_EDGE('',*,*,#3324,.T.);
#4421=ORIENTED_EDGE('',*,*,#3320,.F.);
#4422=ORIENTED_EDGE('',*,*,#3325,.T.);
#4423=ORIENTED_EDGE('',*,*,#3326,.T.);
#4424=ORIENTED_EDGE('',*,*,#3327,.T.);
#4425=ORIENTED_EDGE('',*,*,#3323,.F.);
#4426=ORIENTED_EDGE('',*,*,#3328,.T.);
#4427=ORIENTED_EDGE('',*,*,#3329,.T.);
#4428=ORIENTED_EDGE('',*,*,#3330,.T.);
#4429=ORIENTED_EDGE('',*,*,#3326,.F.);
#4430=ORIENTED_EDGE('',*,*,#3331,.T.);
#4431=ORIENTED_EDGE('',*,*,#3332,.T.);
#4432=ORIENTED_EDGE('',*,*,#3333,.T.);
#4433=ORIENTED_EDGE('',*,*,#3329,.F.);
#4434=ORIENTED_EDGE('',*,*,#3334,.T.);
#4435=ORIENTED_EDGE('',*,*,#3335,.F.);
#4436=ORIENTED_EDGE('',*,*,#3336,.T.);
#4437=ORIENTED_EDGE('',*,*,#3337,.F.);
#4438=ORIENTED_EDGE('',*,*,#3338,.T.);
#4439=ORIENTED_EDGE('',*,*,#3339,.T.);
#4440=ORIENTED_EDGE('',*,*,#3340,.T.);
#4441=ORIENTED_EDGE('',*,*,#3341,.F.);
#4442=ORIENTED_EDGE('',*,*,#3342,.T.);
#4443=ORIENTED_EDGE('',*,*,#3343,.T.);
#4444=ORIENTED_EDGE('',*,*,#3344,.T.);
#4445=ORIENTED_EDGE('',*,*,#3339,.F.);
#4446=ORIENTED_EDGE('',*,*,#3345,.T.);
#4447=ORIENTED_EDGE('',*,*,#3346,.T.);
#4448=ORIENTED_EDGE('',*,*,#3347,.T.);
#4449=ORIENTED_EDGE('',*,*,#3343,.F.);
#4450=ORIENTED_EDGE('',*,*,#3348,.T.);
#4451=ORIENTED_EDGE('',*,*,#3349,.T.);
#4452=ORIENTED_EDGE('',*,*,#3350,.T.);
#4453=ORIENTED_EDGE('',*,*,#3346,.F.);
#4454=ORIENTED_EDGE('',*,*,#3351,.T.);
#4455=ORIENTED_EDGE('',*,*,#3352,.T.);
#4456=ORIENTED_EDGE('',*,*,#3353,.T.);
#4457=ORIENTED_EDGE('',*,*,#3349,.F.);
#4458=ORIENTED_EDGE('',*,*,#3354,.T.);
#4459=ORIENTED_EDGE('',*,*,#3355,.T.);
#4460=ORIENTED_EDGE('',*,*,#3356,.T.);
#4461=ORIENTED_EDGE('',*,*,#3352,.F.);
#4462=ORIENTED_EDGE('',*,*,#3357,.T.);
#4463=ORIENTED_EDGE('',*,*,#3358,.T.);
#4464=ORIENTED_EDGE('',*,*,#3359,.T.);
#4465=ORIENTED_EDGE('',*,*,#3355,.F.);
#4466=ORIENTED_EDGE('',*,*,#3360,.T.);
#4467=ORIENTED_EDGE('',*,*,#3361,.F.);
#4468=ORIENTED_EDGE('',*,*,#3362,.T.);
#4469=ORIENTED_EDGE('',*,*,#3363,.F.);
#4470=ORIENTED_EDGE('',*,*,#3364,.T.);
#4471=ORIENTED_EDGE('',*,*,#3365,.T.);
#4472=ORIENTED_EDGE('',*,*,#3366,.T.);
#4473=ORIENTED_EDGE('',*,*,#3367,.F.);
#4474=ORIENTED_EDGE('',*,*,#3368,.T.);
#4475=ORIENTED_EDGE('',*,*,#3369,.T.);
#4476=ORIENTED_EDGE('',*,*,#3370,.T.);
#4477=ORIENTED_EDGE('',*,*,#3365,.F.);
#4478=ORIENTED_EDGE('',*,*,#3371,.T.);
#4479=ORIENTED_EDGE('',*,*,#3372,.T.);
#4480=ORIENTED_EDGE('',*,*,#3373,.T.);
#4481=ORIENTED_EDGE('',*,*,#3369,.F.);
#4482=ORIENTED_EDGE('',*,*,#3374,.T.);
#4483=ORIENTED_EDGE('',*,*,#3375,.T.);
#4484=ORIENTED_EDGE('',*,*,#3376,.T.);
#4485=ORIENTED_EDGE('',*,*,#3372,.F.);
#4486=ORIENTED_EDGE('',*,*,#3377,.T.);
#4487=ORIENTED_EDGE('',*,*,#3378,.T.);
#4488=ORIENTED_EDGE('',*,*,#3379,.T.);
#4489=ORIENTED_EDGE('',*,*,#3375,.F.);
#4490=ORIENTED_EDGE('',*,*,#3380,.T.);
#4491=ORIENTED_EDGE('',*,*,#3381,.T.);
#4492=ORIENTED_EDGE('',*,*,#3382,.T.);
#4493=ORIENTED_EDGE('',*,*,#3378,.F.);
#4494=ORIENTED_EDGE('',*,*,#3383,.T.);
#4495=ORIENTED_EDGE('',*,*,#3384,.T.);
#4496=ORIENTED_EDGE('',*,*,#3385,.T.);
#4497=ORIENTED_EDGE('',*,*,#3381,.F.);
#4498=ORIENTED_EDGE('',*,*,#3386,.T.);
#4499=ORIENTED_EDGE('',*,*,#3387,.F.);
#4500=ORIENTED_EDGE('',*,*,#3388,.T.);
#4501=ORIENTED_EDGE('',*,*,#3389,.F.);
#4502=ORIENTED_EDGE('',*,*,#3390,.T.);
#4503=ORIENTED_EDGE('',*,*,#3391,.T.);
#4504=ORIENTED_EDGE('',*,*,#3392,.T.);
#4505=ORIENTED_EDGE('',*,*,#3393,.F.);
#4506=ORIENTED_EDGE('',*,*,#3394,.T.);
#4507=ORIENTED_EDGE('',*,*,#3395,.T.);
#4508=ORIENTED_EDGE('',*,*,#3396,.T.);
#4509=ORIENTED_EDGE('',*,*,#3391,.F.);
#4510=ORIENTED_EDGE('',*,*,#3397,.T.);
#4511=ORIENTED_EDGE('',*,*,#3398,.T.);
#4512=ORIENTED_EDGE('',*,*,#3399,.T.);
#4513=ORIENTED_EDGE('',*,*,#3395,.F.);
#4514=ORIENTED_EDGE('',*,*,#3400,.T.);
#4515=ORIENTED_EDGE('',*,*,#3401,.T.);
#4516=ORIENTED_EDGE('',*,*,#3402,.T.);
#4517=ORIENTED_EDGE('',*,*,#3398,.F.);
#4518=ORIENTED_EDGE('',*,*,#3403,.T.);
#4519=ORIENTED_EDGE('',*,*,#3404,.T.);
#4520=ORIENTED_EDGE('',*,*,#3405,.T.);
#4521=ORIENTED_EDGE('',*,*,#3401,.F.);
#4522=ORIENTED_EDGE('',*,*,#3406,.T.);
#4523=ORIENTED_EDGE('',*,*,#3407,.T.);
#4524=ORIENTED_EDGE('',*,*,#3408,.T.);
#4525=ORIENTED_EDGE('',*,*,#3404,.F.);
#4526=ORIENTED_EDGE('',*,*,#3409,.T.);
#4527=ORIENTED_EDGE('',*,*,#3410,.T.);
#4528=ORIENTED_EDGE('',*,*,#3411,.T.);
#4529=ORIENTED_EDGE('',*,*,#3407,.F.);
#4530=ORIENTED_EDGE('',*,*,#3412,.T.);
#4531=ORIENTED_EDGE('',*,*,#3413,.F.);
#4532=ORIENTED_EDGE('',*,*,#3414,.T.);
#4533=ORIENTED_EDGE('',*,*,#3415,.F.);
#4534=ORIENTED_EDGE('',*,*,#3416,.T.);
#4535=ORIENTED_EDGE('',*,*,#3417,.T.);
#4536=ORIENTED_EDGE('',*,*,#3418,.T.);
#4537=ORIENTED_EDGE('',*,*,#3419,.F.);
#4538=ORIENTED_EDGE('',*,*,#3420,.F.);
#4539=ORIENTED_EDGE('',*,*,#3421,.T.);
#4540=ORIENTED_EDGE('',*,*,#3422,.T.);
#4541=ORIENTED_EDGE('',*,*,#3417,.F.);
#4542=ORIENTED_EDGE('',*,*,#3423,.F.);
#4543=ORIENTED_EDGE('',*,*,#3424,.T.);
#4544=ORIENTED_EDGE('',*,*,#3425,.T.);
#4545=ORIENTED_EDGE('',*,*,#3421,.F.);
#4546=ORIENTED_EDGE('',*,*,#3426,.F.);
#4547=ORIENTED_EDGE('',*,*,#3427,.T.);
#4548=ORIENTED_EDGE('',*,*,#3428,.T.);
#4549=ORIENTED_EDGE('',*,*,#3424,.F.);
#4550=ORIENTED_EDGE('',*,*,#3429,.F.);
#4551=ORIENTED_EDGE('',*,*,#3430,.T.);
#4552=ORIENTED_EDGE('',*,*,#3431,.T.);
#4553=ORIENTED_EDGE('',*,*,#3427,.F.);
#4554=ORIENTED_EDGE('',*,*,#3432,.F.);
#4555=ORIENTED_EDGE('',*,*,#3433,.T.);
#4556=ORIENTED_EDGE('',*,*,#3434,.T.);
#4557=ORIENTED_EDGE('',*,*,#3430,.F.);
#4558=ORIENTED_EDGE('',*,*,#3435,.F.);
#4559=ORIENTED_EDGE('',*,*,#3436,.T.);
#4560=ORIENTED_EDGE('',*,*,#3437,.T.);
#4561=ORIENTED_EDGE('',*,*,#3433,.F.);
#4562=ORIENTED_EDGE('',*,*,#3438,.F.);
#4563=ORIENTED_EDGE('',*,*,#3439,.F.);
#4564=ORIENTED_EDGE('',*,*,#3440,.F.);
#4565=ORIENTED_EDGE('',*,*,#3441,.F.);
#4566=ORIENTED_EDGE('',*,*,#3442,.T.);
#4567=ORIENTED_EDGE('',*,*,#3443,.T.);
#4568=ORIENTED_EDGE('',*,*,#3444,.T.);
#4569=ORIENTED_EDGE('',*,*,#3445,.F.);
#4570=ORIENTED_EDGE('',*,*,#3446,.F.);
#4571=ORIENTED_EDGE('',*,*,#3447,.T.);
#4572=ORIENTED_EDGE('',*,*,#3448,.T.);
#4573=ORIENTED_EDGE('',*,*,#3443,.F.);
#4574=ORIENTED_EDGE('',*,*,#3449,.F.);
#4575=ORIENTED_EDGE('',*,*,#3450,.T.);
#4576=ORIENTED_EDGE('',*,*,#3451,.T.);
#4577=ORIENTED_EDGE('',*,*,#3447,.F.);
#4578=ORIENTED_EDGE('',*,*,#3452,.F.);
#4579=ORIENTED_EDGE('',*,*,#3453,.T.);
#4580=ORIENTED_EDGE('',*,*,#3454,.T.);
#4581=ORIENTED_EDGE('',*,*,#3450,.F.);
#4582=ORIENTED_EDGE('',*,*,#3455,.F.);
#4583=ORIENTED_EDGE('',*,*,#3456,.T.);
#4584=ORIENTED_EDGE('',*,*,#3457,.T.);
#4585=ORIENTED_EDGE('',*,*,#3453,.F.);
#4586=ORIENTED_EDGE('',*,*,#3458,.F.);
#4587=ORIENTED_EDGE('',*,*,#3459,.T.);
#4588=ORIENTED_EDGE('',*,*,#3460,.T.);
#4589=ORIENTED_EDGE('',*,*,#3456,.F.);
#4590=ORIENTED_EDGE('',*,*,#3461,.F.);
#4591=ORIENTED_EDGE('',*,*,#3462,.T.);
#4592=ORIENTED_EDGE('',*,*,#3463,.T.);
#4593=ORIENTED_EDGE('',*,*,#3459,.F.);
#4594=ORIENTED_EDGE('',*,*,#3464,.F.);
#4595=ORIENTED_EDGE('',*,*,#3465,.F.);
#4596=ORIENTED_EDGE('',*,*,#3466,.F.);
#4597=ORIENTED_EDGE('',*,*,#3467,.F.);
#4598=ORIENTED_EDGE('',*,*,#3468,.T.);
#4599=ORIENTED_EDGE('',*,*,#3469,.T.);
#4600=ORIENTED_EDGE('',*,*,#3470,.T.);
#4601=ORIENTED_EDGE('',*,*,#3471,.F.);
#4602=ORIENTED_EDGE('',*,*,#3472,.F.);
#4603=ORIENTED_EDGE('',*,*,#3473,.T.);
#4604=ORIENTED_EDGE('',*,*,#3474,.T.);
#4605=ORIENTED_EDGE('',*,*,#3469,.F.);
#4606=ORIENTED_EDGE('',*,*,#3475,.F.);
#4607=ORIENTED_EDGE('',*,*,#3476,.T.);
#4608=ORIENTED_EDGE('',*,*,#3477,.T.);
#4609=ORIENTED_EDGE('',*,*,#3473,.F.);
#4610=ORIENTED_EDGE('',*,*,#3478,.F.);
#4611=ORIENTED_EDGE('',*,*,#3479,.T.);
#4612=ORIENTED_EDGE('',*,*,#3480,.T.);
#4613=ORIENTED_EDGE('',*,*,#3476,.F.);
#4614=ORIENTED_EDGE('',*,*,#3481,.F.);
#4615=ORIENTED_EDGE('',*,*,#3482,.T.);
#4616=ORIENTED_EDGE('',*,*,#3483,.T.);
#4617=ORIENTED_EDGE('',*,*,#3479,.F.);
#4618=ORIENTED_EDGE('',*,*,#3484,.F.);
#4619=ORIENTED_EDGE('',*,*,#3485,.T.);
#4620=ORIENTED_EDGE('',*,*,#3486,.T.);
#4621=ORIENTED_EDGE('',*,*,#3482,.F.);
#4622=ORIENTED_EDGE('',*,*,#3487,.F.);
#4623=ORIENTED_EDGE('',*,*,#3488,.T.);
#4624=ORIENTED_EDGE('',*,*,#3489,.T.);
#4625=ORIENTED_EDGE('',*,*,#3485,.F.);
#4626=ORIENTED_EDGE('',*,*,#3490,.F.);
#4627=ORIENTED_EDGE('',*,*,#3491,.F.);
#4628=ORIENTED_EDGE('',*,*,#3492,.F.);
#4629=ORIENTED_EDGE('',*,*,#3493,.F.);
#4630=ORIENTED_EDGE('',*,*,#3494,.T.);
#4631=ORIENTED_EDGE('',*,*,#3495,.T.);
#4632=ORIENTED_EDGE('',*,*,#3496,.T.);
#4633=ORIENTED_EDGE('',*,*,#3497,.F.);
#4634=ORIENTED_EDGE('',*,*,#3498,.F.);
#4635=ORIENTED_EDGE('',*,*,#3499,.T.);
#4636=ORIENTED_EDGE('',*,*,#3500,.T.);
#4637=ORIENTED_EDGE('',*,*,#3495,.F.);
#4638=ORIENTED_EDGE('',*,*,#3501,.F.);
#4639=ORIENTED_EDGE('',*,*,#3502,.T.);
#4640=ORIENTED_EDGE('',*,*,#3503,.T.);
#4641=ORIENTED_EDGE('',*,*,#3499,.F.);
#4642=ORIENTED_EDGE('',*,*,#3504,.F.);
#4643=ORIENTED_EDGE('',*,*,#3505,.T.);
#4644=ORIENTED_EDGE('',*,*,#3506,.T.);
#4645=ORIENTED_EDGE('',*,*,#3502,.F.);
#4646=ORIENTED_EDGE('',*,*,#3507,.F.);
#4647=ORIENTED_EDGE('',*,*,#3508,.T.);
#4648=ORIENTED_EDGE('',*,*,#3509,.T.);
#4649=ORIENTED_EDGE('',*,*,#3505,.F.);
#4650=ORIENTED_EDGE('',*,*,#3510,.F.);
#4651=ORIENTED_EDGE('',*,*,#3511,.T.);
#4652=ORIENTED_EDGE('',*,*,#3512,.T.);
#4653=ORIENTED_EDGE('',*,*,#3508,.F.);
#4654=ORIENTED_EDGE('',*,*,#3513,.F.);
#4655=ORIENTED_EDGE('',*,*,#3514,.T.);
#4656=ORIENTED_EDGE('',*,*,#3515,.T.);
#4657=ORIENTED_EDGE('',*,*,#3511,.F.);
#4658=ORIENTED_EDGE('',*,*,#3516,.F.);
#4659=ORIENTED_EDGE('',*,*,#3517,.F.);
#4660=ORIENTED_EDGE('',*,*,#3518,.F.);
#4661=ORIENTED_EDGE('',*,*,#3519,.F.);
#4662=ORIENTED_EDGE('',*,*,#3520,.T.);
#4663=ORIENTED_EDGE('',*,*,#3521,.F.);
#4664=ORIENTED_EDGE('',*,*,#3522,.T.);
#4665=ORIENTED_EDGE('',*,*,#3523,.T.);
#4666=ORIENTED_EDGE('',*,*,#3522,.F.);
#4667=ORIENTED_EDGE('',*,*,#3524,.F.);
#4668=ORIENTED_EDGE('',*,*,#3525,.T.);
#4669=ORIENTED_EDGE('',*,*,#3526,.T.);
#4670=ORIENTED_EDGE('',*,*,#3525,.F.);
#4671=ORIENTED_EDGE('',*,*,#3526,.F.);
#4672=ORIENTED_EDGE('',*,*,#3523,.F.);
#4673=ORIENTED_EDGE('',*,*,#3521,.T.);
#4674=ORIENTED_EDGE('',*,*,#3527,.T.);
#4675=ORIENTED_EDGE('',*,*,#3528,.T.);
#4676=ORIENTED_EDGE('',*,*,#3529,.T.);
#4677=ORIENTED_EDGE('',*,*,#3530,.T.);
#4678=ORIENTED_EDGE('',*,*,#3531,.T.);
#4679=ORIENTED_EDGE('',*,*,#3532,.T.);
#4680=ORIENTED_EDGE('',*,*,#3533,.T.);
#4681=ORIENTED_EDGE('',*,*,#3534,.T.);
#4682=ORIENTED_EDGE('',*,*,#3535,.T.);
#4683=ORIENTED_EDGE('',*,*,#3536,.T.);
#4684=ORIENTED_EDGE('',*,*,#3537,.T.);
#4685=ORIENTED_EDGE('',*,*,#3538,.T.);
#4686=ORIENTED_EDGE('',*,*,#3539,.T.);
#4687=ORIENTED_EDGE('',*,*,#3540,.T.);
#4688=ORIENTED_EDGE('',*,*,#3517,.T.);
#4689=ORIENTED_EDGE('',*,*,#3541,.T.);
#4690=ORIENTED_EDGE('',*,*,#3514,.F.);
#4691=ORIENTED_EDGE('',*,*,#3542,.F.);
#4692=ORIENTED_EDGE('',*,*,#3543,.F.);
#4693=ORIENTED_EDGE('',*,*,#3496,.F.);
#4694=ORIENTED_EDGE('',*,*,#3500,.F.);
#4695=ORIENTED_EDGE('',*,*,#3503,.F.);
#4696=ORIENTED_EDGE('',*,*,#3506,.F.);
#4697=ORIENTED_EDGE('',*,*,#3509,.F.);
#4698=ORIENTED_EDGE('',*,*,#3512,.F.);
#4699=ORIENTED_EDGE('',*,*,#3515,.F.);
#4700=ORIENTED_EDGE('',*,*,#3541,.F.);
#4701=ORIENTED_EDGE('',*,*,#3520,.F.);
#4702=ORIENTED_EDGE('',*,*,#3544,.F.);
#4703=ORIENTED_EDGE('',*,*,#3336,.F.);
#4704=ORIENTED_EDGE('',*,*,#3545,.F.);
#4705=ORIENTED_EDGE('',*,*,#3334,.F.);
#4706=ORIENTED_EDGE('',*,*,#3331,.F.);
#4707=ORIENTED_EDGE('',*,*,#3328,.F.);
#4708=ORIENTED_EDGE('',*,*,#3325,.F.);
#4709=ORIENTED_EDGE('',*,*,#3322,.F.);
#4710=ORIENTED_EDGE('',*,*,#3319,.F.);
#4711=ORIENTED_EDGE('',*,*,#3316,.F.);
#4712=ORIENTED_EDGE('',*,*,#3546,.F.);
#4713=ORIENTED_EDGE('',*,*,#3314,.F.);
#4714=ORIENTED_EDGE('',*,*,#3318,.F.);
#4715=ORIENTED_EDGE('',*,*,#3321,.F.);
#4716=ORIENTED_EDGE('',*,*,#3324,.F.);
#4717=ORIENTED_EDGE('',*,*,#3327,.F.);
#4718=ORIENTED_EDGE('',*,*,#3330,.F.);
#4719=ORIENTED_EDGE('',*,*,#3333,.F.);
#4720=ORIENTED_EDGE('',*,*,#3547,.F.);
#4721=ORIENTED_EDGE('',*,*,#3338,.F.);
#4722=ORIENTED_EDGE('',*,*,#3548,.F.);
#4723=ORIENTED_EDGE('',*,*,#3518,.T.);
#4724=ORIENTED_EDGE('',*,*,#3542,.T.);
#4725=ORIENTED_EDGE('',*,*,#3516,.T.);
#4726=ORIENTED_EDGE('',*,*,#3513,.T.);
#4727=ORIENTED_EDGE('',*,*,#3510,.T.);
#4728=ORIENTED_EDGE('',*,*,#3507,.T.);
#4729=ORIENTED_EDGE('',*,*,#3504,.T.);
#4730=ORIENTED_EDGE('',*,*,#3501,.T.);
#4731=ORIENTED_EDGE('',*,*,#3498,.T.);
#4732=ORIENTED_EDGE('',*,*,#3549,.F.);
#4733=ORIENTED_EDGE('',*,*,#3550,.T.);
#4734=ORIENTED_EDGE('',*,*,#3546,.T.);
#4735=ORIENTED_EDGE('',*,*,#3497,.T.);
#4736=ORIENTED_EDGE('',*,*,#3543,.T.);
#4737=ORIENTED_EDGE('',*,*,#3315,.T.);
#4738=ORIENTED_EDGE('',*,*,#3551,.T.);
#4739=ORIENTED_EDGE('',*,*,#3419,.T.);
#4740=ORIENTED_EDGE('',*,*,#3552,.T.);
#4741=ORIENTED_EDGE('',*,*,#3341,.T.);
#4742=ORIENTED_EDGE('',*,*,#3553,.T.);
#4743=ORIENTED_EDGE('',*,*,#3445,.T.);
#4744=ORIENTED_EDGE('',*,*,#3554,.T.);
#4745=ORIENTED_EDGE('',*,*,#3367,.T.);
#4746=ORIENTED_EDGE('',*,*,#3555,.T.);
#4747=ORIENTED_EDGE('',*,*,#3471,.T.);
#4748=ORIENTED_EDGE('',*,*,#3556,.T.);
#4749=ORIENTED_EDGE('',*,*,#3393,.T.);
#4750=ORIENTED_EDGE('',*,*,#3491,.T.);
#4751=ORIENTED_EDGE('',*,*,#3557,.T.);
#4752=ORIENTED_EDGE('',*,*,#3488,.F.);
#4753=ORIENTED_EDGE('',*,*,#3558,.F.);
#4754=ORIENTED_EDGE('',*,*,#3556,.F.);
#4755=ORIENTED_EDGE('',*,*,#3470,.F.);
#4756=ORIENTED_EDGE('',*,*,#3474,.F.);
#4757=ORIENTED_EDGE('',*,*,#3477,.F.);
#4758=ORIENTED_EDGE('',*,*,#3480,.F.);
#4759=ORIENTED_EDGE('',*,*,#3483,.F.);
#4760=ORIENTED_EDGE('',*,*,#3486,.F.);
#4761=ORIENTED_EDGE('',*,*,#3489,.F.);
#4762=ORIENTED_EDGE('',*,*,#3557,.F.);
#4763=ORIENTED_EDGE('',*,*,#3494,.F.);
#4764=ORIENTED_EDGE('',*,*,#3559,.F.);
#4765=ORIENTED_EDGE('',*,*,#3414,.F.);
#4766=ORIENTED_EDGE('',*,*,#3560,.F.);
#4767=ORIENTED_EDGE('',*,*,#3412,.F.);
#4768=ORIENTED_EDGE('',*,*,#3409,.F.);
#4769=ORIENTED_EDGE('',*,*,#3406,.F.);
#4770=ORIENTED_EDGE('',*,*,#3403,.F.);
#4771=ORIENTED_EDGE('',*,*,#3400,.F.);
#4772=ORIENTED_EDGE('',*,*,#3397,.F.);
#4773=ORIENTED_EDGE('',*,*,#3394,.F.);
#4774=ORIENTED_EDGE('',*,*,#3555,.F.);
#4775=ORIENTED_EDGE('',*,*,#3392,.F.);
#4776=ORIENTED_EDGE('',*,*,#3396,.F.);
#4777=ORIENTED_EDGE('',*,*,#3399,.F.);
#4778=ORIENTED_EDGE('',*,*,#3402,.F.);
#4779=ORIENTED_EDGE('',*,*,#3405,.F.);
#4780=ORIENTED_EDGE('',*,*,#3408,.F.);
#4781=ORIENTED_EDGE('',*,*,#3411,.F.);
#4782=ORIENTED_EDGE('',*,*,#3561,.F.);
#4783=ORIENTED_EDGE('',*,*,#3416,.F.);
#4784=ORIENTED_EDGE('',*,*,#3562,.F.);
#4785=ORIENTED_EDGE('',*,*,#3492,.T.);
#4786=ORIENTED_EDGE('',*,*,#3558,.T.);
#4787=ORIENTED_EDGE('',*,*,#3490,.T.);
#4788=ORIENTED_EDGE('',*,*,#3487,.T.);
#4789=ORIENTED_EDGE('',*,*,#3484,.T.);
#4790=ORIENTED_EDGE('',*,*,#3481,.T.);
#4791=ORIENTED_EDGE('',*,*,#3478,.T.);
#4792=ORIENTED_EDGE('',*,*,#3475,.T.);
#4793=ORIENTED_EDGE('',*,*,#3472,.T.);
#4794=ORIENTED_EDGE('',*,*,#3465,.T.);
#4795=ORIENTED_EDGE('',*,*,#3563,.T.);
#4796=ORIENTED_EDGE('',*,*,#3462,.F.);
#4797=ORIENTED_EDGE('',*,*,#3564,.F.);
#4798=ORIENTED_EDGE('',*,*,#3554,.F.);
#4799=ORIENTED_EDGE('',*,*,#3444,.F.);
#4800=ORIENTED_EDGE('',*,*,#3448,.F.);
#4801=ORIENTED_EDGE('',*,*,#3451,.F.);
#4802=ORIENTED_EDGE('',*,*,#3454,.F.);
#4803=ORIENTED_EDGE('',*,*,#3457,.F.);
#4804=ORIENTED_EDGE('',*,*,#3460,.F.);
#4805=ORIENTED_EDGE('',*,*,#3463,.F.);
#4806=ORIENTED_EDGE('',*,*,#3563,.F.);
#4807=ORIENTED_EDGE('',*,*,#3468,.F.);
#4808=ORIENTED_EDGE('',*,*,#3565,.F.);
#4809=ORIENTED_EDGE('',*,*,#3388,.F.);
#4810=ORIENTED_EDGE('',*,*,#3566,.F.);
#4811=ORIENTED_EDGE('',*,*,#3386,.F.);
#4812=ORIENTED_EDGE('',*,*,#3383,.F.);
#4813=ORIENTED_EDGE('',*,*,#3380,.F.);
#4814=ORIENTED_EDGE('',*,*,#3377,.F.);
#4815=ORIENTED_EDGE('',*,*,#3374,.F.);
#4816=ORIENTED_EDGE('',*,*,#3371,.F.);
#4817=ORIENTED_EDGE('',*,*,#3368,.F.);
#4818=ORIENTED_EDGE('',*,*,#3553,.F.);
#4819=ORIENTED_EDGE('',*,*,#3366,.F.);
#4820=ORIENTED_EDGE('',*,*,#3370,.F.);
#4821=ORIENTED_EDGE('',*,*,#3373,.F.);
#4822=ORIENTED_EDGE('',*,*,#3376,.F.);
#4823=ORIENTED_EDGE('',*,*,#3379,.F.);
#4824=ORIENTED_EDGE('',*,*,#3382,.F.);
#4825=ORIENTED_EDGE('',*,*,#3385,.F.);
#4826=ORIENTED_EDGE('',*,*,#3567,.F.);
#4827=ORIENTED_EDGE('',*,*,#3390,.F.);
#4828=ORIENTED_EDGE('',*,*,#3568,.F.);
#4829=ORIENTED_EDGE('',*,*,#3466,.T.);
#4830=ORIENTED_EDGE('',*,*,#3564,.T.);
#4831=ORIENTED_EDGE('',*,*,#3464,.T.);
#4832=ORIENTED_EDGE('',*,*,#3461,.T.);
#4833=ORIENTED_EDGE('',*,*,#3458,.T.);
#4834=ORIENTED_EDGE('',*,*,#3455,.T.);
#4835=ORIENTED_EDGE('',*,*,#3452,.T.);
#4836=ORIENTED_EDGE('',*,*,#3449,.T.);
#4837=ORIENTED_EDGE('',*,*,#3446,.T.);
#4838=ORIENTED_EDGE('',*,*,#3439,.T.);
#4839=ORIENTED_EDGE('',*,*,#3569,.T.);
#4840=ORIENTED_EDGE('',*,*,#3436,.F.);
#4841=ORIENTED_EDGE('',*,*,#3570,.F.);
#4842=ORIENTED_EDGE('',*,*,#3552,.F.);
#4843=ORIENTED_EDGE('',*,*,#3418,.F.);
#4844=ORIENTED_EDGE('',*,*,#3422,.F.);
#4845=ORIENTED_EDGE('',*,*,#3425,.F.);
#4846=ORIENTED_EDGE('',*,*,#3428,.F.);
#4847=ORIENTED_EDGE('',*,*,#3431,.F.);
#4848=ORIENTED_EDGE('',*,*,#3434,.F.);
#4849=ORIENTED_EDGE('',*,*,#3437,.F.);
#4850=ORIENTED_EDGE('',*,*,#3569,.F.);
#4851=ORIENTED_EDGE('',*,*,#3442,.F.);
#4852=ORIENTED_EDGE('',*,*,#3571,.F.);
#4853=ORIENTED_EDGE('',*,*,#3362,.F.);
#4854=ORIENTED_EDGE('',*,*,#3572,.F.);
#4855=ORIENTED_EDGE('',*,*,#3360,.F.);
#4856=ORIENTED_EDGE('',*,*,#3357,.F.);
#4857=ORIENTED_EDGE('',*,*,#3354,.F.);
#4858=ORIENTED_EDGE('',*,*,#3351,.F.);
#4859=ORIENTED_EDGE('',*,*,#3348,.F.);
#4860=ORIENTED_EDGE('',*,*,#3345,.F.);
#4861=ORIENTED_EDGE('',*,*,#3342,.F.);
#4862=ORIENTED_EDGE('',*,*,#3551,.F.);
#4863=ORIENTED_EDGE('',*,*,#3340,.F.);
#4864=ORIENTED_EDGE('',*,*,#3344,.F.);
#4865=ORIENTED_EDGE('',*,*,#3347,.F.);
#4866=ORIENTED_EDGE('',*,*,#3350,.F.);
#4867=ORIENTED_EDGE('',*,*,#3353,.F.);
#4868=ORIENTED_EDGE('',*,*,#3356,.F.);
#4869=ORIENTED_EDGE('',*,*,#3359,.F.);
#4870=ORIENTED_EDGE('',*,*,#3573,.F.);
#4871=ORIENTED_EDGE('',*,*,#3364,.F.);
#4872=ORIENTED_EDGE('',*,*,#3574,.F.);
#4873=ORIENTED_EDGE('',*,*,#3440,.T.);
#4874=ORIENTED_EDGE('',*,*,#3570,.T.);
#4875=ORIENTED_EDGE('',*,*,#3438,.T.);
#4876=ORIENTED_EDGE('',*,*,#3435,.T.);
#4877=ORIENTED_EDGE('',*,*,#3432,.T.);
#4878=ORIENTED_EDGE('',*,*,#3429,.T.);
#4879=ORIENTED_EDGE('',*,*,#3426,.T.);
#4880=ORIENTED_EDGE('',*,*,#3423,.T.);
#4881=ORIENTED_EDGE('',*,*,#3420,.T.);
#4882=ORIENTED_EDGE('',*,*,#3413,.T.);
#4883=ORIENTED_EDGE('',*,*,#3561,.T.);
#4884=ORIENTED_EDGE('',*,*,#3410,.F.);
#4885=ORIENTED_EDGE('',*,*,#3560,.T.);
#4886=ORIENTED_EDGE('',*,*,#3387,.T.);
#4887=ORIENTED_EDGE('',*,*,#3567,.T.);
#4888=ORIENTED_EDGE('',*,*,#3384,.F.);
#4889=ORIENTED_EDGE('',*,*,#3566,.T.);
#4890=ORIENTED_EDGE('',*,*,#3361,.T.);
#4891=ORIENTED_EDGE('',*,*,#3573,.T.);
#4892=ORIENTED_EDGE('',*,*,#3358,.F.);
#4893=ORIENTED_EDGE('',*,*,#3572,.T.);
#4894=ORIENTED_EDGE('',*,*,#3335,.T.);
#4895=ORIENTED_EDGE('',*,*,#3547,.T.);
#4896=ORIENTED_EDGE('',*,*,#3332,.F.);
#4897=ORIENTED_EDGE('',*,*,#3545,.T.);
#4898=ORIENTED_EDGE('',*,*,#3575,.F.);
#4899=ORIENTED_EDGE('',*,*,#3576,.T.);
#4900=ORIENTED_EDGE('',*,*,#3577,.F.);
#4901=ORIENTED_EDGE('',*,*,#3576,.F.);
#4902=ORIENTED_EDGE('',*,*,#3578,.F.);
#4903=ORIENTED_EDGE('',*,*,#3579,.T.);
#4904=ORIENTED_EDGE('',*,*,#3580,.F.);
#4905=ORIENTED_EDGE('',*,*,#3579,.F.);
#4906=ORIENTED_EDGE('',*,*,#3581,.F.);
#4907=ORIENTED_EDGE('',*,*,#3582,.T.);
#4908=ORIENTED_EDGE('',*,*,#3583,.F.);
#4909=ORIENTED_EDGE('',*,*,#3582,.F.);
#4910=ORIENTED_EDGE('',*,*,#3584,.F.);
#4911=ORIENTED_EDGE('',*,*,#3585,.T.);
#4912=ORIENTED_EDGE('',*,*,#3586,.F.);
#4913=ORIENTED_EDGE('',*,*,#3585,.F.);
#4914=ORIENTED_EDGE('',*,*,#3587,.T.);
#4915=ORIENTED_EDGE('',*,*,#3588,.F.);
#4916=ORIENTED_EDGE('',*,*,#3584,.T.);
#4917=ORIENTED_EDGE('',*,*,#3581,.T.);
#4918=ORIENTED_EDGE('',*,*,#3578,.T.);
#4919=ORIENTED_EDGE('',*,*,#3575,.T.);
#4920=ORIENTED_EDGE('',*,*,#3587,.F.);
#4921=ORIENTED_EDGE('',*,*,#3589,.T.);
#4922=ORIENTED_EDGE('',*,*,#3590,.T.);
#4923=ORIENTED_EDGE('',*,*,#3589,.F.);
#4924=ORIENTED_EDGE('',*,*,#3590,.F.);
#4925=ORIENTED_EDGE('',*,*,#3591,.F.);
#4926=ORIENTED_EDGE('',*,*,#3586,.T.);
#4927=ORIENTED_EDGE('',*,*,#3583,.T.);
#4928=ORIENTED_EDGE('',*,*,#3580,.T.);
#4929=ORIENTED_EDGE('',*,*,#3577,.T.);
#4930=ORIENTED_EDGE('',*,*,#3550,.F.);
#4931=ORIENTED_EDGE('',*,*,#3592,.T.);
#4932=ORIENTED_EDGE('',*,*,#3588,.T.);
#4933=ORIENTED_EDGE('',*,*,#3592,.F.);
#4934=ORIENTED_EDGE('',*,*,#3593,.F.);
#4935=ORIENTED_EDGE('',*,*,#3531,.F.);
#4936=ORIENTED_EDGE('',*,*,#3594,.F.);
#4937=ORIENTED_EDGE('',*,*,#3595,.T.);
#4938=ORIENTED_EDGE('',*,*,#3596,.F.);
#4939=ORIENTED_EDGE('',*,*,#3597,.T.);
#4940=ORIENTED_EDGE('',*,*,#3598,.F.);
#4941=ORIENTED_EDGE('',*,*,#3536,.F.);
#4942=ORIENTED_EDGE('',*,*,#3599,.F.);
#4943=ORIENTED_EDGE('',*,*,#3535,.F.);
#4944=ORIENTED_EDGE('',*,*,#3600,.F.);
#4945=ORIENTED_EDGE('',*,*,#3601,.T.);
#4946=ORIENTED_EDGE('',*,*,#3602,.F.);
#4947=ORIENTED_EDGE('',*,*,#3603,.T.);
#4948=ORIENTED_EDGE('',*,*,#3604,.F.);
#4949=ORIENTED_EDGE('',*,*,#3529,.F.);
#4950=ORIENTED_EDGE('',*,*,#3596,.T.);
#4951=ORIENTED_EDGE('',*,*,#3539,.F.);
#4952=ORIENTED_EDGE('',*,*,#3605,.T.);
#4953=ORIENTED_EDGE('',*,*,#3606,.F.);
#4954=ORIENTED_EDGE('',*,*,#3607,.T.);
#4955=ORIENTED_EDGE('',*,*,#3532,.F.);
#4956=ORIENTED_EDGE('',*,*,#3599,.T.);
#4957=ORIENTED_EDGE('',*,*,#3608,.F.);
#4958=ORIENTED_EDGE('',*,*,#3602,.T.);
#4959=ORIENTED_EDGE('',*,*,#3528,.F.);
#4960=ORIENTED_EDGE('',*,*,#3609,.T.);
#4961=ORIENTED_EDGE('',*,*,#3591,.T.);
#4962=ORIENTED_EDGE('',*,*,#3609,.F.);
#4963=ORIENTED_EDGE('',*,*,#3527,.F.);
#4964=ORIENTED_EDGE('',*,*,#3593,.T.);
#4965=ORIENTED_EDGE('',*,*,#3610,.F.);
#4966=ORIENTED_EDGE('',*,*,#3606,.T.);
#4967=ORIENTED_EDGE('',*,*,#3611,.F.);
#4968=ORIENTED_EDGE('',*,*,#3612,.F.);
#4969=ORIENTED_EDGE('',*,*,#3597,.F.);
#4970=ORIENTED_EDGE('',*,*,#3610,.T.);
#4971=ORIENTED_EDGE('',*,*,#3595,.F.);
#4972=ORIENTED_EDGE('',*,*,#3613,.F.);
#4973=ORIENTED_EDGE('',*,*,#3603,.F.);
#4974=ORIENTED_EDGE('',*,*,#3608,.T.);
#4975=ORIENTED_EDGE('',*,*,#3601,.F.);
#4976=ORIENTED_EDGE('',*,*,#3614,.F.);
#4977=ORIENTED_EDGE('',*,*,#3615,.F.);
#4978=ORIENTED_EDGE('',*,*,#3616,.F.);
#4979=ORIENTED_EDGE('',*,*,#3600,.T.);
#4980=ORIENTED_EDGE('',*,*,#3534,.F.);
#4981=ORIENTED_EDGE('',*,*,#3617,.F.);
#4982=ORIENTED_EDGE('',*,*,#3614,.T.);
#4983=ORIENTED_EDGE('',*,*,#3594,.T.);
#4984=ORIENTED_EDGE('',*,*,#3530,.F.);
#4985=ORIENTED_EDGE('',*,*,#3604,.T.);
#4986=ORIENTED_EDGE('',*,*,#3613,.T.);
#4987=ORIENTED_EDGE('',*,*,#3540,.F.);
#4988=ORIENTED_EDGE('',*,*,#3618,.T.);
#4989=ORIENTED_EDGE('',*,*,#3616,.T.);
#4990=ORIENTED_EDGE('',*,*,#3618,.F.);
#4991=ORIENTED_EDGE('',*,*,#3598,.T.);
#4992=ORIENTED_EDGE('',*,*,#3612,.T.);
#4993=ORIENTED_EDGE('',*,*,#3619,.F.);
#4994=ORIENTED_EDGE('',*,*,#3537,.F.);
#4995=ORIENTED_EDGE('',*,*,#3617,.T.);
#4996=ORIENTED_EDGE('',*,*,#3533,.F.);
#4997=ORIENTED_EDGE('',*,*,#3607,.F.);
#4998=ORIENTED_EDGE('',*,*,#3615,.T.);
#4999=ORIENTED_EDGE('',*,*,#3620,.T.);
#5000=ORIENTED_EDGE('',*,*,#3548,.T.);
#5001=ORIENTED_EDGE('',*,*,#3337,.T.);
#5002=ORIENTED_EDGE('',*,*,#3544,.T.);
#5003=ORIENTED_EDGE('',*,*,#3519,.T.);
#5004=ORIENTED_EDGE('',*,*,#3568,.T.);
#5005=ORIENTED_EDGE('',*,*,#3389,.T.);
#5006=ORIENTED_EDGE('',*,*,#3565,.T.);
#5007=ORIENTED_EDGE('',*,*,#3467,.T.);
#5008=ORIENTED_EDGE('',*,*,#3574,.T.);
#5009=ORIENTED_EDGE('',*,*,#3363,.T.);
#5010=ORIENTED_EDGE('',*,*,#3571,.T.);
#5011=ORIENTED_EDGE('',*,*,#3441,.T.);
#5012=ORIENTED_EDGE('',*,*,#3562,.T.);
#5013=ORIENTED_EDGE('',*,*,#3415,.T.);
#5014=ORIENTED_EDGE('',*,*,#3559,.T.);
#5015=ORIENTED_EDGE('',*,*,#3493,.T.);
#5016=ORIENTED_EDGE('',*,*,#3524,.T.);
#5017=ORIENTED_EDGE('',*,*,#3619,.T.);
#5018=ORIENTED_EDGE('',*,*,#3611,.T.);
#5019=ORIENTED_EDGE('',*,*,#3605,.F.);
#5020=ORIENTED_EDGE('',*,*,#3538,.F.);
#5021=ORIENTED_EDGE('',*,*,#3620,.F.);
#5022=ORIENTED_EDGE('',*,*,#3621,.T.);
#5023=ORIENTED_EDGE('',*,*,#3549,.T.);
#5024=ORIENTED_EDGE('',*,*,#3621,.F.);
#5612=CYLINDRICAL_SURFACE('',#6563,0.25175);
#5613=CYLINDRICAL_SURFACE('',#6565,0.25175);
#5614=CYLINDRICAL_SURFACE('',#6566,0.25175);
#5615=CYLINDRICAL_SURFACE('',#6567,0.25175);
#5616=CYLINDRICAL_SURFACE('',#6568,0.25175);
#5617=CYLINDRICAL_SURFACE('',#6569,0.25175);
#5618=CYLINDRICAL_SURFACE('',#6570,0.25175);
#5619=CYLINDRICAL_SURFACE('',#6571,0.25175);
#5620=CYLINDRICAL_SURFACE('',#6573,0.25175);
#5621=CYLINDRICAL_SURFACE('',#6575,0.25175);
#5622=CYLINDRICAL_SURFACE('',#6576,0.25175);
#5623=CYLINDRICAL_SURFACE('',#6577,0.25175);
#5624=CYLINDRICAL_SURFACE('',#6578,0.25175);
#5625=CYLINDRICAL_SURFACE('',#6579,0.25175);
#5626=CYLINDRICAL_SURFACE('',#6580,0.25175);
#5627=CYLINDRICAL_SURFACE('',#6581,0.25175);
#5628=CYLINDRICAL_SURFACE('',#6583,0.25175);
#5629=CYLINDRICAL_SURFACE('',#6585,0.25175);
#5630=CYLINDRICAL_SURFACE('',#6586,0.25175);
#5631=CYLINDRICAL_SURFACE('',#6587,0.25175);
#5632=CYLINDRICAL_SURFACE('',#6588,0.25175);
#5633=CYLINDRICAL_SURFACE('',#6589,0.25175);
#5634=CYLINDRICAL_SURFACE('',#6590,0.25175);
#5635=CYLINDRICAL_SURFACE('',#6591,0.25175);
#5636=CYLINDRICAL_SURFACE('',#6593,0.25175);
#5637=CYLINDRICAL_SURFACE('',#6595,0.25175);
#5638=CYLINDRICAL_SURFACE('',#6596,0.25175);
#5639=CYLINDRICAL_SURFACE('',#6597,0.25175);
#5640=CYLINDRICAL_SURFACE('',#6598,0.25175);
#5641=CYLINDRICAL_SURFACE('',#6599,0.25175);
#5642=CYLINDRICAL_SURFACE('',#6600,0.25175);
#5643=CYLINDRICAL_SURFACE('',#6601,0.25175);
#5644=CYLINDRICAL_SURFACE('',#6603,0.30735);
#5645=CYLINDRICAL_SURFACE('',#6605,0.30735);
#5646=CYLINDRICAL_SURFACE('',#6606,0.30735);
#5647=CYLINDRICAL_SURFACE('',#6607,0.30735);
#5648=CYLINDRICAL_SURFACE('',#6608,0.30735);
#5649=CYLINDRICAL_SURFACE('',#6609,0.30735);
#5650=CYLINDRICAL_SURFACE('',#6610,0.30735);
#5651=CYLINDRICAL_SURFACE('',#6611,0.30735);
#5652=CYLINDRICAL_SURFACE('',#6613,0.30735);
#5653=CYLINDRICAL_SURFACE('',#6615,0.30735);
#5654=CYLINDRICAL_SURFACE('',#6616,0.30735);
#5655=CYLINDRICAL_SURFACE('',#6617,0.30735);
#5656=CYLINDRICAL_SURFACE('',#6618,0.30735);
#5657=CYLINDRICAL_SURFACE('',#6619,0.30735);
#5658=CYLINDRICAL_SURFACE('',#6620,0.30735);
#5659=CYLINDRICAL_SURFACE('',#6621,0.30735);
#5660=CYLINDRICAL_SURFACE('',#6623,0.30735);
#5661=CYLINDRICAL_SURFACE('',#6625,0.30735);
#5662=CYLINDRICAL_SURFACE('',#6626,0.30735);
#5663=CYLINDRICAL_SURFACE('',#6627,0.30735);
#5664=CYLINDRICAL_SURFACE('',#6628,0.30735);
#5665=CYLINDRICAL_SURFACE('',#6629,0.30735);
#5666=CYLINDRICAL_SURFACE('',#6630,0.30735);
#5667=CYLINDRICAL_SURFACE('',#6631,0.30735);
#5668=CYLINDRICAL_SURFACE('',#6633,0.30735);
#5669=CYLINDRICAL_SURFACE('',#6635,0.30735);
#5670=CYLINDRICAL_SURFACE('',#6636,0.30735);
#5671=CYLINDRICAL_SURFACE('',#6637,0.30735);
#5672=CYLINDRICAL_SURFACE('',#6638,0.30735);
#5673=CYLINDRICAL_SURFACE('',#6639,0.30735);
#5674=CYLINDRICAL_SURFACE('',#6640,0.30735);
#5675=CYLINDRICAL_SURFACE('',#6641,0.30735);
#5676=CYLINDRICAL_SURFACE('',#6643,6.35);
#5677=CYLINDRICAL_SURFACE('',#6646,6.85);
#5678=CYLINDRICAL_SURFACE('',#6659,0.30735);
#5679=CYLINDRICAL_SURFACE('',#6663,0.30735);
#5680=CYLINDRICAL_SURFACE('',#6664,0.30735);
#5681=CYLINDRICAL_SURFACE('',#6665,0.30735);
#5682=CYLINDRICAL_SURFACE('',#6666,0.25175);
#5683=CYLINDRICAL_SURFACE('',#6667,0.25175);
#5684=CYLINDRICAL_SURFACE('',#6668,0.25175);
#5685=CYLINDRICAL_SURFACE('',#6669,0.25175);
#5686=CYLINDRICAL_SURFACE('',#6670,0.35);
#5687=CYLINDRICAL_SURFACE('',#6673,0.35);
#5688=CYLINDRICAL_SURFACE('',#6676,0.35);
#5689=CYLINDRICAL_SURFACE('',#6679,0.35);
#5690=CYLINDRICAL_SURFACE('',#6685,4.8);
#5691=CYLINDRICAL_SURFACE('',#6689,3.5);
#5692=CYLINDRICAL_SURFACE('',#6694,2.7);
#5693=CYLINDRICAL_SURFACE('',#6703,2.1);
#5694=CYLINDRICAL_SURFACE('',#6704,2.1);
#5695=CYLINDRICAL_SURFACE('',#6705,1.7);
#5696=CYLINDRICAL_SURFACE('',#6706,2.1);
#5697=CYLINDRICAL_SURFACE('',#6711,8.2);
#5875=ADVANCED_FACE('',(#796),#5612,.F.);
#5876=ADVANCED_FACE('',(#797),#5613,.F.);
#5877=ADVANCED_FACE('',(#798),#5614,.F.);
#5878=ADVANCED_FACE('',(#799),#5615,.F.);
#5879=ADVANCED_FACE('',(#800),#5616,.F.);
#5880=ADVANCED_FACE('',(#801),#5617,.F.);
#5881=ADVANCED_FACE('',(#802),#5618,.F.);
#5882=ADVANCED_FACE('',(#803),#5619,.F.);
#5883=ADVANCED_FACE('',(#804),#5620,.F.);
#5884=ADVANCED_FACE('',(#805),#5621,.F.);
#5885=ADVANCED_FACE('',(#806),#5622,.F.);
#5886=ADVANCED_FACE('',(#807),#5623,.F.);
#5887=ADVANCED_FACE('',(#808),#5624,.F.);
#5888=ADVANCED_FACE('',(#809),#5625,.F.);
#5889=ADVANCED_FACE('',(#810),#5626,.F.);
#5890=ADVANCED_FACE('',(#811),#5627,.F.);
#5891=ADVANCED_FACE('',(#812),#5628,.F.);
#5892=ADVANCED_FACE('',(#813),#5629,.F.);
#5893=ADVANCED_FACE('',(#814),#5630,.F.);
#5894=ADVANCED_FACE('',(#815),#5631,.F.);
#5895=ADVANCED_FACE('',(#816),#5632,.F.);
#5896=ADVANCED_FACE('',(#817),#5633,.F.);
#5897=ADVANCED_FACE('',(#818),#5634,.F.);
#5898=ADVANCED_FACE('',(#819),#5635,.F.);
#5899=ADVANCED_FACE('',(#820),#5636,.F.);
#5900=ADVANCED_FACE('',(#821),#5637,.F.);
#5901=ADVANCED_FACE('',(#822),#5638,.F.);
#5902=ADVANCED_FACE('',(#823),#5639,.F.);
#5903=ADVANCED_FACE('',(#824),#5640,.F.);
#5904=ADVANCED_FACE('',(#825),#5641,.F.);
#5905=ADVANCED_FACE('',(#826),#5642,.F.);
#5906=ADVANCED_FACE('',(#827),#5643,.F.);
#5907=ADVANCED_FACE('',(#828),#5644,.F.);
#5908=ADVANCED_FACE('',(#829),#5645,.F.);
#5909=ADVANCED_FACE('',(#830),#5646,.F.);
#5910=ADVANCED_FACE('',(#831),#5647,.F.);
#5911=ADVANCED_FACE('',(#832),#5648,.F.);
#5912=ADVANCED_FACE('',(#833),#5649,.F.);
#5913=ADVANCED_FACE('',(#834),#5650,.F.);
#5914=ADVANCED_FACE('',(#835),#5651,.F.);
#5915=ADVANCED_FACE('',(#836),#5652,.F.);
#5916=ADVANCED_FACE('',(#837),#5653,.F.);
#5917=ADVANCED_FACE('',(#838),#5654,.F.);
#5918=ADVANCED_FACE('',(#839),#5655,.F.);
#5919=ADVANCED_FACE('',(#840),#5656,.F.);
#5920=ADVANCED_FACE('',(#841),#5657,.F.);
#5921=ADVANCED_FACE('',(#842),#5658,.F.);
#5922=ADVANCED_FACE('',(#843),#5659,.F.);
#5923=ADVANCED_FACE('',(#844),#5660,.F.);
#5924=ADVANCED_FACE('',(#845),#5661,.F.);
#5925=ADVANCED_FACE('',(#846),#5662,.F.);
#5926=ADVANCED_FACE('',(#847),#5663,.F.);
#5927=ADVANCED_FACE('',(#848),#5664,.F.);
#5928=ADVANCED_FACE('',(#849),#5665,.F.);
#5929=ADVANCED_FACE('',(#850),#5666,.F.);
#5930=ADVANCED_FACE('',(#851),#5667,.F.);
#5931=ADVANCED_FACE('',(#852),#5668,.F.);
#5932=ADVANCED_FACE('',(#853),#5669,.F.);
#5933=ADVANCED_FACE('',(#854),#5670,.F.);
#5934=ADVANCED_FACE('',(#855),#5671,.F.);
#5935=ADVANCED_FACE('',(#856),#5672,.F.);
#5936=ADVANCED_FACE('',(#857),#5673,.F.);
#5937=ADVANCED_FACE('',(#858),#5674,.F.);
#5938=ADVANCED_FACE('',(#859),#5675,.F.);
#5939=ADVANCED_FACE('',(#860),#5676,.T.);
#5940=ADVANCED_FACE('',(#861),#5677,.F.);
#5941=ADVANCED_FACE('',(#862,#477),#614,.T.);
#5942=ADVANCED_FACE('',(#863,#478,#479,#480,#481),#615,.T.);
#5943=ADVANCED_FACE('',(#864),#5678,.F.);
#5944=ADVANCED_FACE('',(#865),#138,.F.);
#5945=ADVANCED_FACE('',(#866),#139,.F.);
#5946=ADVANCED_FACE('',(#867,#482,#483,#484,#485,#486),#616,.F.);
#5947=ADVANCED_FACE('',(#868),#5679,.F.);
#5948=ADVANCED_FACE('',(#869),#140,.F.);
#5949=ADVANCED_FACE('',(#870),#141,.F.);
#5950=ADVANCED_FACE('',(#871),#5680,.F.);
#5951=ADVANCED_FACE('',(#872),#142,.F.);
#5952=ADVANCED_FACE('',(#873),#143,.F.);
#5953=ADVANCED_FACE('',(#874),#5681,.F.);
#5954=ADVANCED_FACE('',(#875),#144,.F.);
#5955=ADVANCED_FACE('',(#876),#145,.F.);
#5956=ADVANCED_FACE('',(#877),#5682,.F.);
#5957=ADVANCED_FACE('',(#878),#5683,.F.);
#5958=ADVANCED_FACE('',(#879),#5684,.F.);
#5959=ADVANCED_FACE('',(#880),#5685,.F.);
#5960=ADVANCED_FACE('',(#881),#5686,.F.);
#5961=ADVANCED_FACE('',(#882),#5687,.F.);
#5962=ADVANCED_FACE('',(#883),#5688,.F.);
#5963=ADVANCED_FACE('',(#884),#5689,.F.);
#5964=ADVANCED_FACE('',(#885,#487,#488,#489,#490,#491),#617,.T.);
#5965=ADVANCED_FACE('',(#886),#5690,.T.);
#5966=ADVANCED_FACE('',(#887,#492,#493,#494,#495,#496),#618,.F.);
#5967=ADVANCED_FACE('',(#888),#5691,.T.);
#5968=ADVANCED_FACE('',(#889),#619,.T.);
#5969=ADVANCED_FACE('',(#890),#620,.T.);
#5970=ADVANCED_FACE('',(#891),#621,.T.);
#5971=ADVANCED_FACE('',(#892),#622,.T.);
#5972=ADVANCED_FACE('',(#893),#5692,.F.);
#5973=ADVANCED_FACE('',(#894,#497),#623,.F.);
#5974=ADVANCED_FACE('',(#895),#5693,.T.);
#5975=ADVANCED_FACE('',(#896),#5694,.T.);
#5976=ADVANCED_FACE('',(#897),#5695,.F.);
#5977=ADVANCED_FACE('',(#898),#5696,.T.);
#5978=ADVANCED_FACE('',(#899),#624,.T.);
#5979=ADVANCED_FACE('',(#900,#498,#499,#500,#501,#502),#625,.T.);
#5980=ADVANCED_FACE('',(#901),#626,.T.);
#5981=ADVANCED_FACE('',(#902),#5697,.T.);
#6116=CLOSED_SHELL('',(#5875,#5876,#5877,#5878,#5879,#5880,#5881,#5882,
#5883,#5884,#5885,#5886,#5887,#5888,#5889,#5890,#5891,#5892,#5893,#5894,
#5895,#5896,#5897,#5898,#5899,#5900,#5901,#5902,#5903,#5904,#5905,#5906,
#5907,#5908,#5909,#5910,#5911,#5912,#5913,#5914,#5915,#5916,#5917,#5918,
#5919,#5920,#5921,#5922,#5923,#5924,#5925,#5926,#5927,#5928,#5929,#5930,
#5931,#5932,#5933,#5934,#5935,#5936,#5937,#5938,#5939,#5940,#5941,#5942,
#5943,#5944,#5945,#5946,#5947,#5948,#5949,#5950,#5951,#5952,#5953,#5954,
#5955,#5956,#5957,#5958,#5959,#5960,#5961,#5962,#5963,#5964,#5965,#5966,
#5967,#5968,#5969,#5970,#5971,#5972,#5973,#5974,#5975,#5976,#5977,#5978,
#5979,#5980,#5981));
#6562=AXIS2_PLACEMENT_3D('',#9196,#7582,#7583);
#6563=AXIS2_PLACEMENT_3D('',#9197,#7584,#7585);
#6564=AXIS2_PLACEMENT_3D('',#9207,#7587,#7588);
#6565=AXIS2_PLACEMENT_3D('',#9218,#7589,#7590);
#6566=AXIS2_PLACEMENT_3D('',#9269,#7592,#7593);
#6567=AXIS2_PLACEMENT_3D('',#9320,#7595,#7596);
#6568=AXIS2_PLACEMENT_3D('',#9368,#7598,#7599);
#6569=AXIS2_PLACEMENT_3D('',#9419,#7601,#7602);
#6570=AXIS2_PLACEMENT_3D('',#9470,#7604,#7605);
#6571=AXIS2_PLACEMENT_3D('',#9518,#7607,#7608);
#6572=AXIS2_PLACEMENT_3D('',#9537,#7610,#7611);
#6573=AXIS2_PLACEMENT_3D('',#9557,#7612,#7613);
#6574=AXIS2_PLACEMENT_3D('',#9567,#7615,#7616);
#6575=AXIS2_PLACEMENT_3D('',#9578,#7617,#7618);
#6576=AXIS2_PLACEMENT_3D('',#9629,#7620,#7621);
#6577=AXIS2_PLACEMENT_3D('',#9680,#7623,#7624);
#6578=AXIS2_PLACEMENT_3D('',#9728,#7626,#7627);
#6579=AXIS2_PLACEMENT_3D('',#9779,#7629,#7630);
#6580=AXIS2_PLACEMENT_3D('',#9830,#7632,#7633);
#6581=AXIS2_PLACEMENT_3D('',#9878,#7635,#7636);
#6582=AXIS2_PLACEMENT_3D('',#9897,#7638,#7639);
#6583=AXIS2_PLACEMENT_3D('',#9917,#7640,#7641);
#6584=AXIS2_PLACEMENT_3D('',#9927,#7643,#7644);
#6585=AXIS2_PLACEMENT_3D('',#9938,#7645,#7646);
#6586=AXIS2_PLACEMENT_3D('',#9989,#7648,#7649);
#6587=AXIS2_PLACEMENT_3D('',#10040,#7651,#7652);
#6588=AXIS2_PLACEMENT_3D('',#10088,#7654,#7655);
#6589=AXIS2_PLACEMENT_3D('',#10139,#7657,#7658);
#6590=AXIS2_PLACEMENT_3D('',#10190,#7660,#7661);
#6591=AXIS2_PLACEMENT_3D('',#10238,#7663,#7664);
#6592=AXIS2_PLACEMENT_3D('',#10257,#7666,#7667);
#6593=AXIS2_PLACEMENT_3D('',#10277,#7668,#7669);
#6594=AXIS2_PLACEMENT_3D('',#10287,#7671,#7672);
#6595=AXIS2_PLACEMENT_3D('',#10298,#7673,#7674);
#6596=AXIS2_PLACEMENT_3D('',#10349,#7676,#7677);
#6597=AXIS2_PLACEMENT_3D('',#10400,#7679,#7680);
#6598=AXIS2_PLACEMENT_3D('',#10448,#7682,#7683);
#6599=AXIS2_PLACEMENT_3D('',#10499,#7685,#7686);
#6600=AXIS2_PLACEMENT_3D('',#10550,#7688,#7689);
#6601=AXIS2_PLACEMENT_3D('',#10598,#7691,#7692);
#6602=AXIS2_PLACEMENT_3D('',#10617,#7694,#7695);
#6603=AXIS2_PLACEMENT_3D('',#10637,#7696,#7697);
#6604=AXIS2_PLACEMENT_3D('',#10651,#7699,#7700);
#6605=AXIS2_PLACEMENT_3D('',#10661,#7701,#7702);
#6606=AXIS2_PLACEMENT_3D('',#10685,#7704,#7705);
#6607=AXIS2_PLACEMENT_3D('',#10710,#7707,#7708);
#6608=AXIS2_PLACEMENT_3D('',#10735,#7710,#7711);
#6609=AXIS2_PLACEMENT_3D('',#10759,#7713,#7714);
#6610=AXIS2_PLACEMENT_3D('',#10784,#7716,#7717);
#6611=AXIS2_PLACEMENT_3D('',#10809,#7719,#7720);
#6612=AXIS2_PLACEMENT_3D('',#10820,#7722,#7723);
#6613=AXIS2_PLACEMENT_3D('',#10826,#7724,#7725);
#6614=AXIS2_PLACEMENT_3D('',#10840,#7727,#7728);
#6615=AXIS2_PLACEMENT_3D('',#10850,#7729,#7730);
#6616=AXIS2_PLACEMENT_3D('',#10874,#7732,#7733);
#6617=AXIS2_PLACEMENT_3D('',#10899,#7735,#7736);
#6618=AXIS2_PLACEMENT_3D('',#10924,#7738,#7739);
#6619=AXIS2_PLACEMENT_3D('',#10948,#7741,#7742);
#6620=AXIS2_PLACEMENT_3D('',#10973,#7744,#7745);
#6621=AXIS2_PLACEMENT_3D('',#10998,#7747,#7748);
#6622=AXIS2_PLACEMENT_3D('',#11009,#7750,#7751);
#6623=AXIS2_PLACEMENT_3D('',#11015,#7752,#7753);
#6624=AXIS2_PLACEMENT_3D('',#11029,#7755,#7756);
#6625=AXIS2_PLACEMENT_3D('',#11039,#7757,#7758);
#6626=AXIS2_PLACEMENT_3D('',#11063,#7760,#7761);
#6627=AXIS2_PLACEMENT_3D('',#11088,#7763,#7764);
#6628=AXIS2_PLACEMENT_3D('',#11113,#7766,#7767);
#6629=AXIS2_PLACEMENT_3D('',#11137,#7769,#7770);
#6630=AXIS2_PLACEMENT_3D('',#11162,#7772,#7773);
#6631=AXIS2_PLACEMENT_3D('',#11187,#7775,#7776);
#6632=AXIS2_PLACEMENT_3D('',#11198,#7778,#7779);
#6633=AXIS2_PLACEMENT_3D('',#11204,#7780,#7781);
#6634=AXIS2_PLACEMENT_3D('',#11218,#7783,#7784);
#6635=AXIS2_PLACEMENT_3D('',#11228,#7785,#7786);
#6636=AXIS2_PLACEMENT_3D('',#11252,#7788,#7789);
#6637=AXIS2_PLACEMENT_3D('',#11277,#7791,#7792);
#6638=AXIS2_PLACEMENT_3D('',#11302,#7794,#7795);
#6639=AXIS2_PLACEMENT_3D('',#11326,#7797,#7798);
#6640=AXIS2_PLACEMENT_3D('',#11351,#7800,#7801);
#6641=AXIS2_PLACEMENT_3D('',#11376,#7803,#7804);
#6642=AXIS2_PLACEMENT_3D('',#11387,#7806,#7807);
#6643=AXIS2_PLACEMENT_3D('',#11393,#7808,#7809);
#6644=AXIS2_PLACEMENT_3D('',#11395,#7810,#7811);
#6645=AXIS2_PLACEMENT_3D('',#11398,#7813,#7814);
#6646=AXIS2_PLACEMENT_3D('',#11399,#7815,#7816);
#6647=AXIS2_PLACEMENT_3D('',#11401,#7817,#7818);
#6648=AXIS2_PLACEMENT_3D('',#11404,#7820,#7821);
#6649=AXIS2_PLACEMENT_3D('',#11405,#7822,#7823);
#6650=AXIS2_PLACEMENT_3D('',#11406,#7824,#7825);
#6651=AXIS2_PLACEMENT_3D('',#11409,#7826,#7827);
#6652=AXIS2_PLACEMENT_3D('',#11411,#7828,#7829);
#6653=AXIS2_PLACEMENT_3D('',#11415,#7831,#7832);
#6654=AXIS2_PLACEMENT_3D('',#11419,#7834,#7835);
#6655=AXIS2_PLACEMENT_3D('',#11423,#7837,#7838);
#6656=AXIS2_PLACEMENT_3D('',#11429,#7841,#7842);
#6657=AXIS2_PLACEMENT_3D('',#11432,#7844,#7845);
#6658=AXIS2_PLACEMENT_3D('',#11434,#7846,#7847);
#6659=AXIS2_PLACEMENT_3D('',#11435,#7848,#7849);
#6660=AXIS2_PLACEMENT_3D('',#12187,#7850,#7851);
#6661=AXIS2_PLACEMENT_3D('',#12189,#7852,#7853);
#6662=AXIS2_PLACEMENT_3D('',#12191,#7854,#7855);
#6663=AXIS2_PLACEMENT_3D('',#12540,#7856,#7857);
#6664=AXIS2_PLACEMENT_3D('',#13176,#7858,#7859);
#6665=AXIS2_PLACEMENT_3D('',#13812,#7860,#7861);
#6666=AXIS2_PLACEMENT_3D('',#14448,#7862,#7863);
#6667=AXIS2_PLACEMENT_3D('',#14449,#7864,#7865);
#6668=AXIS2_PLACEMENT_3D('',#14450,#7866,#7867);
#6669=AXIS2_PLACEMENT_3D('',#14451,#7868,#7869);
#6670=AXIS2_PLACEMENT_3D('',#14452,#7870,#7871);
#6671=AXIS2_PLACEMENT_3D('',#14454,#7872,#7873);
#6672=AXIS2_PLACEMENT_3D('',#14457,#7875,#7876);
#6673=AXIS2_PLACEMENT_3D('',#14458,#7877,#7878);
#6674=AXIS2_PLACEMENT_3D('',#14460,#7879,#7880);
#6675=AXIS2_PLACEMENT_3D('',#14463,#7882,#7883);
#6676=AXIS2_PLACEMENT_3D('',#14464,#7884,#7885);
#6677=AXIS2_PLACEMENT_3D('',#14466,#7886,#7887);
#6678=AXIS2_PLACEMENT_3D('',#14469,#7889,#7890);
#6679=AXIS2_PLACEMENT_3D('',#14470,#7891,#7892);
#6680=AXIS2_PLACEMENT_3D('',#14472,#7893,#7894);
#6681=AXIS2_PLACEMENT_3D('',#14475,#7896,#7897);
#6682=AXIS2_PLACEMENT_3D('',#14476,#7898,#7899);
#6683=AXIS2_PLACEMENT_3D('',#14478,#7900,#7901);
#6684=AXIS2_PLACEMENT_3D('',#14480,#7902,#7903);
#6685=AXIS2_PLACEMENT_3D('',#14481,#7904,#7905);
#6686=AXIS2_PLACEMENT_3D('',#14484,#7907,#7908);
#6687=AXIS2_PLACEMENT_3D('',#14485,#7909,#7910);
#6688=AXIS2_PLACEMENT_3D('',#14487,#7911,#7912);
#6689=AXIS2_PLACEMENT_3D('',#14488,#7913,#7914);
#6690=AXIS2_PLACEMENT_3D('',#14490,#7916,#7917);
#6691=AXIS2_PLACEMENT_3D('',#14496,#7921,#7922);
#6692=AXIS2_PLACEMENT_3D('',#14502,#7926,#7927);
#6693=AXIS2_PLACEMENT_3D('',#14508,#7931,#7932);
#6694=AXIS2_PLACEMENT_3D('',#14514,#7936,#7937);
#6695=AXIS2_PLACEMENT_3D('',#14518,#7939,#7940);
#6696=AXIS2_PLACEMENT_3D('',#14520,#7942,#7943);
#6697=AXIS2_PLACEMENT_3D('',#14522,#7945,#7946);
#6698=AXIS2_PLACEMENT_3D('',#14523,#7947,#7948);
#6699=AXIS2_PLACEMENT_3D('',#14526,#7950,#7951);
#6700=AXIS2_PLACEMENT_3D('',#14527,#7952,#7953);
#6701=AXIS2_PLACEMENT_3D('',#14529,#7954,#7955);
#6702=AXIS2_PLACEMENT_3D('',#14532,#7957,#7958);
#6703=AXIS2_PLACEMENT_3D('',#14533,#7959,#7960);
#6704=AXIS2_PLACEMENT_3D('',#14535,#7962,#7963);
#6705=AXIS2_PLACEMENT_3D('',#14536,#7964,#7965);
#6706=AXIS2_PLACEMENT_3D('',#14538,#7967,#7968);
#6707=AXIS2_PLACEMENT_3D('',#14540,#7970,#7971);
#6708=AXIS2_PLACEMENT_3D('',#14541,#7972,#7973);
#6709=AXIS2_PLACEMENT_3D('',#14543,#7974,#7975);
#6710=AXIS2_PLACEMENT_3D('',#14544,#7976,#7977);
#6711=AXIS2_PLACEMENT_3D('',#14545,#7978,#7979);
#7582=DIRECTION('axis',(0.,0.,1.));
#7583=DIRECTION('refdir',(1.,0.,0.));
#7584=DIRECTION('center_axis',(0.,0.,-1.));
#7585=DIRECTION('ref_axis',(-0.346876982621325,0.937910634830166,0.));
#7586=DIRECTION('',(0.,0.,-1.));
#7587=DIRECTION('center_axis',(0.,0.,-1.));
#7588=DIRECTION('ref_axis',(1.,0.,0.));
#7589=DIRECTION('center_axis',(0.,0.,-1.));
#7590=DIRECTION('ref_axis',(1.,0.,0.));
#7591=DIRECTION('',(0.,0.,-1.));
#7592=DIRECTION('center_axis',(0.,0.,-1.));
#7593=DIRECTION('ref_axis',(1.,0.,0.));
#7594=DIRECTION('',(0.,0.,-1.));
#7595=DIRECTION('center_axis',(0.,0.,-1.));
#7596=DIRECTION('ref_axis',(1.,0.,0.));
#7597=DIRECTION('',(0.,0.,-1.));
#7598=DIRECTION('center_axis',(0.,0.,-1.));
#7599=DIRECTION('ref_axis',(1.,0.,0.));
#7600=DIRECTION('',(0.,0.,-1.));
#7601=DIRECTION('center_axis',(0.,0.,-1.));
#7602=DIRECTION('ref_axis',(1.,0.,0.));
#7603=DIRECTION('',(0.,0.,-1.));
#7604=DIRECTION('center_axis',(0.,0.,-1.));
#7605=DIRECTION('ref_axis',(1.,0.,0.));
#7606=DIRECTION('',(0.,0.,-1.));
#7607=DIRECTION('center_axis',(0.,0.,-1.));
#7608=DIRECTION('ref_axis',(0.93800197321156,-0.346629915401454,0.));
#7609=DIRECTION('',(0.,0.,-1.));
#7610=DIRECTION('center_axis',(0.,0.,-1.));
#7611=DIRECTION('ref_axis',(1.,0.,0.));
#7612=DIRECTION('center_axis',(0.,0.,-1.));
#7613=DIRECTION('ref_axis',(-0.346877122944053,0.937910582933179,0.));
#7614=DIRECTION('',(0.,0.,-1.));
#7615=DIRECTION('center_axis',(0.,0.,-1.));
#7616=DIRECTION('ref_axis',(1.,0.,0.));
#7617=DIRECTION('center_axis',(0.,0.,-1.));
#7618=DIRECTION('ref_axis',(1.,0.,0.));
#7619=DIRECTION('',(0.,0.,-1.));
#7620=DIRECTION('center_axis',(0.,0.,-1.));
#7621=DIRECTION('ref_axis',(1.,0.,0.));
#7622=DIRECTION('',(0.,0.,-1.));
#7623=DIRECTION('center_axis',(0.,0.,-1.));
#7624=DIRECTION('ref_axis',(1.,0.,0.));
#7625=DIRECTION('',(0.,0.,-1.));
#7626=DIRECTION('center_axis',(0.,0.,-1.));
#7627=DIRECTION('ref_axis',(1.,0.,0.));
#7628=DIRECTION('',(0.,0.,-1.));
#7629=DIRECTION('center_axis',(0.,0.,-1.));
#7630=DIRECTION('ref_axis',(1.,0.,0.));
#7631=DIRECTION('',(0.,0.,-1.));
#7632=DIRECTION('center_axis',(0.,0.,-1.));
#7633=DIRECTION('ref_axis',(1.,0.,0.));
#7634=DIRECTION('',(0.,0.,-1.));
#7635=DIRECTION('center_axis',(0.,0.,-1.));
#7636=DIRECTION('ref_axis',(0.93800198232385,-0.346629890743035,0.));
#7637=DIRECTION('',(0.,0.,-1.));
#7638=DIRECTION('center_axis',(0.,0.,-1.));
#7639=DIRECTION('ref_axis',(1.,0.,0.));
#7640=DIRECTION('center_axis',(0.,0.,-1.));
#7641=DIRECTION('ref_axis',(-0.346876854373397,0.937910682261385,0.));
#7642=DIRECTION('',(0.,0.,-1.));
#7643=DIRECTION('center_axis',(0.,0.,-1.));
#7644=DIRECTION('ref_axis',(1.,0.,0.));
#7645=DIRECTION('center_axis',(0.,0.,-1.));
#7646=DIRECTION('ref_axis',(1.,0.,0.));
#7647=DIRECTION('',(0.,0.,-1.));
#7648=DIRECTION('center_axis',(0.,0.,-1.));
#7649=DIRECTION('ref_axis',(1.,0.,0.));
#7650=DIRECTION('',(0.,0.,-1.));
#7651=DIRECTION('center_axis',(0.,0.,-1.));
#7652=DIRECTION('ref_axis',(1.,0.,0.));
#7653=DIRECTION('',(0.,0.,-1.));
#7654=DIRECTION('center_axis',(0.,0.,-1.));
#7655=DIRECTION('ref_axis',(1.,0.,0.));
#7656=DIRECTION('',(0.,0.,-1.));
#7657=DIRECTION('center_axis',(0.,0.,-1.));
#7658=DIRECTION('ref_axis',(1.,0.,0.));
#7659=DIRECTION('',(0.,0.,-1.));
#7660=DIRECTION('center_axis',(0.,0.,-1.));
#7661=DIRECTION('ref_axis',(1.,0.,0.));
#7662=DIRECTION('',(0.,0.,-1.));
#7663=DIRECTION('center_axis',(0.,0.,-1.));
#7664=DIRECTION('ref_axis',(0.938001962568159,-0.346629944203154,0.));
#7665=DIRECTION('',(0.,0.,-1.));
#7666=DIRECTION('center_axis',(0.,0.,-1.));
#7667=DIRECTION('ref_axis',(1.,0.,0.));
#7668=DIRECTION('center_axis',(0.,0.,-1.));
#7669=DIRECTION('ref_axis',(-0.346877157281527,0.937910570233797,0.));
#7670=DIRECTION('',(0.,0.,-1.));
#7671=DIRECTION('center_axis',(0.,0.,-1.));
#7672=DIRECTION('ref_axis',(1.,0.,0.));
#7673=DIRECTION('center_axis',(0.,0.,-1.));
#7674=DIRECTION('ref_axis',(1.,0.,0.));
#7675=DIRECTION('',(0.,0.,-1.));
#7676=DIRECTION('center_axis',(0.,0.,-1.));
#7677=DIRECTION('ref_axis',(1.,0.,0.));
#7678=DIRECTION('',(0.,0.,-1.));
#7679=DIRECTION('center_axis',(0.,0.,-1.));
#7680=DIRECTION('ref_axis',(1.,0.,0.));
#7681=DIRECTION('',(0.,0.,-1.));
#7682=DIRECTION('center_axis',(0.,0.,-1.));
#7683=DIRECTION('ref_axis',(1.,0.,0.));
#7684=DIRECTION('',(0.,0.,-1.));
#7685=DIRECTION('center_axis',(0.,0.,-1.));
#7686=DIRECTION('ref_axis',(1.,0.,0.));
#7687=DIRECTION('',(0.,0.,-1.));
#7688=DIRECTION('center_axis',(0.,0.,-1.));
#7689=DIRECTION('ref_axis',(1.,0.,0.));
#7690=DIRECTION('',(0.,0.,-1.));
#7691=DIRECTION('center_axis',(0.,0.,-1.));
#7692=DIRECTION('ref_axis',(0.938001982323848,-0.346629890743041,0.));
#7693=DIRECTION('',(0.,0.,-1.));
#7694=DIRECTION('center_axis',(0.,0.,-1.));
#7695=DIRECTION('ref_axis',(1.,0.,0.));
#7696=DIRECTION('center_axis',(0.,0.,-1.));
#7697=DIRECTION('ref_axis',(0.793238951796279,0.608910474005121,0.));
#7698=DIRECTION('',(1.22464679914735E-16,-2.8461799209306E-30,-1.));
#7699=DIRECTION('center_axis',(0.,0.,1.));
#7700=DIRECTION('ref_axis',(1.,-2.31183580855735E-14,0.));
#7701=DIRECTION('center_axis',(0.,0.,-1.));
#7702=DIRECTION('ref_axis',(1.,-2.31183580855735E-14,0.));
#7703=DIRECTION('',(1.22464679914735E-16,-2.8461799209306E-30,-1.));
#7704=DIRECTION('center_axis',(0.,0.,-1.));
#7705=DIRECTION('ref_axis',(1.,-2.31183580855735E-14,0.));
#7706=DIRECTION('',(1.22464679914735E-16,-2.8461799209306E-30,-1.));
#7707=DIRECTION('center_axis',(0.,0.,-1.));
#7708=DIRECTION('ref_axis',(1.,-2.31183580855735E-14,0.));
#7709=DIRECTION('',(1.22464679914735E-16,-2.8461799209306E-30,-1.));
#7710=DIRECTION('center_axis',(0.,0.,-1.));
#7711=DIRECTION('ref_axis',(1.,-2.31183580855735E-14,0.));
#7712=DIRECTION('',(1.22464679914735E-16,-2.8461799209306E-30,-1.));
#7713=DIRECTION('center_axis',(0.,0.,-1.));
#7714=DIRECTION('ref_axis',(1.,-2.31183580855735E-14,0.));
#7715=DIRECTION('',(1.22464679914735E-16,-2.8461799209306E-30,-1.));
#7716=DIRECTION('center_axis',(0.,0.,-1.));
#7717=DIRECTION('ref_axis',(1.,-2.31183580855735E-14,0.));
#7718=DIRECTION('',(1.22464679914735E-16,-2.8461799209306E-30,-1.));
#7719=DIRECTION('center_axis',(0.,0.,-1.));
#7720=DIRECTION('ref_axis',(-0.609093803263995,-0.793098189901731,0.));
#7721=DIRECTION('',(1.22464679914735E-16,-2.8461799209306E-30,-1.));
#7722=DIRECTION('center_axis',(0.,0.,-1.));
#7723=DIRECTION('ref_axis',(1.,-2.31183580855735E-14,0.));
#7724=DIRECTION('center_axis',(0.,0.,-1.));
#7725=DIRECTION('ref_axis',(0.793238910128574,0.608910528286408,0.));
#7726=DIRECTION('',(1.22464679914735E-16,-2.2355846543427E-30,-1.));
#7727=DIRECTION('center_axis',(0.,0.,1.));
#7728=DIRECTION('ref_axis',(1.,-1.81324693622859E-14,0.));
#7729=DIRECTION('center_axis',(0.,0.,-1.));
#7730=DIRECTION('ref_axis',(1.,-1.81324693622859E-14,0.));
#7731=DIRECTION('',(1.22464679914735E-16,-2.2355846543427E-30,-1.));
#7732=DIRECTION('center_axis',(0.,0.,-1.));
#7733=DIRECTION('ref_axis',(1.,-1.81324693622859E-14,0.));
#7734=DIRECTION('',(1.22464679914735E-16,-2.2355846543427E-30,-1.));
#7735=DIRECTION('center_axis',(0.,0.,-1.));
#7736=DIRECTION('ref_axis',(1.,-1.81324693622859E-14,0.));
#7737=DIRECTION('',(1.22464679914735E-16,-2.2355846543427E-30,-1.));
#7738=DIRECTION('center_axis',(0.,0.,-1.));
#7739=DIRECTION('ref_axis',(1.,-1.81324693622859E-14,0.));
#7740=DIRECTION('',(1.22464679914735E-16,-2.2355846543427E-30,-1.));
#7741=DIRECTION('center_axis',(0.,0.,-1.));
#7742=DIRECTION('ref_axis',(1.,-1.81324693622859E-14,0.));
#7743=DIRECTION('',(1.22464679914735E-16,-2.2355846543427E-30,-1.));
#7744=DIRECTION('center_axis',(0.,0.,-1.));
#7745=DIRECTION('ref_axis',(1.,-1.81324693622859E-14,0.));
#7746=DIRECTION('',(1.22464679914735E-16,-2.2355846543427E-30,-1.));
#7747=DIRECTION('center_axis',(0.,0.,-1.));
#7748=DIRECTION('ref_axis',(-0.609093787363252,-0.793098202113388,0.));
#7749=DIRECTION('',(1.22464679914735E-16,-2.2355846543427E-30,-1.));
#7750=DIRECTION('center_axis',(0.,0.,-1.));
#7751=DIRECTION('ref_axis',(1.,-1.81324693622859E-14,0.));
#7752=DIRECTION('center_axis',(0.,0.,-1.));
#7753=DIRECTION('ref_axis',(0.793238959206298,0.608910464351951,0.));
#7754=DIRECTION('',(1.22464679914735E-16,-2.23556116661122E-30,-1.));
#7755=DIRECTION('center_axis',(0.,0.,1.));
#7756=DIRECTION('ref_axis',(1.,-1.81322775704035E-14,0.));
#7757=DIRECTION('center_axis',(0.,0.,-1.));
#7758=DIRECTION('ref_axis',(1.,-1.81322775704035E-14,0.));
#7759=DIRECTION('',(1.22464679914735E-16,-2.23556116661122E-30,-1.));
#7760=DIRECTION('center_axis',(0.,0.,-1.));
#7761=DIRECTION('ref_axis',(1.,-1.81322775704035E-14,0.));
#7762=DIRECTION('',(1.22464679914735E-16,-2.23556116661122E-30,-1.));
#7763=DIRECTION('center_axis',(0.,0.,-1.));
#7764=DIRECTION('ref_axis',(1.,-1.81322775704035E-14,0.));
#7765=DIRECTION('',(1.22464679914735E-16,-2.23556116661122E-30,-1.));
#7766=DIRECTION('center_axis',(0.,0.,-1.));
#7767=DIRECTION('ref_axis',(1.,-1.81322775704035E-14,0.));
#7768=DIRECTION('',(1.22464679914735E-16,-2.23556116661122E-30,-1.));
#7769=DIRECTION('center_axis',(0.,0.,-1.));
#7770=DIRECTION('ref_axis',(1.,-1.81322775704035E-14,0.));
#7771=DIRECTION('',(1.22464679914735E-16,-2.23556116661122E-30,-1.));
#7772=DIRECTION('center_axis',(0.,0.,-1.));
#7773=DIRECTION('ref_axis',(1.,-1.81322775704035E-14,0.));
#7774=DIRECTION('',(1.22464679914735E-16,-2.23556116661122E-30,-1.));
#7775=DIRECTION('center_axis',(0.,0.,-1.));
#7776=DIRECTION('ref_axis',(-0.609093821447985,-0.793098175936555,0.));
#7777=DIRECTION('',(1.22464679914735E-16,-2.23556116661122E-30,-1.));
#7778=DIRECTION('center_axis',(0.,0.,-1.));
#7779=DIRECTION('ref_axis',(1.,-1.81322775704035E-14,0.));
#7780=DIRECTION('center_axis',(0.,0.,-1.));
#7781=DIRECTION('ref_axis',(0.793238929068431,0.608910503613107,0.));
#7782=DIRECTION('',(1.22464679914735E-16,-1.43058875937861E-30,-1.));
#7783=DIRECTION('center_axis',(0.,0.,1.));
#7784=DIRECTION('ref_axis',(1.,-1.15591790427867E-14,0.));
#7785=DIRECTION('center_axis',(0.,0.,-1.));
#7786=DIRECTION('ref_axis',(1.,-1.15591790427867E-14,0.));
#7787=DIRECTION('',(1.22464679914735E-16,-1.43058875937861E-30,-1.));
#7788=DIRECTION('center_axis',(0.,0.,-1.));
#7789=DIRECTION('ref_axis',(1.,-1.15591790427867E-14,0.));
#7790=DIRECTION('',(1.22464679914735E-16,-1.43058875937861E-30,-1.));
#7791=DIRECTION('center_axis',(0.,0.,-1.));
#7792=DIRECTION('ref_axis',(1.,-1.15591790427867E-14,0.));
#7793=DIRECTION('',(1.22464679914735E-16,-1.43058875937861E-30,-1.));
#7794=DIRECTION('center_axis',(0.,0.,-1.));
#7795=DIRECTION('ref_axis',(1.,-1.15591790427867E-14,0.));
#7796=DIRECTION('',(1.22464679914735E-16,-1.43058875937861E-30,-1.));
#7797=DIRECTION('center_axis',(0.,0.,-1.));
#7798=DIRECTION('ref_axis',(1.,-1.15591790427867E-14,0.));
#7799=DIRECTION('',(1.22464679914735E-16,-1.43058875937861E-30,-1.));
#7800=DIRECTION('center_axis',(0.,0.,-1.));
#7801=DIRECTION('ref_axis',(1.,-1.15591790427867E-14,0.));
#7802=DIRECTION('',(1.22464679914735E-16,-1.43058875937861E-30,-1.));
#7803=DIRECTION('center_axis',(0.,0.,-1.));
#7804=DIRECTION('ref_axis',(-0.609093787363245,-0.793098202113394,0.));
#7805=DIRECTION('',(1.22464679914735E-16,-1.43058875937861E-30,-1.));
#7806=DIRECTION('center_axis',(0.,0.,-1.));
#7807=DIRECTION('ref_axis',(1.,-1.15591790427867E-14,0.));
#7808=DIRECTION('center_axis',(0.,0.,-1.));
#7809=DIRECTION('ref_axis',(1.,0.,0.));
#7810=DIRECTION('center_axis',(0.,0.,1.));
#7811=DIRECTION('ref_axis',(1.,0.,0.));
#7812=DIRECTION('',(0.,0.,-1.));
#7813=DIRECTION('center_axis',(0.,0.,1.));
#7814=DIRECTION('ref_axis',(1.,0.,0.));
#7815=DIRECTION('center_axis',(0.,0.,-1.));
#7816=DIRECTION('ref_axis',(1.,0.,0.));
#7817=DIRECTION('center_axis',(0.,0.,-1.));
#7818=DIRECTION('ref_axis',(1.,0.,0.));
#7819=DIRECTION('',(0.,0.,-1.));
#7820=DIRECTION('center_axis',(0.,0.,-1.));
#7821=DIRECTION('ref_axis',(1.,0.,0.));
#7822=DIRECTION('center_axis',(0.,0.,1.));
#7823=DIRECTION('ref_axis',(1.,0.,0.));
#7824=DIRECTION('center_axis',(0.,0.,1.));
#7825=DIRECTION('ref_axis',(1.,0.,0.));
#7826=DIRECTION('center_axis',(0.,0.,-1.));
#7827=DIRECTION('ref_axis',(1.,0.,0.));
#7828=DIRECTION('center_axis',(0.,0.,-1.));
#7829=DIRECTION('ref_axis',(1.,0.,0.));
#7830=DIRECTION('',(0.5,-0.866025403784439,0.));
#7831=DIRECTION('center_axis',(0.,0.,1.));
#7832=DIRECTION('ref_axis',(1.,0.,0.));
#7833=DIRECTION('',(-0.5,-0.866025403784438,0.));
#7834=DIRECTION('center_axis',(0.,0.,-1.));
#7835=DIRECTION('ref_axis',(1.,0.,0.));
#7836=DIRECTION('',(-1.,0.,0.));
#7837=DIRECTION('center_axis',(0.,0.,1.));
#7838=DIRECTION('ref_axis',(1.,0.,0.));
#7839=DIRECTION('',(-0.5,0.866025403784439,0.));
#7840=DIRECTION('',(0.5,0.866025403784438,0.));
#7841=DIRECTION('center_axis',(0.,0.,1.));
#7842=DIRECTION('ref_axis',(1.,0.,0.));
#7843=DIRECTION('',(1.,0.,0.));
#7844=DIRECTION('center_axis',(0.,0.,-1.));
#7845=DIRECTION('ref_axis',(1.,0.,0.));
#7846=DIRECTION('center_axis',(0.,0.,-1.));
#7847=DIRECTION('ref_axis',(1.,0.,0.));
#7848=DIRECTION('center_axis',(0.,0.,-1.));
#7849=DIRECTION('ref_axis',(1.,-1.15591790427867E-14,0.));
#7850=DIRECTION('center_axis',(0.,0.,1.));
#7851=DIRECTION('ref_axis',(1.,0.,0.));
#7852=DIRECTION('center_axis',(0.,0.,1.));
#7853=DIRECTION('ref_axis',(1.,0.,0.));
#7854=DIRECTION('center_axis',(0.,0.,1.));
#7855=DIRECTION('ref_axis',(1.,0.,0.));
#7856=DIRECTION('center_axis',(0.,0.,-1.));
#7857=DIRECTION('ref_axis',(1.,-1.81322775704035E-14,0.));
#7858=DIRECTION('center_axis',(0.,0.,-1.));
#7859=DIRECTION('ref_axis',(1.,-1.81324693622859E-14,0.));
#7860=DIRECTION('center_axis',(0.,0.,-1.));
#7861=DIRECTION('ref_axis',(1.,-2.31183580855735E-14,0.));
#7862=DIRECTION('center_axis',(0.,0.,-1.));
#7863=DIRECTION('ref_axis',(1.,0.,0.));
#7864=DIRECTION('center_axis',(0.,0.,-1.));
#7865=DIRECTION('ref_axis',(1.,0.,0.));
#7866=DIRECTION('center_axis',(0.,0.,-1.));
#7867=DIRECTION('ref_axis',(1.,0.,0.));
#7868=DIRECTION('center_axis',(0.,0.,-1.));
#7869=DIRECTION('ref_axis',(1.,0.,0.));
#7870=DIRECTION('center_axis',(0.,0.,-1.));
#7871=DIRECTION('ref_axis',(1.,0.,0.));
#7872=DIRECTION('center_axis',(0.,0.,-1.));
#7873=DIRECTION('ref_axis',(1.,0.,0.));
#7874=DIRECTION('',(0.,0.,-1.));
#7875=DIRECTION('center_axis',(0.,0.,1.));
#7876=DIRECTION('ref_axis',(1.,0.,0.));
#7877=DIRECTION('center_axis',(0.,0.,-1.));
#7878=DIRECTION('ref_axis',(1.,0.,0.));
#7879=DIRECTION('center_axis',(0.,0.,-1.));
#7880=DIRECTION('ref_axis',(1.,0.,0.));
#7881=DIRECTION('',(0.,0.,-1.));
#7882=DIRECTION('center_axis',(0.,0.,1.));
#7883=DIRECTION('ref_axis',(1.,0.,0.));
#7884=DIRECTION('center_axis',(0.,0.,-1.));
#7885=DIRECTION('ref_axis',(1.,0.,0.));
#7886=DIRECTION('center_axis',(0.,0.,-1.));
#7887=DIRECTION('ref_axis',(1.,0.,0.));
#7888=DIRECTION('',(0.,0.,-1.));
#7889=DIRECTION('center_axis',(0.,0.,1.));
#7890=DIRECTION('ref_axis',(1.,0.,0.));
#7891=DIRECTION('center_axis',(0.,0.,-1.));
#7892=DIRECTION('ref_axis',(1.,0.,0.));
#7893=DIRECTION('center_axis',(0.,0.,-1.));
#7894=DIRECTION('ref_axis',(1.,0.,0.));
#7895=DIRECTION('',(0.,0.,-1.));
#7896=DIRECTION('center_axis',(0.,0.,1.));
#7897=DIRECTION('ref_axis',(1.,0.,0.));
#7898=DIRECTION('center_axis',(0.,0.,1.));
#7899=DIRECTION('ref_axis',(1.,0.,0.));
#7900=DIRECTION('center_axis',(0.,0.,1.));
#7901=DIRECTION('ref_axis',(1.,0.,0.));
#7902=DIRECTION('center_axis',(0.,0.,1.));
#7903=DIRECTION('ref_axis',(1.,0.,0.));
#7904=DIRECTION('center_axis',(0.,0.,1.));
#7905=DIRECTION('ref_axis',(1.,0.,0.));
#7906=DIRECTION('',(0.,0.,-1.));
#7907=DIRECTION('center_axis',(0.,0.,1.));
#7908=DIRECTION('ref_axis',(1.,0.,0.));
#7909=DIRECTION('center_axis',(0.,0.,1.));
#7910=DIRECTION('ref_axis',(1.,0.,0.));
#7911=DIRECTION('center_axis',(0.,0.,-1.));
#7912=DIRECTION('ref_axis',(1.,0.,0.));
#7913=DIRECTION('center_axis',(0.,0.,1.));
#7914=DIRECTION('ref_axis',(1.,0.,0.));
#7915=DIRECTION('',(0.,0.,-1.));
#7916=DIRECTION('center_axis',(-0.866025403784438,0.5,0.));
#7917=DIRECTION('ref_axis',(-0.5,-0.866025403784438,0.));
#7918=DIRECTION('',(0.,0.,-1.));
#7919=DIRECTION('',(0.,0.,1.));
#7920=DIRECTION('',(-0.5,-0.866025403784438,0.));
#7921=DIRECTION('center_axis',(0.866025403784438,-0.5,0.));
#7922=DIRECTION('ref_axis',(0.5,0.866025403784438,0.));
#7923=DIRECTION('',(0.,0.,1.));
#7924=DIRECTION('',(0.5,0.866025403784438,0.));
#7925=DIRECTION('',(0.,0.,-1.));
#7926=DIRECTION('center_axis',(0.866025403784439,0.5,0.));
#7927=DIRECTION('ref_axis',(-0.5,0.866025403784439,0.));
#7928=DIRECTION('',(0.,0.,-1.));
#7929=DIRECTION('',(0.,0.,1.));
#7930=DIRECTION('',(-0.5,0.866025403784439,0.));
#7931=DIRECTION('center_axis',(-0.866025403784439,-0.5,0.));
#7932=DIRECTION('ref_axis',(0.5,-0.866025403784439,0.));
#7933=DIRECTION('',(0.,0.,1.));
#7934=DIRECTION('',(0.5,-0.866025403784439,0.));
#7935=DIRECTION('',(0.,0.,-1.));
#7936=DIRECTION('center_axis',(0.,0.,1.));
#7937=DIRECTION('ref_axis',(1.,0.,0.));
#7938=DIRECTION('',(0.,0.,-1.));
#7939=DIRECTION('center_axis',(0.,0.,-1.));
#7940=DIRECTION('ref_axis',(1.,0.,0.));
#7941=DIRECTION('',(0.,0.,1.));
#7942=DIRECTION('center_axis',(0.,0.,-1.));
#7943=DIRECTION('ref_axis',(1.,0.,0.));
#7944=DIRECTION('',(0.,0.,-1.));
#7945=DIRECTION('center_axis',(0.,0.,-1.));
#7946=DIRECTION('ref_axis',(1.,0.,0.));
#7947=DIRECTION('center_axis',(0.,0.,1.));
#7948=DIRECTION('ref_axis',(1.,0.,0.));
#7949=DIRECTION('',(1.,0.,0.));
#7950=DIRECTION('center_axis',(0.,0.,1.));
#7951=DIRECTION('ref_axis',(1.,0.,0.));
#7952=DIRECTION('center_axis',(0.,0.,1.));
#7953=DIRECTION('ref_axis',(1.,0.,0.));
#7954=DIRECTION('center_axis',(0.,0.,1.));
#7955=DIRECTION('ref_axis',(1.,0.,0.));
#7956=DIRECTION('',(-1.,0.,0.));
#7957=DIRECTION('center_axis',(0.,0.,-1.));
#7958=DIRECTION('ref_axis',(1.,0.,0.));
#7959=DIRECTION('center_axis',(0.,0.,1.));
#7960=DIRECTION('ref_axis',(1.,0.,0.));
#7961=DIRECTION('',(0.,0.,1.));
#7962=DIRECTION('center_axis',(0.,0.,1.));
#7963=DIRECTION('ref_axis',(-1.,-1.22464679914735E-16,0.));
#7964=DIRECTION('center_axis',(0.,0.,1.));
#7965=DIRECTION('ref_axis',(1.,0.,0.));
#7966=DIRECTION('',(0.,0.,-1.));
#7967=DIRECTION('center_axis',(0.,0.,1.));
#7968=DIRECTION('ref_axis',(1.,0.,0.));
#7969=DIRECTION('',(0.,0.,-1.));
#7970=DIRECTION('center_axis',(0.,1.,0.));
#7971=DIRECTION('ref_axis',(-1.,0.,0.));
#7972=DIRECTION('center_axis',(0.,0.,1.));
#7973=DIRECTION('ref_axis',(1.,0.,0.));
#7974=DIRECTION('center_axis',(0.,0.,1.));
#7975=DIRECTION('ref_axis',(1.,0.,0.));
#7976=DIRECTION('center_axis',(0.,-1.,0.));
#7977=DIRECTION('ref_axis',(1.,0.,0.));
#7978=DIRECTION('center_axis',(0.,0.,1.));
#7979=DIRECTION('ref_axis',(1.,0.,0.));
#7980=DIRECTION('',(0.,0.,-1.));
#9196=CARTESIAN_POINT('',(0.,0.,0.));
#9197=CARTESIAN_POINT('Origin',(0.,-7.4,-0.45));
#9198=CARTESIAN_POINT('',(-0.251358478231671,-7.40000989059476,-0.761258330249198));
#9199=CARTESIAN_POINT('',(-0.251584539328545,-7.40033372506469,-0.788741669750802));
#9200=CARTESIAN_POINT('',(-0.25175,-7.4,-0.45));
#9201=CARTESIAN_POINT('',(-0.191346599666506,-7.23640127966251,-0.8));
#9202=CARTESIAN_POINT('Ctrl Pts',(-0.251584539328545,-7.40033372506469,
-0.788741669750802));
#9203=CARTESIAN_POINT('Ctrl Pts',(-0.251071222245464,-7.34107836270979,
-0.792494446500535));
#9204=CARTESIAN_POINT('Ctrl Pts',(-0.229922182808405,-7.28151964396956,
-0.796247223250268));
#9205=CARTESIAN_POINT('Ctrl Pts',(-0.191346599666506,-7.23640127966251,
-0.8));
#9206=CARTESIAN_POINT('',(0.191702374352699,-7.23617294219443,-0.8));
#9207=CARTESIAN_POINT('Origin',(0.,-7.4,-0.8));
#9208=CARTESIAN_POINT('Ctrl Pts',(0.191704041017362,-7.23617187252308,-0.8));
#9209=CARTESIAN_POINT('Ctrl Pts',(0.140332563765971,-7.17646166153928,-0.795000212253756));
#9210=CARTESIAN_POINT('Ctrl Pts',(0.0585928763053871,-7.14242248557627,
-0.790000424507512));
#9211=CARTESIAN_POINT('Ctrl Pts',(-0.0199179743947309,-7.14865374913574,
-0.785000636761267));
#9212=CARTESIAN_POINT('Ctrl Pts',(-0.102096219979331,-7.15517608716323,
-0.779767299182859));
#9213=CARTESIAN_POINT('Ctrl Pts',(-0.180736932942895,-7.20581895652833,
-0.77453396160445));
#9214=CARTESIAN_POINT('Ctrl Pts',(-0.220629120750179,-7.27793230721061,
-0.769300624026042));
#9215=CARTESIAN_POINT('Ctrl Pts',(-0.241063798043618,-7.314872197719,-0.766619859433761));
#9216=CARTESIAN_POINT('Ctrl Pts',(-0.251330955357681,-7.35744589098191,
-0.763939094841479));
#9217=CARTESIAN_POINT('Ctrl Pts',(-0.251358478231671,-7.40000989059476,
-0.761258330249198));
#9218=CARTESIAN_POINT('Origin',(0.,-7.4,-0.45));
#9219=CARTESIAN_POINT('',(-0.252017165498346,-7.40015401716005,-0.661258330249198));
#9220=CARTESIAN_POINT('',(-0.252073448596348,-7.39987961136196,-0.688741669750803));
#9221=CARTESIAN_POINT('',(-0.25175,-7.4,-0.45));
#9222=CARTESIAN_POINT('Ctrl Pts',(-0.252073448596348,-7.39987961136196,
-0.688741669750803));
#9223=CARTESIAN_POINT('Ctrl Pts',(-0.25211567655556,-7.3927435289656,-0.689194416785009));
#9224=CARTESIAN_POINT('Ctrl Pts',(-0.251838292098126,-7.38561079836488,
-0.689647163819216));
#9225=CARTESIAN_POINT('Ctrl Pts',(-0.251230519881648,-7.37850635975571,
-0.690099910853423));
#9226=CARTESIAN_POINT('Ctrl Pts',(-0.244205234370541,-7.29638561077722,
-0.695333248431831));
#9227=CARTESIAN_POINT('Ctrl Pts',(-0.193036097579369,-7.21804501839796,
-0.700566586010239));
#9228=CARTESIAN_POINT('Ctrl Pts',(-0.12066406959885,-7.17860007027604,-0.705799923588648));
#9229=CARTESIAN_POINT('Ctrl Pts',(-0.0482920416183288,-7.13915512215413,
-0.711033261167056));
#9230=CARTESIAN_POINT('Ctrl Pts',(0.0452828775515399,-7.13860581828957,
-0.716266598745465));
#9231=CARTESIAN_POINT('Ctrl Pts',(0.118103971990326,-7.17721638163908,-0.721499936323874));
#9232=CARTESIAN_POINT('Ctrl Pts',(0.190925066429111,-7.21582694498859,-0.726733273902282));
#9233=CARTESIAN_POINT('Ctrl Pts',(0.242992336136814,-7.29359737555218,-0.73196661148069));
#9234=CARTESIAN_POINT('Ctrl Pts',(0.250965104406924,-7.37562272577954,-0.737199949059099));
#9235=CARTESIAN_POINT('Ctrl Pts',(0.258937872677034,-7.4576480760069,-0.742433286637507));
#9236=CARTESIAN_POINT('Ctrl Pts',(0.22281613950955,-7.54392834589802,-0.747666624215916));
#9237=CARTESIAN_POINT('Ctrl Pts',(0.158787402101112,-7.59585258416295,-0.752899961794324));
#9238=CARTESIAN_POINT('Ctrl Pts',(0.0947586646926728,-7.64777682242788,
-0.758133299372733));
#9239=CARTESIAN_POINT('Ctrl Pts',(0.0028229230432783,-7.66534502906661,
-0.763366636951141));
#9240=CARTESIAN_POINT('Ctrl Pts',(-0.0757847496475859,-7.64053050273058,
-0.76859997452955));
#9241=CARTESIAN_POINT('Ctrl Pts',(-0.154392422338449,-7.61571597639454,
-0.773833312107958));
#9242=CARTESIAN_POINT('Ctrl Pts',(-0.219672026070782,-7.54851871708374,
-0.779066649686366));
#9243=CARTESIAN_POINT('Ctrl Pts',(-0.242359215388134,-7.46941970437215,
-0.784299987264775));
#9244=CARTESIAN_POINT('Ctrl Pts',(-0.248777636388646,-7.44704184358004,
-0.78578054809345));
#9245=CARTESIAN_POINT('Ctrl Pts',(-0.251787055283152,-7.42371139292034,
-0.787261108922126));
#9246=CARTESIAN_POINT('Ctrl Pts',(-0.251584539328545,-7.40033372506469,
-0.788741669750802));
#9247=CARTESIAN_POINT('Ctrl Pts',(-0.251358478231671,-7.40000989059476,
-0.761258330249198));
#9248=CARTESIAN_POINT('Ctrl Pts',(-0.251384684988075,-7.44053852033946,
-0.758705757263071));
#9249=CARTESIAN_POINT('Ctrl Pts',(-0.242127141836486,-7.4810583613502,-0.756153184276944));
#9250=CARTESIAN_POINT('Ctrl Pts',(-0.223523592831821,-7.51669741987088,
-0.753600611290817));
#9251=CARTESIAN_POINT('Ctrl Pts',(-0.185382214455175,-7.58976534984939,
-0.748367273712408));
#9252=CARTESIAN_POINT('Ctrl Pts',(-0.107955795050881,-7.64231737780695,
-0.743133936134));
#9253=CARTESIAN_POINT('Ctrl Pts',(-0.0259706133934279,-7.65080523818006,
-0.737900598555591));
#9254=CARTESIAN_POINT('Ctrl Pts',(0.0560145682640249,-7.65929309855318,
-0.732667260977183));
#9255=CARTESIAN_POINT('Ctrl Pts',(0.142558512174636,-7.62371679134186,-0.727433923398774));
#9256=CARTESIAN_POINT('Ctrl Pts',(0.194864662021149,-7.56002033893795,-0.722200585820366));
#9257=CARTESIAN_POINT('Ctrl Pts',(0.247170811867661,-7.49632388653404,-0.716967248241958));
#9258=CARTESIAN_POINT('Ctrl Pts',(0.265239167650075,-7.40450728893754,-0.71173391066355));
#9259=CARTESIAN_POINT('Ctrl Pts',(0.240965802115707,-7.32574032208645,-0.706500573085141));
#9260=CARTESIAN_POINT('Ctrl Pts',(0.216692436581339,-7.24697335523537,-0.701267235506732));
#9261=CARTESIAN_POINT('Ctrl Pts',(0.150077349730189,-7.1812560191297,-0.696033897928324));
#9262=CARTESIAN_POINT('Ctrl Pts',(0.0709891696492391,-7.15805132892677,
-0.690800560349915));
#9263=CARTESIAN_POINT('Ctrl Pts',(-0.00809901043171256,-7.13484663872384,
-0.685567222771507));
#9264=CARTESIAN_POINT('Ctrl Pts',(-0.0996602837424652,-7.15415459442365,
-0.680333885193099));
#9265=CARTESIAN_POINT('Ctrl Pts',(-0.162643425289155,-7.20731920825571,
-0.675100547614691));
#9266=CARTESIAN_POINT('Ctrl Pts',(-0.218173720095525,-7.2541928097761,-0.670486475159527));
#9267=CARTESIAN_POINT('Ctrl Pts',(-0.251489074403517,-7.32738456435463,
-0.665872402704362));
#9268=CARTESIAN_POINT('Ctrl Pts',(-0.252017165498346,-7.40015401716005,
-0.661258330249198));
#9269=CARTESIAN_POINT('Origin',(0.,-7.4,-0.45));
#9270=CARTESIAN_POINT('',(-0.251711685022834,-7.3997833335225,-0.561258330249198));
#9271=CARTESIAN_POINT('',(-0.25137527833601,-7.39994331833701,-0.588741669750803));
#9272=CARTESIAN_POINT('',(-0.25175,-7.4,-0.45));
#9273=CARTESIAN_POINT('Ctrl Pts',(-0.25137527833601,-7.39994331833701,-0.588741669750803));
#9274=CARTESIAN_POINT('Ctrl Pts',(-0.251453232926026,-7.36206606061581,
-0.591127724647892));
#9275=CARTESIAN_POINT('Ctrl Pts',(-0.243409884741493,-7.32422023730893,
-0.593513779544982));
#9276=CARTESIAN_POINT('Ctrl Pts',(-0.227072436774608,-7.29037848576413,
-0.595899834442071));
#9277=CARTESIAN_POINT('Ctrl Pts',(-0.191239489056313,-7.21615332426654,
-0.601133172020479));
#9278=CARTESIAN_POINT('Ctrl Pts',(-0.115507184704655,-7.16119003463128,
-0.606366509598888));
#9279=CARTESIAN_POINT('Ctrl Pts',(-0.0338304512848064,-7.15013153945356,
-0.611599847177296));
#9280=CARTESIAN_POINT('Ctrl Pts',(0.0478462821350425,-7.13907304427583,
-0.616833184755704));
#9281=CARTESIAN_POINT('Ctrl Pts',(0.135467444623083,-7.17191934355563,-0.622066522334113));
#9282=CARTESIAN_POINT('Ctrl Pts',(0.189747638705398,-7.23394390765325,-0.627299859912521));
#9283=CARTESIAN_POINT('Ctrl Pts',(0.244027832787713,-7.29596847175088,-0.63253319749093));
#9284=CARTESIAN_POINT('Ctrl Pts',(0.264967058464304,-7.38717130066634,-0.637766535069338));
#9285=CARTESIAN_POINT('Ctrl Pts',(0.243177171908073,-7.46666063157891,-0.642999872647747));
#9286=CARTESIAN_POINT('Ctrl Pts',(0.221387285351841,-7.54614996249148,-0.648233210226155));
#9287=CARTESIAN_POINT('Ctrl Pts',(0.156868286562786,-7.61392579540117,-0.653466547804563));
#9288=CARTESIAN_POINT('Ctrl Pts',(0.0785474602301629,-7.63960159378581,
-0.658699885382972));
#9289=CARTESIAN_POINT('Ctrl Pts',(0.000226633897540712,-7.66527739217044,
-0.66393322296138));
#9290=CARTESIAN_POINT('Ctrl Pts',(-0.0918960199786485,-7.64885315603003,
-0.669166560539789));
#9291=CARTESIAN_POINT('Ctrl Pts',(-0.156516629801222,-7.59769058517097,
-0.674399898118197));
#9292=CARTESIAN_POINT('Ctrl Pts',(-0.215546774837709,-7.55095419585892,
-0.679180488662399));
#9293=CARTESIAN_POINT('Ctrl Pts',(-0.251627560346938,-7.47523005089924,
-0.683961079206601));
#9294=CARTESIAN_POINT('Ctrl Pts',(-0.252073448596348,-7.39987961136196,
-0.688741669750803));
#9295=CARTESIAN_POINT('Ctrl Pts',(-0.252017165498346,-7.40015401716005,
-0.661258330249198));
#9296=CARTESIAN_POINT('Ctrl Pts',(-0.252088041801243,-7.40992057037261,
-0.660639065125953));
#9297=CARTESIAN_POINT('Ctrl Pts',(-0.25156832334334,-7.41967951669182,-0.660019800002709));
#9298=CARTESIAN_POINT('Ctrl Pts',(-0.250432450937044,-7.42936620955704,
-0.659400534879464));
#9299=CARTESIAN_POINT('Ctrl Pts',(-0.240833325255617,-7.51122732506196,
-0.654167197301056));
#9300=CARTESIAN_POINT('Ctrl Pts',(-0.187230064110134,-7.58792828410748,
-0.648933859722648));
#9301=CARTESIAN_POINT('Ctrl Pts',(-0.113656121528127,-7.62508004699099,
-0.643700522144239));
#9302=CARTESIAN_POINT('Ctrl Pts',(-0.0400821789461197,-7.66223180987451,
-0.638467184565831));
#9303=CARTESIAN_POINT('Ctrl Pts',(0.0534624450724112,-7.65983437659602,
-0.633233846987422));
#9304=CARTESIAN_POINT('Ctrl Pts',(0.125036656278963,-7.61896254712631,-0.628000509409014));
#9305=CARTESIAN_POINT('Ctrl Pts',(0.196610867485515,-7.5780907176566,-0.622767171830605));
#9306=CARTESIAN_POINT('Ctrl Pts',(0.246214665880088,-7.49874449199566,-0.617533834252197));
#9307=CARTESIAN_POINT('Ctrl Pts',(0.251607907559673,-7.41649918096761,-0.612300496673789));
#9308=CARTESIAN_POINT('Ctrl Pts',(0.257001149239257,-7.33425386993957,-0.60706715909538));
#9309=CARTESIAN_POINT('Ctrl Pts',(0.218183834203852,-7.24910947354443,-0.601833821516971));
#9310=CARTESIAN_POINT('Ctrl Pts',(0.152559913142665,-7.19924086556578,-0.596600483938563));
#9311=CARTESIAN_POINT('Ctrl Pts',(0.086935992081478,-7.14937225758713,-0.591367146360155));
#9312=CARTESIAN_POINT('Ctrl Pts',(-0.00549453500549198,-7.13477943802497,
-0.586133808781747));
#9313=CARTESIAN_POINT('Ctrl Pts',(-0.0832900084867264,-7.16200517980322,
-0.580900471203338));
#9314=CARTESIAN_POINT('Ctrl Pts',(-0.161085481967961,-7.18923092158147,
-0.57566713362493));
#9315=CARTESIAN_POINT('Ctrl Pts',(-0.22424590184346,-7.25827522470013,-0.570433796046521));
#9316=CARTESIAN_POINT('Ctrl Pts',(-0.244452985661471,-7.33818173858017,
-0.565200458468112));
#9317=CARTESIAN_POINT('Ctrl Pts',(-0.249526797809548,-7.35824552633334,
-0.563886415728474));
#9318=CARTESIAN_POINT('Ctrl Pts',(-0.251892549336989,-7.37899413924599,
-0.562572372988836));
#9319=CARTESIAN_POINT('Ctrl Pts',(-0.251711685022834,-7.3997833335225,-0.561258330249198));
#9320=CARTESIAN_POINT('Origin',(0.,-7.4,-0.45));
#9321=CARTESIAN_POINT('',(-0.251454207353971,-7.40014378921791,-0.461258330249198));
#9322=CARTESIAN_POINT('',(-0.251895011223093,-7.40019827523323,-0.488741669750802));
#9323=CARTESIAN_POINT('',(-0.25175,-7.4,-0.45));
#9324=CARTESIAN_POINT('Ctrl Pts',(-0.251895011223093,-7.40019827523323,
-0.488741669750802));
#9325=CARTESIAN_POINT('Ctrl Pts',(-0.251306428556441,-7.33199055382304,
-0.493061032510774));
#9326=CARTESIAN_POINT('Ctrl Pts',(-0.222557857907552,-7.26334536000167,
-0.497380395270746));
#9327=CARTESIAN_POINT('Ctrl Pts',(-0.173090828377879,-7.21664697959534,
-0.501699758030719));
#9328=CARTESIAN_POINT('Ctrl Pts',(-0.113156602216345,-7.16006724721073,
-0.506933095609127));
#9329=CARTESIAN_POINT('Ctrl Pts',(-0.0228082327120731,-7.13570484976218,
-0.512166433187536));
#9330=CARTESIAN_POINT('Ctrl Pts',(0.0574461554993007,-7.15448278304868,
-0.517399770765944));
#9331=CARTESIAN_POINT('Ctrl Pts',(0.137700543710675,-7.17326071633519,-0.522633108344353));
#9332=CARTESIAN_POINT('Ctrl Pts',(0.20786095062915,-7.23517898035675,-0.527866445922761));
#9333=CARTESIAN_POINT('Ctrl Pts',(0.236470620838672,-7.31247622838102,-0.533099783501169));
#9334=CARTESIAN_POINT('Ctrl Pts',(0.265080291048194,-7.38977347640529,-0.538333121079578));
#9335=CARTESIAN_POINT('Ctrl Pts',(0.252139224548762,-7.48244970843227,-0.543566458657986));
#9336=CARTESIAN_POINT('Ctrl Pts',(0.203449611448168,-7.54895308331631,-0.548799796236395));
#9337=CARTESIAN_POINT('Ctrl Pts',(0.154759998347575,-7.61545645820036,-0.554033133814803));
#9338=CARTESIAN_POINT('Ctrl Pts',(0.0703218386458203,-7.65578697594147,
-0.559266471393212));
#9339=CARTESIAN_POINT('Ctrl Pts',(-0.0120066154728626,-7.65186227152851,
-0.56449980897162));
#9340=CARTESIAN_POINT('Ctrl Pts',(-0.0943350695915468,-7.64793756711556,
-0.569733146550029));
#9341=CARTESIAN_POINT('Ctrl Pts',(-0.174553818127159,-7.59975764054855,
-0.574966484128437));
#9342=CARTESIAN_POINT('Ctrl Pts',(-0.216696396852498,-7.52892416058508,
-0.580199821706846));
#9343=CARTESIAN_POINT('Ctrl Pts',(-0.239624754282723,-7.49038605029967,
-0.583047104388165));
#9344=CARTESIAN_POINT('Ctrl Pts',(-0.251282255013556,-7.44514230351416,
-0.585894387069484));
#9345=CARTESIAN_POINT('Ctrl Pts',(-0.25137527833601,-7.39994331833701,-0.588741669750803));
#9346=CARTESIAN_POINT('Ctrl Pts',(-0.251711685022834,-7.3997833335225,-0.561258330249198));
#9347=CARTESIAN_POINT('Ctrl Pts',(-0.251172234857628,-7.46178967423907,
-0.557339035410427));
#9348=CARTESIAN_POINT('Ctrl Pts',(-0.227977979841335,-7.52415702852661,
-0.553419740571657));
#9349=CARTESIAN_POINT('Ctrl Pts',(-0.186412622838117,-7.56979132243042,
-0.549500445732887));
#9350=CARTESIAN_POINT('Ctrl Pts',(-0.130911428436227,-7.63072566775921,
-0.544267108154479));
#9351=CARTESIAN_POINT('Ctrl Pts',(-0.0426552918719249,-7.66182563377536,
-0.53903377057607));
#9352=CARTESIAN_POINT('Ctrl Pts',(0.038785725966995,-7.64914740004011,-0.533800432997662));
#9353=CARTESIAN_POINT('Ctrl Pts',(0.120226743805915,-7.63646916630487,-0.528567095419253));
#9354=CARTESIAN_POINT('Ctrl Pts',(0.194852642919453,-7.58001273281824,-0.523333757840845));
#9355=CARTESIAN_POINT('Ctrl Pts',(0.229204542838122,-7.50509061308471,-0.518100420262437));
#9356=CARTESIAN_POINT('Ctrl Pts',(0.263556442756791,-7.43016849335117,-0.512867082684028));
#9357=CARTESIAN_POINT('Ctrl Pts',(0.257634343480592,-7.33678068737074,-0.50763374510562));
#9358=CARTESIAN_POINT('Ctrl Pts',(0.214093446943169,-7.26679806554806,-0.502400407527211));
#9359=CARTESIAN_POINT('Ctrl Pts',(0.170552550405746,-7.19681544372539,-0.497167069948803));
#9360=CARTESIAN_POINT('Ctrl Pts',(0.0893928566070999,-7.15023800606048,
-0.491933732370394));
#9361=CARTESIAN_POINT('Ctrl Pts',(0.00700270341056665,-7.14794897033469,
-0.486700394791986));
#9362=CARTESIAN_POINT('Ctrl Pts',(-0.0753874497859666,-7.1456599346089,
-0.481467057213577));
#9363=CARTESIAN_POINT('Ctrl Pts',(-0.159008062380387,-7.18765930082222,
-0.476233719635169));
#9364=CARTESIAN_POINT('Ctrl Pts',(-0.206367431528416,-7.25511645158031,
-0.47100038205676));
#9365=CARTESIAN_POINT('Ctrl Pts',(-0.235754505003739,-7.29697444676534,
-0.46775303145424));
#9366=CARTESIAN_POINT('Ctrl Pts',(-0.251179709674751,-7.34863459471956,
-0.464505680851719));
#9367=CARTESIAN_POINT('Ctrl Pts',(-0.251454207353971,-7.40014378921791,
-0.461258330249198));
#9368=CARTESIAN_POINT('Origin',(0.,-7.4,-0.45));
#9369=CARTESIAN_POINT('',(-0.252147125090441,-7.40001476863366,-0.361258330249198));
#9370=CARTESIAN_POINT('',(-0.251847319535426,-7.39979207600155,-0.388741669750802));
#9371=CARTESIAN_POINT('',(-0.25175,-7.4,-0.45));
#9372=CARTESIAN_POINT('Ctrl Pts',(-0.251847319535426,-7.39979207600155,
-0.388741669750802));
#9373=CARTESIAN_POINT('Ctrl Pts',(-0.251989595225182,-7.38368773667891,
-0.389761002795249));
#9374=CARTESIAN_POINT('Ctrl Pts',(-0.250573880883256,-7.36760829714423,
-0.390780335839695));
#9375=CARTESIAN_POINT('Ctrl Pts',(-0.247508235120279,-7.35184983468962,
-0.391799668884141));
#9376=CARTESIAN_POINT('Ctrl Pts',(-0.231768963975402,-7.27094462496357,
-0.39703300646255));
#9377=CARTESIAN_POINT('Ctrl Pts',(-0.172539514683342,-7.19849997924377,
-0.402266344040958));
#9378=CARTESIAN_POINT('Ctrl Pts',(-0.0963756949442417,-7.16699680195703,
-0.407499681619367));
#9379=CARTESIAN_POINT('Ctrl Pts',(-0.0202118752051417,-7.13549362467028,
-0.412733019197775));
#9380=CARTESIAN_POINT('Ctrl Pts',(0.0728863149809975,-7.14493191581659,
-0.417966356776183));
#9381=CARTESIAN_POINT('Ctrl Pts',(0.141177855474435,-7.19107997225668,-0.423199694354592));
#9382=CARTESIAN_POINT('Ctrl Pts',(0.209469395967872,-7.23722802869677,-0.428433031933));
#9383=CARTESIAN_POINT('Ctrl Pts',(0.252954286768607,-7.32008585043064,-0.433666369511409));
#9384=CARTESIAN_POINT('Ctrl Pts',(0.252135868492745,-7.40250373569222,-0.438899707089817));
#9385=CARTESIAN_POINT('Ctrl Pts',(0.251317450216883,-7.48492162095379,-0.444133044668226));
#9386=CARTESIAN_POINT('Ctrl Pts',(0.206195722864424,-7.56689956974307,-0.449366382246634));
#9387=CARTESIAN_POINT('Ctrl Pts',(0.137001229345556,-7.61168237537139,-0.454599719825043));
#9388=CARTESIAN_POINT('Ctrl Pts',(0.0678067358266871,-7.65646518099971,
-0.459833057403451));
#9389=CARTESIAN_POINT('Ctrl Pts',(-0.0254605238585907,-7.66405284346707,
-0.465066394981859));
#9390=CARTESIAN_POINT('Ctrl Pts',(-0.100983726473419,-7.63104339814856,
-0.470299732560268));
#9391=CARTESIAN_POINT('Ctrl Pts',(-0.176506929088247,-7.59803395283005,
-0.475533070138676));
#9392=CARTESIAN_POINT('Ctrl Pts',(-0.234286074632624,-7.52442739972568,
-0.480766407717085));
#9393=CARTESIAN_POINT('Ctrl Pts',(-0.248415605995416,-7.44322558951315,
-0.485999745295493));
#9394=CARTESIAN_POINT('Ctrl Pts',(-0.25088325415845,-7.42904412144736,-0.48691372011393));
#9395=CARTESIAN_POINT('Ctrl Pts',(-0.252019554996279,-7.41463099210748,
-0.487827694932366));
#9396=CARTESIAN_POINT('Ctrl Pts',(-0.251895011223093,-7.40019827523323,
-0.488741669750802));
#9397=CARTESIAN_POINT('Ctrl Pts',(-0.251454207353971,-7.40014378921791,
-0.461258330249198));
#9398=CARTESIAN_POINT('Ctrl Pts',(-0.25162208230268,-7.43164534292534,-0.45927234327331));
#9399=CARTESIAN_POINT('Ctrl Pts',(-0.246123294961887,-7.46309043707242,
-0.457286356297423));
#9400=CARTESIAN_POINT('Ctrl Pts',(-0.234685910778123,-7.49220240059875,
-0.455300369321535));
#9401=CARTESIAN_POINT('Ctrl Pts',(-0.204546895178166,-7.56891626355623,
-0.450067031743127));
#9402=CARTESIAN_POINT('Ctrl Pts',(-0.133170738276618,-7.62942905416833,
-0.444833694164718));
#9403=CARTESIAN_POINT('Ctrl Pts',(-0.0525592823773014,-7.64660957247344,
-0.43960035658631));
#9404=CARTESIAN_POINT('Ctrl Pts',(0.0280521735220159,-7.66379009077855,
-0.434367019007901));
#9405=CARTESIAN_POINT('Ctrl Pts',(0.117898928419101,-7.63763833677668,-0.429133681429493));
#9406=CARTESIAN_POINT('Ctrl Pts',(0.176697758771395,-7.5798795748334,-0.423900343851084));
#9407=CARTESIAN_POINT('Ctrl Pts',(0.235496589123688,-7.52212081289012,-0.418667006272676));
#9408=CARTESIAN_POINT('Ctrl Pts',(0.263247494931189,-7.43275504300543,-0.413433668694268));
#9409=CARTESIAN_POINT('Ctrl Pts',(0.247508224463957,-7.3518498367627,-0.408200331115859));
#9410=CARTESIAN_POINT('Ctrl Pts',(0.231768953996723,-7.27094463051998,-0.402966993537451));
#9411=CARTESIAN_POINT('Ctrl Pts',(0.172539507254754,-7.19849998791922,-0.397733655959042));
#9412=CARTESIAN_POINT('Ctrl Pts',(0.096375690794842,-7.16699681198883,-0.392500318380634));
#9413=CARTESIAN_POINT('Ctrl Pts',(0.0202118743349312,-7.13549363605845,
-0.387266980802225));
#9414=CARTESIAN_POINT('Ctrl Pts',(-0.072886311842922,-7.14493192679844,
-0.382033643223817));
#9415=CARTESIAN_POINT('Ctrl Pts',(-0.141177849396106,-7.19107998125163,
-0.376800305645409));
#9416=CARTESIAN_POINT('Ctrl Pts',(-0.208781959935431,-7.23676350641753,
-0.371619647180005));
#9417=CARTESIAN_POINT('Ctrl Pts',(-0.252076318944627,-7.3184214692473,-0.366438988714602));
#9418=CARTESIAN_POINT('Ctrl Pts',(-0.252147125090441,-7.40001476863366,
-0.361258330249198));
#9419=CARTESIAN_POINT('Origin',(0.,-7.4,-0.45));
#9420=CARTESIAN_POINT('',(-0.251485858071088,-7.39983751670088,-0.261258330249198));
#9421=CARTESIAN_POINT('',(-0.251389279889816,-7.40008150716695,-0.288741669750802));
#9422=CARTESIAN_POINT('',(-0.25175,-7.4,-0.45));
#9423=CARTESIAN_POINT('Ctrl Pts',(-0.251389279889816,-7.40008150716695,
-0.288741669750802));
#9424=CARTESIAN_POINT('Ctrl Pts',(-0.251250058629027,-7.35321657136339,
-0.291694310658131));
#9425=CARTESIAN_POINT('Ctrl Pts',(-0.238659163200998,-7.30628214770086,
-0.29464695156546));
#9426=CARTESIAN_POINT('Ctrl Pts',(-0.214093456160902,-7.26679805981303,
-0.297599592472789));
#9427=CARTESIAN_POINT('Ctrl Pts',(-0.170552557748908,-7.1968154349772,-0.302832930051197));
#9428=CARTESIAN_POINT('Ctrl Pts',(-0.0893928604558538,-7.15023799530713,
-0.308066267629606));
#9429=CARTESIAN_POINT('Ctrl Pts',(-0.00700270371203047,-7.14794895948283,
-0.313299605208015));
#9430=CARTESIAN_POINT('Ctrl Pts',(0.0753874530317917,-7.14565992365854,
-0.318532942786423));
#9431=CARTESIAN_POINT('Ctrl Pts',(0.159008069226383,-7.18765929168002,-0.323766280364831));
#9432=CARTESIAN_POINT('Ctrl Pts',(0.206367440413426,-7.25511644534241,-0.32899961794324));
#9433=CARTESIAN_POINT('Ctrl Pts',(0.253726811600469,-7.32257359900481,-0.334232955521648));
#9434=CARTESIAN_POINT('Ctrl Pts',(0.264824937779963,-7.41548853830811,-0.339466293100057));
#9435=CARTESIAN_POINT('Ctrl Pts',(0.234685920882397,-7.49220240456848,-0.344699630678465));
#9436=CARTESIAN_POINT('Ctrl Pts',(0.204546903984831,-7.56891627082884,-0.349932968256874));
#9437=CARTESIAN_POINT('Ctrl Pts',(0.133170744010206,-7.62942906404626,-0.355166305835282));
#9438=CARTESIAN_POINT('Ctrl Pts',(0.0525592846402059,-7.64660958309106,
-0.36039964341369));
#9439=CARTESIAN_POINT('Ctrl Pts',(-0.0280521747297935,-7.66379010213587,
-0.365632980992099));
#9440=CARTESIAN_POINT('Ctrl Pts',(-0.117898933495167,-7.63763834700807,
-0.370866318570508));
#9441=CARTESIAN_POINT('Ctrl Pts',(-0.176697766379008,-7.57987958257802,
-0.376099656148916));
#9442=CARTESIAN_POINT('Ctrl Pts',(-0.224043947406287,-7.53337088874017,
-0.380313660682878));
#9443=CARTESIAN_POINT('Ctrl Pts',(-0.251259140426578,-7.46636870597724,
-0.38452766521684));
#9444=CARTESIAN_POINT('Ctrl Pts',(-0.251847319535426,-7.39979207600155,
-0.388741669750802));
#9445=CARTESIAN_POINT('Ctrl Pts',(-0.252147125090441,-7.40001476863366,
-0.361258330249198));
#9446=CARTESIAN_POINT('Ctrl Pts',(-0.252147845077095,-7.40084444360018,
-0.361205651136193));
#9447=CARTESIAN_POINT('Ctrl Pts',(-0.252144095887885,-7.40167411188071,
-0.361152972023188));
#9448=CARTESIAN_POINT('Ctrl Pts',(-0.252135857637182,-7.40250373558439,
-0.361100292910183));
#9449=CARTESIAN_POINT('Ctrl Pts',(-0.251317439396557,-7.48492161729753,
-0.355866955331775));
#9450=CARTESIAN_POINT('Ctrl Pts',(-0.206195713986794,-7.56689956255742,
-0.350633617753366));
#9451=CARTESIAN_POINT('Ctrl Pts',(-0.137001223447051,-7.61168236625759,
-0.345400280174958));
#9452=CARTESIAN_POINT('Ctrl Pts',(-0.067806732907307,-7.65646516995776,
-0.340166942596549));
#9453=CARTESIAN_POINT('Ctrl Pts',(0.025460522762417,-7.6640528320982,-0.334933605018141));
#9454=CARTESIAN_POINT('Ctrl Pts',(0.100983722125631,-7.631043388201,-0.329700267439732));
#9455=CARTESIAN_POINT('Ctrl Pts',(0.176506921488845,-7.59803394430381,-0.324466929861324));
#9456=CARTESIAN_POINT('Ctrl Pts',(0.234286064545549,-7.52442739436897,-0.319233592282915));
#9457=CARTESIAN_POINT('Ctrl Pts',(0.248415595300016,-7.44322558765233,-0.314000254704507));
#9458=CARTESIAN_POINT('Ctrl Pts',(0.262545126054484,-7.36202378093569,-0.308766917126099));
#9459=CARTESIAN_POINT('Ctrl Pts',(0.233025044506715,-7.27322671743724,-0.30353357954769));
#9460=CARTESIAN_POINT('Ctrl Pts',(0.17309082092558,-7.21664698748904,-0.298300241969282));
#9461=CARTESIAN_POINT('Ctrl Pts',(0.113156597344446,-7.16006725754084,-0.293066904390873));
#9462=CARTESIAN_POINT('Ctrl Pts',(0.0228082317299446,-7.13570486114289,
-0.287833566812465));
#9463=CARTESIAN_POINT('Ctrl Pts',(-0.0574461530260513,-7.15448279362015,
-0.282600229234056));
#9464=CARTESIAN_POINT('Ctrl Pts',(-0.137700537782047,-7.17326072609741,
-0.277366891655648));
#9465=CARTESIAN_POINT('Ctrl Pts',(-0.207860941679538,-7.23517898744989,
-0.272133554077239));
#9466=CARTESIAN_POINT('Ctrl Pts',(-0.236470610657442,-7.31247623214764,
-0.266900216498831));
#9467=CARTESIAN_POINT('Ctrl Pts',(-0.246751653146716,-7.34025342375566,
-0.265019587748953));
#9468=CARTESIAN_POINT('Ctrl Pts',(-0.251666983719407,-7.37001660175744,
-0.263138958999076));
#9469=CARTESIAN_POINT('Ctrl Pts',(-0.251485858071088,-7.39983751670088,
-0.261258330249198));
#9470=CARTESIAN_POINT('Origin',(0.,-7.4,-0.45));
#9471=CARTESIAN_POINT('',(-0.2516645197469,-7.40021351101923,-0.161258330249198));
#9472=CARTESIAN_POINT('',(-0.252102603566075,-7.4000936994049,-0.188741669750802));
#9473=CARTESIAN_POINT('',(-0.25175,-7.4,-0.45));
#9474=CARTESIAN_POINT('Ctrl Pts',(-0.252102603566075,-7.4000936994049,-0.188741669750802));
#9475=CARTESIAN_POINT('Ctrl Pts',(-0.2517296574347,-7.32310553688027,-0.193627618521014));
#9476=CARTESIAN_POINT('Ctrl Pts',(-0.213827729289536,-7.24579919004338,
-0.198513567291226));
#9477=CARTESIAN_POINT('Ctrl Pts',(-0.152559919713999,-7.19924085691687,
-0.203399516061437));
#9478=CARTESIAN_POINT('Ctrl Pts',(-0.0869359958298059,-7.14937224678642,
-0.208632853639846));
#9479=CARTESIAN_POINT('Ctrl Pts',(0.00549453524232928,-7.13477942660635,
-0.213866191218254));
#9480=CARTESIAN_POINT('Ctrl Pts',(0.0832900120743056,-7.16200516955927,
-0.219099528796662));
#9481=CARTESIAN_POINT('Ctrl Pts',(0.161085488906282,-7.18923091251219,-0.224332866375071));
#9482=CARTESIAN_POINT('Ctrl Pts',(0.224245911498099,-7.2582752185981,-0.229566203953479));
#9483=CARTESIAN_POINT('Ctrl Pts',(0.244452996185411,-7.33818173591718,-0.234799541531888));
#9484=CARTESIAN_POINT('Ctrl Pts',(0.264660080872723,-7.41808825323625,-0.240032879110296));
#9485=CARTESIAN_POINT('Ctrl Pts',(0.241913827655531,-7.50885698178848,-0.245266216688705));
#9486=CARTESIAN_POINT('Ctrl Pts',(0.186412630864449,-7.56979132974143,-0.250499554267113));
#9487=CARTESIAN_POINT('Ctrl Pts',(0.130911434073366,-7.63072567769439,-0.255732891845521));
#9488=CARTESIAN_POINT('Ctrl Pts',(0.0426552937083935,-7.66182564504807,
-0.26096622942393));
#9489=CARTESIAN_POINT('Ctrl Pts',(-0.0387857276371238,-7.64914741076662,
-0.266199567002338));
#9490=CARTESIAN_POINT('Ctrl Pts',(-0.120226748982641,-7.63646917648517,
-0.271432904580747));
#9491=CARTESIAN_POINT('Ctrl Pts',(-0.194852651308702,-7.5800127405686,-0.276666242159156));
#9492=CARTESIAN_POINT('Ctrl Pts',(-0.229204552706265,-7.50509061760952,
-0.281899579737564));
#9493=CARTESIAN_POINT('Ctrl Pts',(-0.244175164861291,-7.47243943968284,
-0.284180276408643));
#9494=CARTESIAN_POINT('Ctrl Pts',(-0.251496818014495,-7.43628120311108,
-0.286460973079723));
#9495=CARTESIAN_POINT('Ctrl Pts',(-0.251389279889816,-7.40008150716695,
-0.288741669750802));
#9496=CARTESIAN_POINT('Ctrl Pts',(-0.251485858071088,-7.39983751670088,
-0.261258330249198));
#9497=CARTESIAN_POINT('Ctrl Pts',(-0.251162954595198,-7.453001037046,-0.257905621420667));
#9498=CARTESIAN_POINT('Ctrl Pts',(-0.234642333184093,-7.5063480587605,-0.254552912592136));
#9499=CARTESIAN_POINT('Ctrl Pts',(-0.20344960268904,-7.54895307690641,-0.251200203763606));
#9500=CARTESIAN_POINT('Ctrl Pts',(-0.154759991684416,-7.61545644892441,
-0.245966866185197));
#9501=CARTESIAN_POINT('Ctrl Pts',(-0.0703218356168507,-7.65578696491737,
-0.240733528606789));
#9502=CARTESIAN_POINT('Ctrl Pts',(0.0120066149565192,-7.65186226067865,
-0.23550019102838));
#9503=CARTESIAN_POINT('Ctrl Pts',(0.0943350655298891,-7.64793755643993,
-0.230266853449972));
#9504=CARTESIAN_POINT('Ctrl Pts',(0.174553810609064,-7.59975763196954,-0.225033515871563));
#9505=CARTESIAN_POINT('Ctrl Pts',(0.216696387521491,-7.52892415504588,-0.219800178293155));
#9506=CARTESIAN_POINT('Ctrl Pts',(0.258838964433917,-7.45809067812223,-0.214566840714747));
#9507=CARTESIAN_POINT('Ctrl Pts',(0.262905373179595,-7.36460364874532,-0.209333503136338));
#9508=CARTESIAN_POINT('Ctrl Pts',(0.227072427000858,-7.29037849046193,-0.20410016555793));
#9509=CARTESIAN_POINT('Ctrl Pts',(0.191239480822121,-7.21615333217855,-0.198866827979521));
#9510=CARTESIAN_POINT('Ctrl Pts',(0.115507179718968,-7.1611900449887,-0.193633490401113));
#9511=CARTESIAN_POINT('Ctrl Pts',(0.0338304498224533,-7.15013155025275,
-0.188400152822704));
#9512=CARTESIAN_POINT('Ctrl Pts',(-0.0478462800740612,-7.13907305551679,
-0.183166815244296));
#9513=CARTESIAN_POINT('Ctrl Pts',(-0.135467438763938,-7.17191935323474,
-0.177933477665887));
#9514=CARTESIAN_POINT('Ctrl Pts',(-0.189747630523594,-7.23394391472528,
-0.172700140087479));
#9515=CARTESIAN_POINT('Ctrl Pts',(-0.229305791562914,-7.27914599512138,
-0.168886203474719));
#9516=CARTESIAN_POINT('Ctrl Pts',(-0.251156029290448,-7.33984512028938,
-0.165072266861958));
#9517=CARTESIAN_POINT('Ctrl Pts',(-0.2516645197469,-7.40021351101923,-0.161258330249198));
#9518=CARTESIAN_POINT('Origin',(0.,-7.4,-0.45));
#9519=CARTESIAN_POINT('',(-0.25205356191611,-7.39987360404796,-0.0612583302491979));
#9520=CARTESIAN_POINT('',(-0.251593604700942,-7.39979879766985,-0.0887416697508022));
#9521=CARTESIAN_POINT('',(-0.25175,-7.4,-0.45));
#9522=CARTESIAN_POINT('',(0.191346599666505,-7.2364012796625,0.));
#9523=CARTESIAN_POINT('Ctrl Pts',(-0.25205356191611,-7.39987360404796,-0.0612583302491979));
#9524=CARTESIAN_POINT('Ctrl Pts',(-0.251574539177045,-7.47426199643967,
-0.056538899568024));
#9525=CARTESIAN_POINT('Ctrl Pts',(-0.216528582359325,-7.54902721912311,
-0.0518194688868501));
#9526=CARTESIAN_POINT('Ctrl Pts',(-0.158787390485525,-7.59585256738247,
-0.0471000382056762));
#9527=CARTESIAN_POINT('Ctrl Pts',(-0.094758661244801,-7.64777680808492,
-0.0418667006272677));
#9528=CARTESIAN_POINT('Ctrl Pts',(-0.00282294424260245,-7.66534503829956,
-0.0366333630488592));
#9529=CARTESIAN_POINT('Ctrl Pts',(0.0757847404228917,-7.64053050058079,
-0.0314000254704507));
#9530=CARTESIAN_POINT('Ctrl Pts',(0.154392425088386,-7.61571596286203,-0.0261666878920423));
#9531=CARTESIAN_POINT('Ctrl Pts',(0.219672077417175,-7.54851865720985,-0.0209333503136338));
#9532=CARTESIAN_POINT('Ctrl Pts',(0.242359266047042,-7.46941964788139,-0.0157000127352254));
#9533=CARTESIAN_POINT('Ctrl Pts',(0.265046454676908,-7.39032063855293,-0.0104666751568169));
#9534=CARTESIAN_POINT('Ctrl Pts',(0.245141179607852,-7.29931992554818,-0.00523333757840846));
#9535=CARTESIAN_POINT('Ctrl Pts',(0.191346599666505,-7.2364012796625,0.));
#9536=CARTESIAN_POINT('',(-0.191702382984482,-7.23617294784579,6.20293008155665E-17));
#9537=CARTESIAN_POINT('Origin',(0.,-7.4,0.));
#9538=CARTESIAN_POINT('Ctrl Pts',(-0.191704050234201,-7.23617187785139,
3.46944695195361E-17));
#9539=CARTESIAN_POINT('Ctrl Pts',(-0.14033257538867,-7.17646167822941,-0.00499978774624427));
#9540=CARTESIAN_POINT('Ctrl Pts',(-0.0585928813496691,-7.14242247150708,
-0.00999957549248857));
#9541=CARTESIAN_POINT('Ctrl Pts',(0.0199179744619951,-7.14865372872736,
-0.0149993632387329));
#9542=CARTESIAN_POINT('Ctrl Pts',(0.102096225396913,-7.15517606011955,-0.0202327008171413));
#9543=CARTESIAN_POINT('Ctrl Pts',(0.180736942103683,-7.2058189496042,-0.0254660383955497));
#9544=CARTESIAN_POINT('Ctrl Pts',(0.220629131202208,-7.27793230733172,-0.0306993759739582));
#9545=CARTESIAN_POINT('Ctrl Pts',(0.260521320300732,-7.35004566505924,-0.0359327135523667));
#9546=CARTESIAN_POINT('Ctrl Pts',(0.261664981791011,-7.44362949102963,-0.0411660511307752));
#9547=CARTESIAN_POINT('Ctrl Pts',(0.223523601724647,-7.51669742191632,-0.0463993887091836));
#9548=CARTESIAN_POINT('Ctrl Pts',(0.185382221658284,-7.58976535280302,-0.0516327262875921));
#9549=CARTESIAN_POINT('Ctrl Pts',(0.107955800035278,-7.64231738860601,-0.0568660638660005));
#9550=CARTESIAN_POINT('Ctrl Pts',(0.0259706150012631,-7.6508052506037,-0.0620994014444089));
#9551=CARTESIAN_POINT('Ctrl Pts',(-0.0560145700327524,-7.65929311260139,
-0.0673327390228174));
#9552=CARTESIAN_POINT('Ctrl Pts',(-0.142558518477778,-7.62371680079378,
-0.0725660766012259));
#9553=CARTESIAN_POINT('Ctrl Pts',(-0.194864670716722,-7.56002034494844,
-0.0777994141796343));
#9554=CARTESIAN_POINT('Ctrl Pts',(-0.231319882275806,-7.51562656574637,
-0.081446832703357));
#9555=CARTESIAN_POINT('Ctrl Pts',(-0.25114405026367,-7.45757339860048,-0.0850942512270796));
#9556=CARTESIAN_POINT('Ctrl Pts',(-0.251593604700942,-7.39979879766985,
-0.0887416697508022));
#9557=CARTESIAN_POINT('Origin',(0.,7.4,-0.45));
#9558=CARTESIAN_POINT('',(-0.251358460963395,7.39999011478219,-0.761258330249198));
#9559=CARTESIAN_POINT('',(-0.2515844849848,7.39966621586329,-0.788741669750802));
#9560=CARTESIAN_POINT('',(-0.25175,7.4,-0.45));
#9561=CARTESIAN_POINT('',(-0.191346599666504,7.5635987203375,-0.8));
#9562=CARTESIAN_POINT('Ctrl Pts',(-0.2515844849848,7.39966621586329,-0.788741669750802));
#9563=CARTESIAN_POINT('Ctrl Pts',(-0.251071187758555,7.45892160063636,-0.792494446500535));
#9564=CARTESIAN_POINT('Ctrl Pts',(-0.229922182808404,7.51848035603044,-0.796247223250268));
#9565=CARTESIAN_POINT('Ctrl Pts',(-0.191346599666504,7.5635987203375,-0.8));
#9566=CARTESIAN_POINT('',(0.191702360493801,7.56382706695207,-0.8));
#9567=CARTESIAN_POINT('Origin',(0.,7.4,-0.8));
#9568=CARTESIAN_POINT('Ctrl Pts',(0.191704026215797,7.56382813610288,-0.8));
#9569=CARTESIAN_POINT('Ctrl Pts',(0.140332545101572,7.62353836531877,-0.795000212253756));
#9570=CARTESIAN_POINT('Ctrl Pts',(0.058592868207462,7.65757749184722,-0.790000424507511));
#9571=CARTESIAN_POINT('Ctrl Pts',(-0.0199179742868679,7.65134621809807,
-0.785000636761267));
#9572=CARTESIAN_POINT('Ctrl Pts',(-0.102096211282372,7.64482386940491,-0.779767299182859));
#9573=CARTESIAN_POINT('Ctrl Pts',(-0.18073691824322,7.59418103237105,-0.774533961604451));
#9574=CARTESIAN_POINT('Ctrl Pts',(-0.220629103980957,7.52206769300185,-0.769300624026042));
#9575=CARTESIAN_POINT('Ctrl Pts',(-0.241063780214276,7.48512780828857,-0.766619859433761));
#9576=CARTESIAN_POINT('Ctrl Pts',(-0.251330937500274,7.44255411530564,-0.763939094841479));
#9577=CARTESIAN_POINT('Ctrl Pts',(-0.251358460963395,7.39999011478219,-0.761258330249198));
#9578=CARTESIAN_POINT('Origin',(0.,7.4,-0.45));
#9579=CARTESIAN_POINT('',(-0.252017148126658,7.3998459827829,-0.661258330249197));
#9580=CARTESIAN_POINT('',(-0.252073462769148,7.40012038728064,-0.688741669750802));
#9581=CARTESIAN_POINT('',(-0.25175,7.4,-0.45));
#9582=CARTESIAN_POINT('Ctrl Pts',(-0.252073462769148,7.40012038728064,-0.688741669750802));
#9583=CARTESIAN_POINT('Ctrl Pts',(-0.252115690748467,7.40725647012215,-0.689194416785009));
#9584=CARTESIAN_POINT('Ctrl Pts',(-0.251838306299564,7.41438920118803,-0.689647163819216));
#9585=CARTESIAN_POINT('Ctrl Pts',(-0.251230534080426,7.42149364028408,-0.690099910853423));
#9586=CARTESIAN_POINT('Ctrl Pts',(-0.244205248538583,7.50361439489039,-0.695333248431831));
#9587=CARTESIAN_POINT('Ctrl Pts',(-0.193036110221656,7.58195499579916,-0.700566586010239));
#9588=CARTESIAN_POINT('Ctrl Pts',(-0.120664077269321,7.62139994469436,-0.705799923588648));
#9589=CARTESIAN_POINT('Ctrl Pts',(-0.0482920443169851,7.66084489358957,
-0.711033261167056));
#9590=CARTESIAN_POINT('Ctrl Pts',(0.0452828832707578,7.6613941904712,-0.716266598745465));
#9591=CARTESIAN_POINT('Ctrl Pts',(0.118103980273902,7.62278362739801,-0.721499936323873));
#9592=CARTESIAN_POINT('Ctrl Pts',(0.190925077277045,7.58417306432483,-0.726733273902282));
#9593=CARTESIAN_POINT('Ctrl Pts',(0.242992343695589,7.50640264129683,-0.73196661148069));
#9594=CARTESIAN_POINT('Ctrl Pts',(0.250965115890772,7.42437728229464,-0.737199949059099));
#9595=CARTESIAN_POINT('Ctrl Pts',(0.258937888085954,7.34235192329245,-0.742433286637507));
#9596=CARTESIAN_POINT('Ctrl Pts',(0.222816166057774,7.25607162831608,-0.747666624215915));
#9597=CARTESIAN_POINT('Ctrl Pts',(0.158787417691483,7.20414739331457,-0.752899961794324));
#9598=CARTESIAN_POINT('Ctrl Pts',(0.0947586693251928,7.15222315831307,-0.758133299372733));
#9599=CARTESIAN_POINT('Ctrl Pts',(0.00282289462079141,7.13465498328644,
-0.763366636951141));
#9600=CARTESIAN_POINT('Ctrl Pts',(-0.0757847619957929,7.15946949434078,
-0.76859997452955));
#9601=CARTESIAN_POINT('Ctrl Pts',(-0.154392418612378,7.18428400539513,-0.773833312107958));
#9602=CARTESIAN_POINT('Ctrl Pts',(-0.219671957141145,7.25148120253045,-0.779066649686367));
#9603=CARTESIAN_POINT('Ctrl Pts',(-0.242359147390014,7.33058021979462,-0.784299987264775));
#9604=CARTESIAN_POINT('Ctrl Pts',(-0.24877756865406,7.3529580818747,-0.785780548093451));
#9605=CARTESIAN_POINT('Ctrl Pts',(-0.251786993105406,7.37628853916314,-0.787261108922127));
#9606=CARTESIAN_POINT('Ctrl Pts',(-0.2515844849848,7.39966621586329,-0.788741669750802));
#9607=CARTESIAN_POINT('Ctrl Pts',(-0.251358460963395,7.39999011478219,-0.761258330249198));
#9608=CARTESIAN_POINT('Ctrl Pts',(-0.25138466828076,7.35946148417043,-0.758705757263071));
#9609=CARTESIAN_POINT('Ctrl Pts',(-0.242127126249713,7.31894164121318,-0.756153184276943));
#9610=CARTESIAN_POINT('Ctrl Pts',(-0.223523578567029,7.28330258339987,-0.753600611290816));
#9611=CARTESIAN_POINT('Ctrl Pts',(-0.185382202900737,7.21023465487163,-0.748367273712408));
#9612=CARTESIAN_POINT('Ctrl Pts',(-0.107955787053529,7.15768263951967,-0.743133936134));
#9613=CARTESIAN_POINT('Ctrl Pts',(-0.025970610812802,7.14919478175684,-0.737900598555592));
#9614=CARTESIAN_POINT('Ctrl Pts',(0.0560145654279252,7.14070692399402,-0.732667260977183));
#9615=CARTESIAN_POINT('Ctrl Pts',(0.14255850206217,7.17628322382034,-0.727433923398774));
#9616=CARTESIAN_POINT('Ctrl Pts',(0.194864648070335,7.2399796707009,-0.722200585820366));
#9617=CARTESIAN_POINT('Ctrl Pts',(0.247170794078499,7.30367611758145,-0.716967248241957));
#9618=CARTESIAN_POINT('Ctrl Pts',(0.265239149460586,7.39549271151625,-0.711733910663549));
#9619=CARTESIAN_POINT('Ctrl Pts',(0.240965785765977,7.47425967354379,-0.706500573085141));
#9620=CARTESIAN_POINT('Ctrl Pts',(0.216692422071369,7.55302663557132,-0.701267235506732));
#9621=CARTESIAN_POINT('Ctrl Pts',(0.150077339300067,7.61874396569159,-0.696033897928324));
#9622=CARTESIAN_POINT('Ctrl Pts',(0.0709891645753919,7.64194865395628,-0.690800560349915));
#9623=CARTESIAN_POINT('Ctrl Pts',(-0.00809901014928227,7.66515334222097,
-0.685567222771507));
#9624=CARTESIAN_POINT('Ctrl Pts',(-0.0996602768273276,7.64584538863009,
-0.680333885193098));
#9625=CARTESIAN_POINT('Ctrl Pts',(-0.162643413958381,7.59268077865113,-0.67510054761469));
#9626=CARTESIAN_POINT('Ctrl Pts',(-0.21817370487162,7.54580718052792,-0.670486475159526));
#9627=CARTESIAN_POINT('Ctrl Pts',(-0.251489057009901,7.47261543070241,-0.665872402704361));
#9628=CARTESIAN_POINT('Ctrl Pts',(-0.252017148126658,7.3998459827829,-0.661258330249197));
#9629=CARTESIAN_POINT('Origin',(0.,7.4,-0.45));
#9630=CARTESIAN_POINT('',(-0.251711667638598,7.40021666645972,-0.561258330249198));
#9631=CARTESIAN_POINT('',(-0.251375292868799,7.40005668164188,-0.588741669750802));
#9632=CARTESIAN_POINT('',(-0.25175,7.4,-0.45));
#9633=CARTESIAN_POINT('Ctrl Pts',(-0.251375292868799,7.40005668164188,-0.588741669750802));
#9634=CARTESIAN_POINT('Ctrl Pts',(-0.251453247461991,7.4379339415428,-0.591127724647892));
#9635=CARTESIAN_POINT('Ctrl Pts',(-0.243409898811809,7.47577976703267,-0.593513779544981));
#9636=CARTESIAN_POINT('Ctrl Pts',(-0.227072449902118,7.50962152054577,-0.595899834442071));
#9637=CARTESIAN_POINT('Ctrl Pts',(-0.191239500115965,7.58384668636041,-0.601133172020479));
#9638=CARTESIAN_POINT('Ctrl Pts',(-0.115507191401049,7.63880997927991,-0.606366509598887));
#9639=CARTESIAN_POINT('Ctrl Pts',(-0.0338304532489083,7.64986847505112,
-0.611599847177296));
#9640=CARTESIAN_POINT('Ctrl Pts',(0.0478462849032329,7.66092697082232,-0.616833184755704));
#9641=CARTESIAN_POINT('Ctrl Pts',(0.135467452492599,7.62808066944522,-0.622066522334113));
#9642=CARTESIAN_POINT('Ctrl Pts',(0.189747649694627,7.56605610184571,-0.627299859912522));
#9643=CARTESIAN_POINT('Ctrl Pts',(0.244027846896655,7.5040315342462,-0.63253319749093));
#9644=CARTESIAN_POINT('Ctrl Pts',(0.264967073711345,7.41282870042428,-0.637766535069338));
#9645=CARTESIAN_POINT('Ctrl Pts',(0.243177185935535,7.33333936475981,-0.642999872647746));
#9646=CARTESIAN_POINT('Ctrl Pts',(0.221387298159724,7.25385002909535,-0.648233210226155));
#9647=CARTESIAN_POINT('Ctrl Pts',(0.156868295793411,7.18607419158834,-0.653466547804564));
#9648=CARTESIAN_POINT('Ctrl Pts',(0.0785474648464412,7.16039839199962,-0.658699885382972));
#9649=CARTESIAN_POINT('Ctrl Pts',(0.000226633899471557,7.1347225924109,
-0.663933222961381));
#9650=CARTESIAN_POINT('Ctrl Pts',(-0.0918960256281538,7.15114683074047,
-0.669166560539789));
#9651=CARTESIAN_POINT('Ctrl Pts',(-0.156516639008589,7.20230940405719,-0.674399898118197));
#9652=CARTESIAN_POINT('Ctrl Pts',(-0.215546787295137,7.24904579561427,-0.679180488662399));
#9653=CARTESIAN_POINT('Ctrl Pts',(-0.251627574307423,7.32476994304303,-0.6839610792066));
#9654=CARTESIAN_POINT('Ctrl Pts',(-0.252073462769148,7.40012038728064,-0.688741669750802));
#9655=CARTESIAN_POINT('Ctrl Pts',(-0.252017148126658,7.3998459827829,-0.661258330249197));
#9656=CARTESIAN_POINT('Ctrl Pts',(-0.252088024432499,7.39007943022609,-0.660639065125953));
#9657=CARTESIAN_POINT('Ctrl Pts',(-0.251568306017017,7.38032048456503,-0.660019800002709));
#9658=CARTESIAN_POINT('Ctrl Pts',(-0.250432433693752,7.37063379235739,-0.659400534879464));
#9659=CARTESIAN_POINT('Ctrl Pts',(-0.240833308714009,7.28877268240962,-0.654167197301056));
#9660=CARTESIAN_POINT('Ctrl Pts',(-0.187230051170462,7.21207172888109,-0.648933859722647));
#9661=CARTESIAN_POINT('Ctrl Pts',(-0.113656113647963,7.17491996861538,-0.643700522144239));
#9662=CARTESIAN_POINT('Ctrl Pts',(-0.0400821761254621,7.13776820834967,
-0.638467184565831));
#9663=CARTESIAN_POINT('Ctrl Pts',(0.0534624413759923,7.14016564134677,-0.633233846987422));
#9664=CARTESIAN_POINT('Ctrl Pts',(0.125036647626303,7.18103746796602,-0.628000509409014));
#9665=CARTESIAN_POINT('Ctrl Pts',(0.196610853876614,7.22190929458527,-0.622767171830605));
#9666=CARTESIAN_POINT('Ctrl Pts',(0.246214648875781,7.30125551482666,-0.617533834252197));
#9667=CARTESIAN_POINT('Ctrl Pts',(0.251607890189855,7.38350082018848,-0.612300496673788));
#9668=CARTESIAN_POINT('Ctrl Pts',(0.257001131503928,7.46574612555029,-0.60706715909538));
#9669=CARTESIAN_POINT('Ctrl Pts',(0.218183819132908,7.55089051603252,-0.601833821516972));
#9670=CARTESIAN_POINT('Ctrl Pts',(0.152559902600542,7.6007591205591,-0.596600483938563));
#9671=CARTESIAN_POINT('Ctrl Pts',(0.0869359860681766,7.65062772508569,-0.591367146360155));
#9672=CARTESIAN_POINT('Ctrl Pts',(-0.00549453462553363,7.66522054365662,
-0.586133808781746));
#9673=CARTESIAN_POINT('Ctrl Pts',(-0.0832900027313079,7.63799480376286,
-0.580900471203338));
#9674=CARTESIAN_POINT('Ctrl Pts',(-0.161085470837084,7.61076906386911,-0.575667133624929));
#9675=CARTESIAN_POINT('Ctrl Pts',(-0.224245886354923,7.54172476551065,-0.570433796046521));
#9676=CARTESIAN_POINT('Ctrl Pts',(-0.244452968778356,7.46181825714769,-0.565200458468112));
#9677=CARTESIAN_POINT('Ctrl Pts',(-0.249526780576268,7.44175447077981,-0.563886415728474));
#9678=CARTESIAN_POINT('Ctrl Pts',(-0.251892531940355,7.42100585930017,-0.562572372988836));
#9679=CARTESIAN_POINT('Ctrl Pts',(-0.251711667638598,7.40021666645972,-0.561258330249198));
#9680=CARTESIAN_POINT('Origin',(0.,7.4,-0.45));
#9681=CARTESIAN_POINT('',(-0.251454189985941,7.399856210792,-0.461258330249197));
#9682=CARTESIAN_POINT('',(-0.251895025789683,7.3998017247554,-0.488741669750802));
#9683=CARTESIAN_POINT('',(-0.25175,7.4,-0.45));
#9684=CARTESIAN_POINT('Ctrl Pts',(-0.251895025789683,7.3998017247554,-0.488741669750802));
#9685=CARTESIAN_POINT('Ctrl Pts',(-0.251306443088966,7.46800945010948,-0.493061032510774));
#9686=CARTESIAN_POINT('Ctrl Pts',(-0.222557870777557,7.53665464789974,-0.497380395270746));
#9687=CARTESIAN_POINT('Ctrl Pts',(-0.17309083838734,7.583353031007,-0.501699758030719));
#9688=CARTESIAN_POINT('Ctrl Pts',(-0.113156608759973,7.63993276666405,-0.506933095609127));
#9689=CARTESIAN_POINT('Ctrl Pts',(-0.0228082340311984,7.66429516552368,
-0.512166433187536));
#9690=CARTESIAN_POINT('Ctrl Pts',(0.0574461588212237,7.64551723115025,-0.517399770765944));
#9691=CARTESIAN_POINT('Ctrl Pts',(0.137700551673646,7.62673929677682,-0.522633108344352));
#9692=CARTESIAN_POINT('Ctrl Pts',(0.207860962649715,7.56482102917033,-0.527866445922761));
#9693=CARTESIAN_POINT('Ctrl Pts',(0.236470634513469,7.48752377667808,-0.533099783501169));
#9694=CARTESIAN_POINT('Ctrl Pts',(0.265080306377223,7.41022652418583,-0.538333121079578));
#9695=CARTESIAN_POINT('Ctrl Pts',(0.252139239128661,7.31755028680782,-0.543566458657986));
#9696=CARTESIAN_POINT('Ctrl Pts',(0.203449623212889,7.25104690807429,-0.548799796236395));
#9697=CARTESIAN_POINT('Ctrl Pts',(0.154760007297116,7.18454352934075,-0.554033133814803));
#9698=CARTESIAN_POINT('Ctrl Pts',(0.0703218427141316,7.1442130092517,-0.559266471393212));
#9699=CARTESIAN_POINT('Ctrl Pts',(-0.0120066161663935,7.14813771389866,
-0.56449980897162));
#9700=CARTESIAN_POINT('Ctrl Pts',(-0.0943350750469181,7.15206241854562,
-0.569733146550028));
#9701=CARTESIAN_POINT('Ctrl Pts',(-0.174553828224984,7.20024234792858,-0.574966484128437));
#9702=CARTESIAN_POINT('Ctrl Pts',(-0.216696409385322,7.27107583197496,-0.580199821706845));
#9703=CARTESIAN_POINT('Ctrl Pts',(-0.239624768140347,7.30961394448175,-0.583047104388164));
#9704=CARTESIAN_POINT('Ctrl Pts',(-0.251282269542556,7.35485769386367,-0.585894387069483));
#9705=CARTESIAN_POINT('Ctrl Pts',(-0.251375292868799,7.40005668164188,-0.588741669750802));
#9706=CARTESIAN_POINT('Ctrl Pts',(-0.251711667638598,7.40021666645972,-0.561258330249198));
#9707=CARTESIAN_POINT('Ctrl Pts',(-0.251172217510369,7.33821033002641,-0.557339035410427));
#9708=CARTESIAN_POINT('Ctrl Pts',(-0.227977964094547,7.27584298004936,-0.553419740571657));
#9709=CARTESIAN_POINT('Ctrl Pts',(-0.18641260996181,7.23020868929834,-0.549500445732887));
#9710=CARTESIAN_POINT('Ctrl Pts',(-0.130911419392803,7.1692743481794,-0.544267108154479));
#9711=CARTESIAN_POINT('Ctrl Pts',(-0.0426552889257632,7.13817438430899,
-0.53903377057607));
#9712=CARTESIAN_POINT('Ctrl Pts',(0.0387857232876696,7.15085261716797,-0.533800432997662));
#9713=CARTESIAN_POINT('Ctrl Pts',(0.120226735501102,7.16353085002696,-0.528567095419254));
#9714=CARTESIAN_POINT('Ctrl Pts',(0.194852629460927,7.21998727961534,-0.523333757840845));
#9715=CARTESIAN_POINT('Ctrl Pts',(0.22920452700707,7.29490939417427,-0.518100420262437));
#9716=CARTESIAN_POINT('Ctrl Pts',(0.263556424553213,7.36983150873319,-0.512867082684028));
#9717=CARTESIAN_POINT('Ctrl Pts',(0.257634325685674,7.46321930826266,-0.50763374510562));
#9718=CARTESIAN_POINT('Ctrl Pts',(0.214093432155548,7.53320192525145,-0.502400407527211));
#9719=CARTESIAN_POINT('Ctrl Pts',(0.170552538625422,7.60318454224025,-0.497167069948803));
#9720=CARTESIAN_POINT('Ctrl Pts',(0.0893928504327086,7.64976197668837,-0.491933732370394));
#9721=CARTESIAN_POINT('Ctrl Pts',(0.00700270292694295,7.65205101225613,
-0.486700394791986));
#9722=CARTESIAN_POINT('Ctrl Pts',(-0.0753874445788215,7.6543400478239,-0.481467057213577));
#9723=CARTESIAN_POINT('Ctrl Pts',(-0.159008051397638,7.61234068451132,-0.476233719635169));
#9724=CARTESIAN_POINT('Ctrl Pts',(-0.206367417274562,7.54488353841248,-0.47100038205676));
#9725=CARTESIAN_POINT('Ctrl Pts',(-0.235754488720125,7.50302554611858,-0.467753031454239));
#9726=CARTESIAN_POINT('Ctrl Pts',(-0.251179692325698,7.45136540173257,-0.464505680851719));
#9727=CARTESIAN_POINT('Ctrl Pts',(-0.251454189985941,7.399856210792,-0.461258330249197));
#9728=CARTESIAN_POINT('Origin',(0.,7.4,-0.45));
#9729=CARTESIAN_POINT('',(-0.252147107674537,7.3999852313674,-0.361258330249197));
#9730=CARTESIAN_POINT('',(-0.251847334099258,7.40020792401048,-0.388741669750802));
#9731=CARTESIAN_POINT('',(-0.25175,7.4,-0.45));
#9732=CARTESIAN_POINT('Ctrl Pts',(-0.251847334099258,7.40020792401048,-0.388741669750802));
#9733=CARTESIAN_POINT('Ctrl Pts',(-0.251989609797241,7.41631226426441,-0.389761002795248));
#9734=CARTESIAN_POINT('Ctrl Pts',(-0.250573895373447,7.43239170472893,-0.390780335839695));
#9735=CARTESIAN_POINT('Ctrl Pts',(-0.24750824943319,7.44815016809482,-0.391799668884141));
#9736=CARTESIAN_POINT('Ctrl Pts',(-0.231768977378143,7.52905538249945,-0.39703300646255));
#9737=CARTESIAN_POINT('Ctrl Pts',(-0.172539524660956,7.60150003240856,-0.402266344040958));
#9738=CARTESIAN_POINT('Ctrl Pts',(-0.0963757005174525,7.63300321151708,
-0.407499681619367));
#9739=CARTESIAN_POINT('Ctrl Pts',(-0.0202118763739491,7.66450639062559,
-0.412733019197775));
#9740=CARTESIAN_POINT('Ctrl Pts',(0.0728863191958706,7.65506809893352,-0.417966356776183));
#9741=CARTESIAN_POINT('Ctrl Pts',(0.141177863638472,7.60892003982476,-0.423199694354592));
#9742=CARTESIAN_POINT('Ctrl Pts',(0.209469408081073,7.562771980716,-0.428433031933));
#9743=CARTESIAN_POINT('Ctrl Pts',(0.252954301396456,7.47991415419055,-0.433666369511409));
#9744=CARTESIAN_POINT('Ctrl Pts',(0.252135883073263,7.39749626416295,-0.438899707089817));
#9745=CARTESIAN_POINT('Ctrl Pts',(0.251317464750071,7.31507837413536,-0.444133044668226));
#9746=CARTESIAN_POINT('Ctrl Pts',(0.206195734788304,7.23310042060562,-0.449366382246634));
#9747=CARTESIAN_POINT('Ctrl Pts',(0.13700123726806,7.18831761238753,-0.454599719825042));
#9748=CARTESIAN_POINT('Ctrl Pts',(0.0678067397478142,7.14353480416943,-0.459833057403451));
#9749=CARTESIAN_POINT('Ctrl Pts',(-0.0254605253309101,7.13594714126297,
-0.465066394981859));
#9750=CARTESIAN_POINT('Ctrl Pts',(-0.100983732313105,7.1689565884905,-0.470299732560268));
#9751=CARTESIAN_POINT('Ctrl Pts',(-0.176506939295298,7.20196603571802,-0.475533070138676));
#9752=CARTESIAN_POINT('Ctrl Pts',(-0.234286088180962,7.27557259307953,-0.480766407717085));
#9753=CARTESIAN_POINT('Ctrl Pts',(-0.248415620360814,7.35677440798752,-0.485999745295493));
#9754=CARTESIAN_POINT('Ctrl Pts',(-0.250883268666544,7.37095587687334,-0.48691372011393));
#9755=CARTESIAN_POINT('Ctrl Pts',(-0.252019569570078,7.38536900704663,-0.487827694932366));
#9756=CARTESIAN_POINT('Ctrl Pts',(-0.251895025789683,7.3998017247554,-0.488741669750802));
#9757=CARTESIAN_POINT('Ctrl Pts',(-0.251454189985941,7.399856210792,-0.461258330249197));
#9758=CARTESIAN_POINT('Ctrl Pts',(-0.251622064923045,7.36835465926041,-0.45927234327331));
#9759=CARTESIAN_POINT('Ctrl Pts',(-0.246123277962045,7.33690956728528,-0.457286356297422));
#9760=CARTESIAN_POINT('Ctrl Pts',(-0.234685894568262,7.30779760576974,-0.455300369321535));
#9761=CARTESIAN_POINT('Ctrl Pts',(-0.204546881050007,7.23108374811093,-0.450067031743127));
#9762=CARTESIAN_POINT('Ctrl Pts',(-0.133170729078467,7.17057096167843,-0.444833694164718));
#9763=CARTESIAN_POINT('Ctrl Pts',(-0.0525592787470221,7.15339044455997,
-0.43960035658631));
#9764=CARTESIAN_POINT('Ctrl Pts',(0.0280521715844237,7.13620992744151,-0.434367019007901));
#9765=CARTESIAN_POINT('Ctrl Pts',(0.117898920275772,7.1623616796371,-0.429133681429493));
#9766=CARTESIAN_POINT('Ctrl Pts',(0.176697746566812,7.22012043759096,-0.423900343851084));
#9767=CARTESIAN_POINT('Ctrl Pts',(0.23549657285785,7.27787919554482,-0.418667006272676));
#9768=CARTESIAN_POINT('Ctrl Pts',(0.26324747674858,7.36724495925696,-0.413433668694268));
#9769=CARTESIAN_POINT('Ctrl Pts',(0.247508207368464,7.44815015991153,-0.408200331115859));
#9770=CARTESIAN_POINT('Ctrl Pts',(0.231768937988348,7.52905536056611,-0.402966993537451));
#9771=CARTESIAN_POINT('Ctrl Pts',(0.172539495337386,7.60149999816312,-0.397733655959042));
#9772=CARTESIAN_POINT('Ctrl Pts',(0.0963756841381397,7.63300317191756,-0.392500318380633));
#9773=CARTESIAN_POINT('Ctrl Pts',(0.0202118729388946,7.664506345672,-0.387266980802225));
#9774=CARTESIAN_POINT('Ctrl Pts',(-0.0728863068086339,7.65506805558386,
-0.382033643223817));
#9775=CARTESIAN_POINT('Ctrl Pts',(-0.141177839644895,7.60892000431816,-0.376800305645409));
#9776=CARTESIAN_POINT('Ctrl Pts',(-0.208781945514779,7.56323648230766,-0.371619647180005));
#9777=CARTESIAN_POINT('Ctrl Pts',(-0.252076301533613,7.48157852511813,-0.366438988714601));
#9778=CARTESIAN_POINT('Ctrl Pts',(-0.252147107674537,7.3999852313674,-0.361258330249197));
#9779=CARTESIAN_POINT('Origin',(0.,7.4,-0.45));
#9780=CARTESIAN_POINT('',(-0.251485840701091,7.40016248328612,-0.261258330249198));
#9781=CARTESIAN_POINT('',(-0.251389294427012,7.3999184928281,-0.288741669750802));
#9782=CARTESIAN_POINT('',(-0.25175,7.4,-0.45));
#9783=CARTESIAN_POINT('Ctrl Pts',(-0.251389294427012,7.3999184928281,-0.288741669750802));
#9784=CARTESIAN_POINT('Ctrl Pts',(-0.251250073158243,7.44678343134187,-0.291694310658131));
#9785=CARTESIAN_POINT('Ctrl Pts',(-0.238659177002226,7.49371785771873,-0.29464695156546));
#9786=CARTESIAN_POINT('Ctrl Pts',(-0.214093468541586,7.53320194788991,-0.297599592472789));
#9787=CARTESIAN_POINT('Ctrl Pts',(-0.170552567611783,7.60318457677283,-0.302832930051198));
#9788=CARTESIAN_POINT('Ctrl Pts',(-0.0893928656252568,7.64976201913611,
-0.308066267629606));
#9789=CARTESIAN_POINT('Ctrl Pts',(-0.00700270411693429,7.65205105509271,
-0.313299605208015));
#9790=CARTESIAN_POINT('Ctrl Pts',(0.075387457391387,7.65434009104931,-0.318532942786423));
#9791=CARTESIAN_POINT('Ctrl Pts',(0.159008078421505,7.61234072059923,-0.323766280364831));
#9792=CARTESIAN_POINT('Ctrl Pts',(0.206367452347224,7.54488356303595,-0.32899961794324));
#9793=CARTESIAN_POINT('Ctrl Pts',(0.253726826272944,7.47742640547267,-0.334232955521648));
#9794=CARTESIAN_POINT('Ctrl Pts',(0.264824953094265,7.3845114607962,-0.339466293100057));
#9795=CARTESIAN_POINT('Ctrl Pts',(0.234685934453829,7.30779759009962,-0.344699630678465));
#9796=CARTESIAN_POINT('Ctrl Pts',(0.204546915813393,7.23108371940303,-0.349932968256874));
#9797=CARTESIAN_POINT('Ctrl Pts',(0.133170751711201,7.17057092268632,-0.355166305835282));
#9798=CARTESIAN_POINT('Ctrl Pts',(0.0525592876795934,7.15339040264801,-0.360399643413691));
#9799=CARTESIAN_POINT('Ctrl Pts',(-0.0280521763520133,7.13620988260969,
-0.365632980992099));
#9800=CARTESIAN_POINT('Ctrl Pts',(-0.117898940313035,7.16236163924978,-0.370866318570508));
#9801=CARTESIAN_POINT('Ctrl Pts',(-0.176697776597091,7.2201204070199,-0.376099656148916));
#9802=CARTESIAN_POINT('Ctrl Pts',(-0.2240439603623,7.26662910354725,-0.380313660682878));
#9803=CARTESIAN_POINT('Ctrl Pts',(-0.251259154956394,7.3336312901848,-0.38452766521684));
#9804=CARTESIAN_POINT('Ctrl Pts',(-0.251847334099258,7.40020792401048,-0.388741669750802));
#9805=CARTESIAN_POINT('Ctrl Pts',(-0.252147107674537,7.3999852313674,-0.361258330249197));
#9806=CARTESIAN_POINT('Ctrl Pts',(-0.252147827661142,7.39915555645819,-0.361205651136192));
#9807=CARTESIAN_POINT('Ctrl Pts',(-0.252144078472191,7.39832588823498,-0.361152972023188));
#9808=CARTESIAN_POINT('Ctrl Pts',(-0.252135840222057,7.3974962645886,-0.361100292910183));
#9809=CARTESIAN_POINT('Ctrl Pts',(-0.251317422037965,7.31507838856804,-0.355866955331774));
#9810=CARTESIAN_POINT('Ctrl Pts',(-0.206195699744786,7.2331004489702,-0.350633617753366));
#9811=CARTESIAN_POINT('Ctrl Pts',(-0.137001213984329,7.1883176483633,-0.345400280174958));
#9812=CARTESIAN_POINT('Ctrl Pts',(-0.0678067282238716,7.14353484775639,
-0.340166942596549));
#9813=CARTESIAN_POINT('Ctrl Pts',(0.0254605210038648,7.13594718614041,-0.334933605018141));
#9814=CARTESIAN_POINT('Ctrl Pts',(0.100983715150651,7.16895662775745,-0.329700267439732));
#9815=CARTESIAN_POINT('Ctrl Pts',(0.176506909297436,7.20196606937449,-0.324466929861324));
#9816=CARTESIAN_POINT('Ctrl Pts',(0.234286048363272,7.27557261422455,-0.319233592282915));
#9817=CARTESIAN_POINT('Ctrl Pts',(0.248415578141833,7.35677441533289,-0.314000254704507));
#9818=CARTESIAN_POINT('Ctrl Pts',(0.262545107920394,7.43797621644123,-0.308766917126099));
#9819=CARTESIAN_POINT('Ctrl Pts',(0.233025028411682,7.52677327380785,-0.30353357954769));
#9820=CARTESIAN_POINT('Ctrl Pts',(0.173090808970175,7.58335299984742,-0.298300241969282));
#9821=CARTESIAN_POINT('Ctrl Pts',(0.113156589528667,7.63993272588698,-0.293066904390873));
#9822=CARTESIAN_POINT('Ctrl Pts',(0.022808230154364,7.6642951205995,-0.287833566812465));
#9823=CARTESIAN_POINT('Ctrl Pts',(-0.0574461490583136,7.64551718942048,
-0.282600229234056));
#9824=CARTESIAN_POINT('Ctrl Pts',(-0.137700528270991,7.62673925824146,-0.277366891655648));
#9825=CARTESIAN_POINT('Ctrl Pts',(-0.207860927322042,7.56482100117091,-0.272133554077239));
#9826=CARTESIAN_POINT('Ctrl Pts',(-0.236470594324117,7.48752376180974,-0.266900216498831));
#9827=CARTESIAN_POINT('Ctrl Pts',(-0.246751636103367,7.45974657211945,-0.265019587748953));
#9828=CARTESIAN_POINT('Ctrl Pts',(-0.251666966336733,7.4299833961716,-0.263138958999075));
#9829=CARTESIAN_POINT('Ctrl Pts',(-0.251485840701091,7.40016248328612,-0.261258330249198));
#9830=CARTESIAN_POINT('Origin',(0.,7.4,-0.45));
#9831=CARTESIAN_POINT('',(-0.251664502419995,7.39978648873079,-0.161258330249198));
#9832=CARTESIAN_POINT('',(-0.252102618136395,7.39990630057405,-0.188741669750802));
#9833=CARTESIAN_POINT('',(-0.25175,7.4,-0.45));
#9834=CARTESIAN_POINT('Ctrl Pts',(-0.252102618136395,7.39990630057405,-0.188741669750802));
#9835=CARTESIAN_POINT('Ctrl Pts',(-0.251729671980332,7.47689446754405,-0.193627618521014));
#9836=CARTESIAN_POINT('Ctrl Pts',(-0.213827741655731,7.55420081887498,-0.198513567291225));
#9837=CARTESIAN_POINT('Ctrl Pts',(-0.152559928540191,7.60075915469979,-0.203399516061437));
#9838=CARTESIAN_POINT('Ctrl Pts',(-0.0869360008643037,7.65062776772039,
-0.208632853639846));
#9839=CARTESIAN_POINT('Ctrl Pts',(0.00549453556043952,7.66522058873043,
-0.213866191218254));
#9840=CARTESIAN_POINT('Ctrl Pts',(0.0832900168929199,7.63799484419977,-0.219099528796662));
#9841=CARTESIAN_POINT('Ctrl Pts',(0.1610854982254,7.61076909966911,-0.224332866375071));
#9842=CARTESIAN_POINT('Ctrl Pts',(0.224245924465617,7.54172478959775,-0.229566203953479));
#9843=CARTESIAN_POINT('Ctrl Pts',(0.24445301032052,7.46181826765958,-0.234799541531888));
#9844=CARTESIAN_POINT('Ctrl Pts',(0.264660096175424,7.38191174572141,-0.240032879110296));
#9845=CARTESIAN_POINT('Ctrl Pts',(0.241913841645014,7.29114301191644,-0.245266216688705));
#9846=CARTESIAN_POINT('Ctrl Pts',(0.186412641644911,7.23020866043887,-0.250499554267113));
#9847=CARTESIAN_POINT('Ctrl Pts',(0.13091144164481,7.16927430896129,-0.255732891845522));
#9848=CARTESIAN_POINT('Ctrl Pts',(0.042655296175016,7.13817433981112,-0.26096622942393));
#9849=CARTESIAN_POINT('Ctrl Pts',(-0.0387857298803423,7.1508525748262,-0.266199567002338));
#9850=CARTESIAN_POINT('Ctrl Pts',(-0.120226755935702,7.16353080984128,-0.271432904580747));
#9851=CARTESIAN_POINT('Ctrl Pts',(-0.194852662576626,7.2199872490216,-0.276666242159155));
#9852=CARTESIAN_POINT('Ctrl Pts',(-0.229204565960548,7.29490937631304,-0.281899579737564));
#9853=CARTESIAN_POINT('Ctrl Pts',(-0.24417517898123,7.32756055612776,-0.284180276408643));
#9854=CARTESIAN_POINT('Ctrl Pts',(-0.251496832557856,7.36371879479052,-0.286460973079723));
#9855=CARTESIAN_POINT('Ctrl Pts',(-0.251389294427012,7.3999184928281,-0.288741669750802));
#9856=CARTESIAN_POINT('Ctrl Pts',(-0.251485840701091,7.40016248328612,-0.261258330249198));
#9857=CARTESIAN_POINT('Ctrl Pts',(-0.251162937247801,7.34699896660984,-0.257905621420667));
#9858=CARTESIAN_POINT('Ctrl Pts',(-0.234642316978043,7.293651948577,-0.254552912592136));
#9859=CARTESIAN_POINT('Ctrl Pts',(-0.203449588637141,7.2510469333767,-0.251200203763606));
#9860=CARTESIAN_POINT('Ctrl Pts',(-0.154759980994992,7.18454356595661,-0.245966866185197));
#9861=CARTESIAN_POINT('Ctrl Pts',(-0.0703218307575955,7.14421305276819,
-0.240733528606789));
#9862=CARTESIAN_POINT('Ctrl Pts',(0.0120066141281704,7.14813775672736,-0.23550019102838));
#9863=CARTESIAN_POINT('Ctrl Pts',(0.0943350590139364,7.15206246068653,-0.230266853449972));
#9864=CARTESIAN_POINT('Ctrl Pts',(0.174553798548072,7.2002423817933,-0.225033515871563));
#9865=CARTESIAN_POINT('Ctrl Pts',(0.216696372552131,7.27107585384036,-0.219800178293155));
#9866=CARTESIAN_POINT('Ctrl Pts',(0.258838946556191,7.34190932588742,-0.214566840714746));
#9867=CARTESIAN_POINT('Ctrl Pts',(0.262905355030174,7.43539634887478,-0.209333503136338));
#9868=CARTESIAN_POINT('Ctrl Pts',(0.227072411321265,7.50962150200167,-0.204100165557929));
#9869=CARTESIAN_POINT('Ctrl Pts',(0.191239467612356,7.58384665512856,-0.198866827979521));
#9870=CARTESIAN_POINT('Ctrl Pts',(0.115507171720556,7.63880993839499,-0.193633490401113));
#9871=CARTESIAN_POINT('Ctrl Pts',(0.0338304474764224,7.64986843242236,-0.188400152822704));
#9872=CARTESIAN_POINT('Ctrl Pts',(-0.0478462767677109,7.66092692644973,
-0.183166815244296));
#9873=CARTESIAN_POINT('Ctrl Pts',(-0.135467429364177,7.62808063123805,-0.177933477665887));
#9874=CARTESIAN_POINT('Ctrl Pts',(-0.189747617397774,7.56605607392972,-0.172700140087479));
#9875=CARTESIAN_POINT('Ctrl Pts',(-0.229305775721628,7.5208539965815,-0.168886203474718));
#9876=CARTESIAN_POINT('Ctrl Pts',(-0.251156011991034,7.4601548753515,-0.165072266861958));
#9877=CARTESIAN_POINT('Ctrl Pts',(-0.251664502419995,7.39978648873079,-0.161258330249198));
#9878=CARTESIAN_POINT('Origin',(0.,7.4,-0.45));
#9879=CARTESIAN_POINT('',(-0.252053546614158,7.40012638988493,-0.0612583302491975));
#9880=CARTESIAN_POINT('',(-0.25159361924534,7.40020120251426,-0.088741669750802));
#9881=CARTESIAN_POINT('',(-0.25175,7.4,-0.45));
#9882=CARTESIAN_POINT('',(0.191346599666508,7.56359872033749,0.));
#9883=CARTESIAN_POINT('Ctrl Pts',(-0.252053546614158,7.40012638988493,-0.0612583302491975));
#9884=CARTESIAN_POINT('Ctrl Pts',(-0.251574518405349,7.32573800995496,-0.0565388995680237));
#9885=CARTESIAN_POINT('Ctrl Pts',(-0.216528551878887,7.25097281135749,-0.0518194688868499));
#9886=CARTESIAN_POINT('Ctrl Pts',(-0.158787371836513,7.20414745955911,-0.047100038205676));
#9887=CARTESIAN_POINT('Ctrl Pts',(-0.0947586557155584,7.15222321493229,
-0.0418667006272676));
#9888=CARTESIAN_POINT('Ctrl Pts',(-0.00282297831979787,7.13465494682447,
-0.0366333630488591));
#9889=CARTESIAN_POINT('Ctrl Pts',(0.0757847255684538,7.15946950281323,-0.0314000254704506));
#9890=CARTESIAN_POINT('Ctrl Pts',(0.154392429456705,7.18428405880198,-0.0261666878920422));
#9891=CARTESIAN_POINT('Ctrl Pts',(0.219672159837449,7.25148143888729,-0.0209333503136337));
#9892=CARTESIAN_POINT('Ctrl Pts',(0.242359347375236,7.33058044279975,-0.0157000127352253));
#9893=CARTESIAN_POINT('Ctrl Pts',(0.265046534913023,7.40967944671221,-0.0104666751568168));
#9894=CARTESIAN_POINT('Ctrl Pts',(0.245141179607854,7.50068007445182,-0.00523333757840841));
#9895=CARTESIAN_POINT('Ctrl Pts',(0.191346599666508,7.56359872033749,2.72395540626932E-17));
#9896=CARTESIAN_POINT('',(-0.191702394569677,7.56382704462399,5.75771190526024E-16));
#9897=CARTESIAN_POINT('Origin',(0.,7.4,0.));
#9898=CARTESIAN_POINT('Ctrl Pts',(-0.191704062602126,7.56382811505056,3.81639164714898E-16));
#9899=CARTESIAN_POINT('Ctrl Pts',(-0.140332590985575,7.6235382994157,-0.00499978774624405));
#9900=CARTESIAN_POINT('Ctrl Pts',(-0.0585928881206123,7.65757754738541,
-0.00999957549248847));
#9901=CARTESIAN_POINT('Ctrl Pts',(0.0199179745523958,7.65134629866448,-0.0149993632387329));
#9902=CARTESIAN_POINT('Ctrl Pts',(0.102096232669162,7.64482397616866,-0.0202327008171413));
#9903=CARTESIAN_POINT('Ctrl Pts',(0.180736954405333,7.59418105970145,-0.0254660383955498));
#9904=CARTESIAN_POINT('Ctrl Pts',(0.220629145239623,7.52206769251925,-0.0306993759739582));
#9905=CARTESIAN_POINT('Ctrl Pts',(0.260521336073913,7.44995432533705,-0.0359327135523667));
#9906=CARTESIAN_POINT('Ctrl Pts',(0.261664996006322,7.35637050743987,-0.0411660511307752));
#9907=CARTESIAN_POINT('Ctrl Pts',(0.22352361367014,7.28330257532835,-0.0463993887091836));
#9908=CARTESIAN_POINT('Ctrl Pts',(0.185382231333959,7.21023464321682,-0.0516327262875921));
#9909=CARTESIAN_POINT('Ctrl Pts',(0.107955806729186,7.15768259689094,-0.0568660638660005));
#9910=CARTESIAN_POINT('Ctrl Pts',(0.0259706171598658,7.14919473271428,-0.0620994014444089));
#9911=CARTESIAN_POINT('Ctrl Pts',(-0.0560145724094547,7.14070686853762,
-0.0673327390228173));
#9912=CARTESIAN_POINT('Ctrl Pts',(-0.142558526943323,7.17628318651017,-0.0725660766012259));
#9913=CARTESIAN_POINT('Ctrl Pts',(-0.19486468239543,7.239979646976,-0.0777994141796343));
#9914=CARTESIAN_POINT('Ctrl Pts',(-0.231319896193954,7.28437342939836,-0.0814468327033569));
#9915=CARTESIAN_POINT('Ctrl Pts',(-0.251144065024393,7.34242659901433,-0.0850942512270795));
#9916=CARTESIAN_POINT('Ctrl Pts',(-0.25159361924534,7.40020120251426,-0.088741669750802));
#9917=CARTESIAN_POINT('Origin',(7.4,0.,-0.45));
#9918=CARTESIAN_POINT('',(7.14864152176833,-9.8905947593236E-6,-0.761258330249198));
#9919=CARTESIAN_POINT('',(7.1484153974468,-0.000333656346126327,-0.788741669750802));
#9920=CARTESIAN_POINT('',(7.14825,3.08304831685346E-17,-0.45));
#9921=CARTESIAN_POINT('',(7.20865340033349,0.163598720337494,-0.8));
#9922=CARTESIAN_POINT('Ctrl Pts',(7.1484153974468,-0.000333656346126327,
-0.788741669750802));
#9923=CARTESIAN_POINT('Ctrl Pts',(7.14892873762876,0.0589216799335651,-0.792494446500535));
#9924=CARTESIAN_POINT('Ctrl Pts',(7.1700778171916,0.118480356030442,-0.796247223250267));
#9925=CARTESIAN_POINT('Ctrl Pts',(7.2086534003335,0.163598720337496,-0.8));
#9926=CARTESIAN_POINT('',(7.59170237435269,0.16382705780558,-0.8));
#9927=CARTESIAN_POINT('Origin',(7.4,0.,-0.8));
#9928=CARTESIAN_POINT('Ctrl Pts',(7.59170404101736,0.163828127476929,-0.8));
#9929=CARTESIAN_POINT('Ctrl Pts',(7.54033256376596,0.223538338460724,-0.795000212253756));
#9930=CARTESIAN_POINT('Ctrl Pts',(7.45859287630538,0.257577514423726,-0.790000424507512));
#9931=CARTESIAN_POINT('Ctrl Pts',(7.38008202560527,0.251346250864262,-0.785000636761268));
#9932=CARTESIAN_POINT('Ctrl Pts',(7.29790378002067,0.244823912836771,-0.779767299182859));
#9933=CARTESIAN_POINT('Ctrl Pts',(7.21926306705711,0.19418104347167,-0.77453396160445));
#9934=CARTESIAN_POINT('Ctrl Pts',(7.17937087924982,0.122067692789386,-0.769300624026042));
#9935=CARTESIAN_POINT('Ctrl Pts',(7.15893620195638,0.0851278022809988,-0.766619859433761));
#9936=CARTESIAN_POINT('Ctrl Pts',(7.14866904464232,0.0425541090180851,-0.763939094841479));
#9937=CARTESIAN_POINT('Ctrl Pts',(7.14864152176833,-9.8905947593236E-6,
-0.761258330249198));
#9938=CARTESIAN_POINT('Origin',(7.4,0.,-0.45));
#9939=CARTESIAN_POINT('',(7.14798283450166,-0.000154017160047509,-0.661258330249198));
#9940=CARTESIAN_POINT('',(7.14792656787638,0.000120390219947525,-0.688741669750802));
#9941=CARTESIAN_POINT('',(7.14825,3.08304831685346E-17,-0.45));
#9942=CARTESIAN_POINT('Ctrl Pts',(7.14792656787638,0.000120390219947525,
-0.688741669750802));
#9943=CARTESIAN_POINT('Ctrl Pts',(7.14788433994059,0.00725647209880052,
-0.689194416785009));
#9944=CARTESIAN_POINT('Ctrl Pts',(7.14816172440802,0.014389202158696,-0.689647163819216));
#9945=CARTESIAN_POINT('Ctrl Pts',(7.14876949662151,0.0214936402017243,-0.690099910853423));
#9946=CARTESIAN_POINT('Ctrl Pts',(7.15579478209814,0.103614382636149,-0.695333248431831));
#9947=CARTESIAN_POINT('Ctrl Pts',(7.20696391712096,0.18195496508943,-0.70056658601024));
#9948=CARTESIAN_POINT('Ctrl Pts',(7.27933593931993,0.221399912316197,-0.705799923588648));
#9949=CARTESIAN_POINT('Ctrl Pts',(7.3517079615189,0.260844859542965,-0.711033261167056));
#9950=CARTESIAN_POINT('Ctrl Pts',(7.44528287089401,0.261394171543217,-0.716266598745465));
#9951=CARTESIAN_POINT('Ctrl Pts',(7.51810396235645,0.222783607866771,-0.721499936323873));
#9952=CARTESIAN_POINT('Ctrl Pts',(7.5909250538189,0.184173044190324,-0.726733273902282));
#9953=CARTESIAN_POINT('Ctrl Pts',(7.64299232736868,0.10640260483718,-0.73196661148069));
#9954=CARTESIAN_POINT('Ctrl Pts',(7.65096509106803,0.0243772648179821,-0.737199949059099));
#9955=CARTESIAN_POINT('Ctrl Pts',(7.65893785476737,-0.0576480752012157,
-0.742433286637507));
#9956=CARTESIAN_POINT('Ctrl Pts',(7.62281610861627,-0.143928315886467,-0.747666624215916));
#9957=CARTESIAN_POINT('Ctrl Pts',(7.55878738396318,-0.195852557959908,-0.752899961794324));
#9958=CARTESIAN_POINT('Ctrl Pts',(7.4947586593101,-0.247776800033349,-0.758133299372733));
#9959=CARTESIAN_POINT('Ctrl Pts',(7.40282295615504,-0.26534504349498,-0.763366636951141));
#9960=CARTESIAN_POINT('Ctrl Pts',(7.32421526476616,-0.240530499385705,-0.768599974529549));
#9961=CARTESIAN_POINT('Ctrl Pts',(7.24560757337728,-0.215715955276429,-0.773833312107958));
#9962=CARTESIAN_POINT('Ctrl Pts',(7.18032789375458,-0.148518623596246,-0.779066649686366));
#9963=CARTESIAN_POINT('Ctrl Pts',(7.1576407055083,-0.0694196161641834,-0.784299987264775));
#9964=CARTESIAN_POINT('Ctrl Pts',(7.1512222848108,-0.0470417568657088,-0.785780548093451));
#9965=CARTESIAN_POINT('Ctrl Pts',(7.14821287237913,-0.0237113139144776,
-0.787261108922126));
#9966=CARTESIAN_POINT('Ctrl Pts',(7.1484153974468,-0.000333656346126327,
-0.788741669750802));
#9967=CARTESIAN_POINT('Ctrl Pts',(7.14864152176833,-9.8905947593236E-6,
-0.761258330249198));
#9968=CARTESIAN_POINT('Ctrl Pts',(7.14861531501193,-0.0405385203394587,
-0.758705757263071));
#9969=CARTESIAN_POINT('Ctrl Pts',(7.15787285816352,-0.0810583613501985,
-0.756153184276944));
#9970=CARTESIAN_POINT('Ctrl Pts',(7.17647640716818,-0.116697419870879,-0.753600611290817));
#9971=CARTESIAN_POINT('Ctrl Pts',(7.21461778554483,-0.189765349849391,-0.748367273712409));
#9972=CARTESIAN_POINT('Ctrl Pts',(7.29204420494912,-0.242317377806947,-0.743133936134));
#9973=CARTESIAN_POINT('Ctrl Pts',(7.37402938660657,-0.250805238180063,-0.737900598555592));
#9974=CARTESIAN_POINT('Ctrl Pts',(7.45601456826403,-0.25929309855318,-0.732667260977183));
#9975=CARTESIAN_POINT('Ctrl Pts',(7.54255851217464,-0.223716791341859,-0.727433923398775));
#9976=CARTESIAN_POINT('Ctrl Pts',(7.59486466202115,-0.160020338937948,-0.722200585820367));
#9977=CARTESIAN_POINT('Ctrl Pts',(7.64717081186766,-0.096323886534038,-0.716967248241958));
#9978=CARTESIAN_POINT('Ctrl Pts',(7.66523916765007,-0.00450728893753763,
-0.71173391066355));
#9979=CARTESIAN_POINT('Ctrl Pts',(7.6409658021157,0.0742596779135476,-0.706500573085141));
#9980=CARTESIAN_POINT('Ctrl Pts',(7.61669243658134,0.153026644764634,-0.701267235506733));
#9981=CARTESIAN_POINT('Ctrl Pts',(7.55007734973019,0.218743980870306,-0.696033897928324));
#9982=CARTESIAN_POINT('Ctrl Pts',(7.47098916964924,0.241948671073236,-0.690800560349916));
#9983=CARTESIAN_POINT('Ctrl Pts',(7.39190098956829,0.265153361276165,-0.685567222771507));
#9984=CARTESIAN_POINT('Ctrl Pts',(7.30033971625753,0.245845405576353,-0.680333885193099));
#9985=CARTESIAN_POINT('Ctrl Pts',(7.23735657471084,0.192680791744281,-0.675100547614691));
#9986=CARTESIAN_POINT('Ctrl Pts',(7.18182627990447,0.145807190223893,-0.670486475159527));
#9987=CARTESIAN_POINT('Ctrl Pts',(7.14851092559648,0.0726154356453729,-0.665872402704362));
#9988=CARTESIAN_POINT('Ctrl Pts',(7.14798283450166,-0.000154017160047509,
-0.661258330249198));
#9989=CARTESIAN_POINT('Origin',(7.4,0.,-0.45));
#9990=CARTESIAN_POINT('',(7.14828831497717,0.000216666477491244,-0.561258330249198));
#9991=CARTESIAN_POINT('',(7.14862473855677,5.66816876182724E-5,-0.588741669750802));
#9992=CARTESIAN_POINT('',(7.14825,3.08304831685346E-17,-0.45));
#9993=CARTESIAN_POINT('Ctrl Pts',(7.14862473855677,5.66816876182724E-5,
-0.588741669750802));
#9994=CARTESIAN_POINT('Ctrl Pts',(7.14854678397043,0.0379339368751698,-0.591127724647892));
#9995=CARTESIAN_POINT('Ctrl Pts',(7.1565901316137,0.0757797576445921,-0.593513779544981));
#9996=CARTESIAN_POINT('Ctrl Pts',(7.17292757848469,0.109621506901428,-0.595899834442071));
#9997=CARTESIAN_POINT('Ctrl Pts',(7.20876052379935,0.183846663380813,-0.601133172020479));
#9998=CARTESIAN_POINT('Ctrl Pts',(7.28449282307928,0.238809949198099,-0.606366509598887));
#9999=CARTESIAN_POINT('Ctrl Pts',(7.3661695509983,0.249868443686133,-0.611599847177296));
#10000=CARTESIAN_POINT('Ctrl Pts',(7.44784627891733,0.260926938174167,-0.616833184755704));
#10001=CARTESIAN_POINT('Ctrl Pts',(7.53546743547544,0.228080641332948,-0.622066522334113));
#10002=CARTESIAN_POINT('Ctrl Pts',(7.58974762593152,0.166056081305598,-0.627299859912522));
#10003=CARTESIAN_POINT('Ctrl Pts',(7.64402781638759,0.104031521278249,-0.63253319749093));
#10004=CARTESIAN_POINT('Ctrl Pts',(7.66496704074163,0.0128286980647704,
-0.637766535069338));
#10005=CARTESIAN_POINT('Ctrl Pts',(7.64317715560285,-0.0666606273237503,
-0.642999872647746));
#10006=CARTESIAN_POINT('Ctrl Pts',(7.62138727046407,-0.146149952712272,
-0.648233210226155));
#10007=CARTESIAN_POINT('Ctrl Pts',(7.55686827583247,-0.213925780275835,
-0.653466547804564));
#10008=CARTESIAN_POINT('Ctrl Pts',(7.47854745486387,-0.23960157726169,-0.658699885382972));
#10009=CARTESIAN_POINT('Ctrl Pts',(7.40022663389526,-0.265277374247545,
-0.663933222961381));
#10010=CARTESIAN_POINT('Ctrl Pts',(7.30810398658965,-0.248853140655693,
-0.669166560539789));
#10011=CARTESIAN_POINT('Ctrl Pts',(7.24348338090206,-0.197690572651982,
-0.674399898118197));
#10012=CARTESIAN_POINT('Ctrl Pts',(7.18445323964283,-0.150954185948262,
-0.679180488662399));
#10013=CARTESIAN_POINT('Ctrl Pts',(7.14837245587845,-0.0752300438529192,
-0.683961079206601));
#10014=CARTESIAN_POINT('Ctrl Pts',(7.14792656787638,0.000120390219947525,
-0.688741669750802));
#10015=CARTESIAN_POINT('Ctrl Pts',(7.14798283450166,-0.000154017160047509,
-0.661258330249198));
#10016=CARTESIAN_POINT('Ctrl Pts',(7.14791195819876,-0.00992057037260971,
-0.660639065125954));
#10017=CARTESIAN_POINT('Ctrl Pts',(7.14843167665666,-0.0196795166918168,
-0.660019800002709));
#10018=CARTESIAN_POINT('Ctrl Pts',(7.14956754906296,-0.0293662095570414,
-0.659400534879465));
#10019=CARTESIAN_POINT('Ctrl Pts',(7.15916667474439,-0.111227325061965,
-0.654167197301056));
#10020=CARTESIAN_POINT('Ctrl Pts',(7.21276993588987,-0.187928284107481,
-0.648933859722648));
#10021=CARTESIAN_POINT('Ctrl Pts',(7.28634387847187,-0.225080046990995,
-0.643700522144239));
#10022=CARTESIAN_POINT('Ctrl Pts',(7.35991782105388,-0.262231809874509,
-0.638467184565831));
#10023=CARTESIAN_POINT('Ctrl Pts',(7.45346244507241,-0.259834376596021,
-0.633233846987423));
#10024=CARTESIAN_POINT('Ctrl Pts',(7.52503665627896,-0.218962547126307,
-0.628000509409014));
#10025=CARTESIAN_POINT('Ctrl Pts',(7.59661086748551,-0.178090717656593,
-0.622767171830606));
#10026=CARTESIAN_POINT('Ctrl Pts',(7.64621466588009,-0.0987444919956527,
-0.617533834252197));
#10027=CARTESIAN_POINT('Ctrl Pts',(7.65160790755967,-0.0164991809676121,
-0.612300496673789));
#10028=CARTESIAN_POINT('Ctrl Pts',(7.65700114923926,0.0657461300604286,
-0.60706715909538));
#10029=CARTESIAN_POINT('Ctrl Pts',(7.61818383420385,0.15089052645557,-0.601833821516972));
#10030=CARTESIAN_POINT('Ctrl Pts',(7.55255991314267,0.20075913443422,-0.596600483938564));
#10031=CARTESIAN_POINT('Ctrl Pts',(7.48693599208148,0.25062774241287,-0.591367146360156));
#10032=CARTESIAN_POINT('Ctrl Pts',(7.39450546499451,0.26522056197503,-0.586133808781746));
#10033=CARTESIAN_POINT('Ctrl Pts',(7.31670999151327,0.23799482019678,-0.580900471203338));
#10034=CARTESIAN_POINT('Ctrl Pts',(7.23891451803204,0.21076907841853,-0.575667133624929));
#10035=CARTESIAN_POINT('Ctrl Pts',(7.17575409815654,0.14172477529987,-0.570433796046521));
#10036=CARTESIAN_POINT('Ctrl Pts',(7.15554701433853,0.0618182614198286,
-0.565200458468113));
#10037=CARTESIAN_POINT('Ctrl Pts',(7.15047320219045,0.0417544736666595,
-0.563886415728475));
#10038=CARTESIAN_POINT('Ctrl Pts',(7.14810745066301,0.0210058607540061,
-0.562572372988836));
#10039=CARTESIAN_POINT('Ctrl Pts',(7.14828831497717,0.000216666477491244,
-0.561258330249198));
#10040=CARTESIAN_POINT('Origin',(7.4,0.,-0.45));
#10041=CARTESIAN_POINT('',(7.14854579264603,-0.000143789217906781,-0.461258330249198));
#10042=CARTESIAN_POINT('',(7.14810500570899,-0.000198275220022497,-0.488741669750802));
#10043=CARTESIAN_POINT('',(7.14825,3.08304831685346E-17,-0.45));
#10044=CARTESIAN_POINT('Ctrl Pts',(7.14810500570899,-0.000198275220022497,
-0.488741669750802));
#10045=CARTESIAN_POINT('Ctrl Pts',(7.14869358833605,0.0680094416058214,
-0.493061032510774));
#10046=CARTESIAN_POINT('Ctrl Pts',(7.17744215705244,0.13665463081379,-0.497380395270747));
#10047=CARTESIAN_POINT('Ctrl Pts',(7.22690918325704,0.183353008080594,-0.501699758030719));
#10048=CARTESIAN_POINT('Ctrl Pts',(7.28684340538992,0.239932736661351,-0.506933095609127));
#10049=CARTESIAN_POINT('Ctrl Pts',(7.37719176882127,0.264295132469651,-0.512166433187535));
#10050=CARTESIAN_POINT('Ctrl Pts',(7.45744615163793,0.245517200446581,-0.517399770765944));
#10051=CARTESIAN_POINT('Ctrl Pts',(7.53770053445458,0.226739268423512,-0.522633108344352));
#10052=CARTESIAN_POINT('Ctrl Pts',(7.60786093665655,0.164821008569074,-0.527866445922761));
#10053=CARTESIAN_POINT('Ctrl Pts',(7.6364706049432,0.0875237657383382,-0.533099783501169));
#10054=CARTESIAN_POINT('Ctrl Pts',(7.66508027322986,0.0102265229076026,
-0.538333121079578));
#10055=CARTESIAN_POINT('Ctrl Pts',(7.65213920760121,-0.0824497028994303,
-0.543566458657986));
#10056=CARTESIAN_POINT('Ctrl Pts',(7.60344959777296,-0.148953073308844,
-0.548799796236394));
#10057=CARTESIAN_POINT('Ctrl Pts',(7.5547599879447,-0.215456443718259,-0.554033133814803));
#10058=CARTESIAN_POINT('Ctrl Pts',(7.47032183391684,-0.255786958730054,
-0.559266471393212));
#10059=CARTESIAN_POINT('Ctrl Pts',(7.38799338533328,-0.251862254589131,
-0.56449980897162));
#10060=CARTESIAN_POINT('Ctrl Pts',(7.30566493674973,-0.247937550448207,
-0.569733146550029));
#10061=CARTESIAN_POINT('Ctrl Pts',(7.22544619361049,-0.199757627154565,
-0.574966484128437));
#10062=CARTESIAN_POINT('Ctrl Pts',(7.18330361771556,-0.128924151937003,
-0.580199821706845));
#10063=CARTESIAN_POINT('Ctrl Pts',(7.16037526182527,-0.0903860442336708,
-0.583047104388164));
#10064=CARTESIAN_POINT('Ctrl Pts',(7.14871776187482,-0.0451423004661291,
-0.585894387069483));
#10065=CARTESIAN_POINT('Ctrl Pts',(7.14862473855677,5.66816876182724E-5,
-0.588741669750802));
#10066=CARTESIAN_POINT('Ctrl Pts',(7.14828831497717,0.000216666477491244,
-0.561258330249198));
#10067=CARTESIAN_POINT('Ctrl Pts',(7.14882776514237,-0.0617896742390719,
-0.557339035410428));
#10068=CARTESIAN_POINT('Ctrl Pts',(7.17202202015866,-0.124157028526609,
-0.553419740571658));
#10069=CARTESIAN_POINT('Ctrl Pts',(7.21358737716188,-0.16979132243042,-0.549500445732887));
#10070=CARTESIAN_POINT('Ctrl Pts',(7.26908857156377,-0.230725667759206,
-0.544267108154479));
#10071=CARTESIAN_POINT('Ctrl Pts',(7.35734470812808,-0.261825633775355,
-0.539033770576071));
#10072=CARTESIAN_POINT('Ctrl Pts',(7.438785725967,-0.249147400040112,-0.533800432997662));
#10073=CARTESIAN_POINT('Ctrl Pts',(7.52022674380592,-0.236469166304868,
-0.528567095419254));
#10074=CARTESIAN_POINT('Ctrl Pts',(7.59485264291945,-0.180012732818235,
-0.523333757840845));
#10075=CARTESIAN_POINT('Ctrl Pts',(7.62920454283812,-0.105090613084703,
-0.518100420262437));
#10076=CARTESIAN_POINT('Ctrl Pts',(7.66355644275679,-0.0301684933511692,
-0.512867082684028));
#10077=CARTESIAN_POINT('Ctrl Pts',(7.65763434348059,0.0632193126292629,
-0.50763374510562));
#10078=CARTESIAN_POINT('Ctrl Pts',(7.61409344694317,0.133201934451936,-0.502400407527211));
#10079=CARTESIAN_POINT('Ctrl Pts',(7.57055255040575,0.203184556274608,-0.497167069948803));
#10080=CARTESIAN_POINT('Ctrl Pts',(7.4893928566071,0.249761993939521,-0.491933732370395));
#10081=CARTESIAN_POINT('Ctrl Pts',(7.40700270341056,0.252051029665313,-0.486700394791986));
#10082=CARTESIAN_POINT('Ctrl Pts',(7.32461255021403,0.254340065391105,-0.481467057213578));
#10083=CARTESIAN_POINT('Ctrl Pts',(7.24099193761961,0.212340699177775,-0.476233719635169));
#10084=CARTESIAN_POINT('Ctrl Pts',(7.19363256847158,0.144883548419682,-0.471000382056761));
#10085=CARTESIAN_POINT('Ctrl Pts',(7.16424549499626,0.103025553234657,-0.46775303145424));
#10086=CARTESIAN_POINT('Ctrl Pts',(7.14882029032525,0.0513654052804403,
-0.464505680851719));
#10087=CARTESIAN_POINT('Ctrl Pts',(7.14854579264603,-0.000143789217906781,
-0.461258330249198));
#10088=CARTESIAN_POINT('Origin',(7.4,0.,-0.45));
#10089=CARTESIAN_POINT('',(7.14785287490956,-1.4768633667023E-5,-0.361258330249198));
#10090=CARTESIAN_POINT('',(7.14815269739345,0.000207923984461611,-0.388741669750802));
#10091=CARTESIAN_POINT('',(7.14825,3.08304831685346E-17,-0.45));
#10092=CARTESIAN_POINT('Ctrl Pts',(7.14815269739345,0.000207923984461611,
-0.388741669750802));
#10093=CARTESIAN_POINT('Ctrl Pts',(7.14801042171326,0.0163122622245923,
-0.389761002795248));
#10094=CARTESIAN_POINT('Ctrl Pts',(7.14942613596003,0.032391700678434,-0.390780335839695));
#10095=CARTESIAN_POINT('Ctrl Pts',(7.15249178151693,0.0481501620737753,
-0.391799668884141));
#10096=CARTESIAN_POINT('Ctrl Pts',(7.16823105160384,0.129055366361475,-0.39703300646255));
#10097=CARTESIAN_POINT('Ctrl Pts',(7.22746049691456,0.201500007211662,-0.402266344040958));
#10098=CARTESIAN_POINT('Ctrl Pts',(7.30362431153402,0.233003182380788,-0.407499681619367));
#10099=CARTESIAN_POINT('Ctrl Pts',(7.37978812615348,0.264506357549914,-0.412733019197775));
#10100=CARTESIAN_POINT('Ctrl Pts',(7.47288631008167,0.255068067037979,-0.417966356776183));
#10101=CARTESIAN_POINT('Ctrl Pts',(7.54117784598463,0.20892001369993,-0.423199694354592));
#10102=CARTESIAN_POINT('Ctrl Pts',(7.60946938188759,0.162771960361881,-0.428433031933));
#10103=CARTESIAN_POINT('Ctrl Pts',(7.65295426976532,0.0799141441977179,
-0.433666369511409));
#10104=CARTESIAN_POINT('Ctrl Pts',(7.65213585154447,-0.00250373552386811,
-0.438899707089817));
#10105=CARTESIAN_POINT('Ctrl Pts',(7.65131743332362,-0.0849216152454548,
-0.444133044668226));
#10106=CARTESIAN_POINT('Ctrl Pts',(7.6061957090042,-0.166899558524465,-0.449366382246634));
#10107=CARTESIAN_POINT('Ctrl Pts',(7.5370012201365,-0.211682361142448,-0.454599719825042));
#10108=CARTESIAN_POINT('Ctrl Pts',(7.46780673126879,-0.25646516376043,-0.459833057403451));
#10109=CARTESIAN_POINT('Ctrl Pts',(7.37453947785282,-0.264052825717385,
-0.46506639498186));
#10110=CARTESIAN_POINT('Ctrl Pts',(7.29901628031458,-0.231043382617906,
-0.470299732560268));
#10111=CARTESIAN_POINT('Ctrl Pts',(7.22349308277634,-0.198033939518426,
-0.475533070138677));
#10112=CARTESIAN_POINT('Ctrl Pts',(7.16571394111585,-0.12442739136251,-0.480766407717085));
#10113=CARTESIAN_POINT('Ctrl Pts',(7.15158441070281,-0.0432255866079445,
-0.485999745295493));
#10114=CARTESIAN_POINT('Ctrl Pts',(7.14911676270564,-0.029044119495361,
-0.486913720113929));
#10115=CARTESIAN_POINT('Ctrl Pts',(7.14798046194419,-0.0146309911242199,
-0.487827694932365));
#10116=CARTESIAN_POINT('Ctrl Pts',(7.14810500570899,-0.000198275220022497,
-0.488741669750802));
#10117=CARTESIAN_POINT('Ctrl Pts',(7.14854579264603,-0.000143789217906781,
-0.461258330249198));
#10118=CARTESIAN_POINT('Ctrl Pts',(7.14837791769732,-0.03164534292534,-0.459272343273311));
#10119=CARTESIAN_POINT('Ctrl Pts',(7.15387670503811,-0.0630904370724168,
-0.457286356297423));
#10120=CARTESIAN_POINT('Ctrl Pts',(7.16531408922188,-0.0922024005987424,
-0.455300369321535));
#10121=CARTESIAN_POINT('Ctrl Pts',(7.19545310482183,-0.168916263556222,
-0.450067031743127));
#10122=CARTESIAN_POINT('Ctrl Pts',(7.26682926172338,-0.229429054168326,
-0.444833694164719));
#10123=CARTESIAN_POINT('Ctrl Pts',(7.3474407176227,-0.246609572473441,-0.43960035658631));
#10124=CARTESIAN_POINT('Ctrl Pts',(7.42805217352202,-0.263790090778555,
-0.434367019007902));
#10125=CARTESIAN_POINT('Ctrl Pts',(7.5178989284191,-0.237638336776682,-0.429133681429493));
#10126=CARTESIAN_POINT('Ctrl Pts',(7.57669775877139,-0.179879574833401,
-0.423900343851085));
#10127=CARTESIAN_POINT('Ctrl Pts',(7.63549658912369,-0.122120812890119,
-0.418667006272676));
#10128=CARTESIAN_POINT('Ctrl Pts',(7.66324749493119,-0.0327550430054262,
-0.413433668694268));
#10129=CARTESIAN_POINT('Ctrl Pts',(7.64750822446396,0.0481501632372987,
-0.408200331115859));
#10130=CARTESIAN_POINT('Ctrl Pts',(7.63176895399672,0.129055369480023,-0.402966993537451));
#10131=CARTESIAN_POINT('Ctrl Pts',(7.57253950725476,0.20150001208078,-0.397733655959043));
#10132=CARTESIAN_POINT('Ctrl Pts',(7.49637569079484,0.233003188011166,-0.392500318380634));
#10133=CARTESIAN_POINT('Ctrl Pts',(7.42021187433493,0.264506363941552,-0.387266980802226));
#10134=CARTESIAN_POINT('Ctrl Pts',(7.32711368815708,0.255068073201566,-0.382033643223817));
#10135=CARTESIAN_POINT('Ctrl Pts',(7.25882215060389,0.208920018748368,-0.376800305645409));
#10136=CARTESIAN_POINT('Ctrl Pts',(7.19121804006457,0.16323649358247,-0.371619647180005));
#10137=CARTESIAN_POINT('Ctrl Pts',(7.14792368105538,0.0815785307526936,
-0.366438988714602));
#10138=CARTESIAN_POINT('Ctrl Pts',(7.14785287490956,-1.4768633667023E-5,
-0.361258330249198));
#10139=CARTESIAN_POINT('Origin',(7.4,0.,-0.45));
#10140=CARTESIAN_POINT('',(7.14851414192891,0.000162483299119997,-0.261258330249198));
#10141=CARTESIAN_POINT('',(7.1486107370081,-8.15071611798959E-5,-0.288741669750802));
#10142=CARTESIAN_POINT('',(7.14825,3.08304831685346E-17,-0.45));
#10143=CARTESIAN_POINT('Ctrl Pts',(7.1486107370081,-8.15071611798959E-5,
-0.288741669750802));
#10144=CARTESIAN_POINT('Ctrl Pts',(7.14874995825962,0.0467834254920333,
-0.291694310658131));
#10145=CARTESIAN_POINT('Ctrl Pts',(7.16134085284144,0.0937178459994653,
-0.29464695156546));
#10146=CARTESIAN_POINT('Ctrl Pts',(7.18590655823031,0.133201931233131,-0.297599592472789));
#10147=CARTESIAN_POINT('Ctrl Pts',(7.22944745371562,0.203184551364662,-0.302832930051197));
#10148=CARTESIAN_POINT('Ctrl Pts',(7.31060714555302,0.249761987904173,-0.308066267629606));
#10149=CARTESIAN_POINT('Ctrl Pts',(7.39299729675863,0.252051023574679,-0.313299605208015));
#10150=CARTESIAN_POINT('Ctrl Pts',(7.47538744796424,0.254340059245185,-0.318532942786423));
#10151=CARTESIAN_POINT('Ctrl Pts',(7.55900805853805,0.212340694046686,-0.323766280364831));
#10152=CARTESIAN_POINT('Ctrl Pts',(7.60636742654168,0.144883544918643,-0.32899961794324));
#10153=CARTESIAN_POINT('Ctrl Pts',(7.6537267945453,0.0774263957905979,-0.334232955521648));
#10154=CARTESIAN_POINT('Ctrl Pts',(7.66482491997874,-0.0154885372669925,
-0.339466293100057));
#10155=CARTESIAN_POINT('Ctrl Pts',(7.63468590510707,-0.0922023983707198,
-0.344699630678465));
#10156=CARTESIAN_POINT('Ctrl Pts',(7.6045468902354,-0.168916259474447,-0.349932968256874));
#10157=CARTESIAN_POINT('Ctrl Pts',(7.53317073505863,-0.229429048624311,
-0.355166305835282));
#10158=CARTESIAN_POINT('Ctrl Pts',(7.45255928110724,-0.246609566514272,
-0.360399643413691));
#10159=CARTESIAN_POINT('Ctrl Pts',(7.37194782715585,-0.263790084404232,
-0.365632980992099));
#10160=CARTESIAN_POINT('Ctrl Pts',(7.28210107442985,-0.237638331034289,
-0.370866318570508));
#10161=CARTESIAN_POINT('Ctrl Pts',(7.2233022454984,-0.179879570486712,-0.376099656148916));
#10162=CARTESIAN_POINT('Ctrl Pts',(7.17595606765367,-0.133370879775126,
-0.380313660682878));
#10163=CARTESIAN_POINT('Ctrl Pts',(7.14874087646276,-0.0663687015160148,
-0.38452766521684));
#10164=CARTESIAN_POINT('Ctrl Pts',(7.14815269739345,0.000207923984461611,
-0.388741669750802));
#10165=CARTESIAN_POINT('Ctrl Pts',(7.14785287490956,-1.4768633667023E-5,
-0.361258330249198));
#10166=CARTESIAN_POINT('Ctrl Pts',(7.14785215492291,-0.000844443600183524,
-0.361205651136193));
#10167=CARTESIAN_POINT('Ctrl Pts',(7.14785590411212,-0.00167411188070867,
-0.361152972023188));
#10168=CARTESIAN_POINT('Ctrl Pts',(7.14786414236282,-0.00250373558438578,
-0.361100292910184));
#10169=CARTESIAN_POINT('Ctrl Pts',(7.14868256060344,-0.0849216172975351,
-0.355866955331775));
#10170=CARTESIAN_POINT('Ctrl Pts',(7.19380428601321,-0.166899562557425,
-0.350633617753366));
#10171=CARTESIAN_POINT('Ctrl Pts',(7.26299877655295,-0.21168236625759,-0.345400280174958));
#10172=CARTESIAN_POINT('Ctrl Pts',(7.33219326709269,-0.256465169957754,
-0.340166942596549));
#10173=CARTESIAN_POINT('Ctrl Pts',(7.42546052276241,-0.264052832098196,
-0.334933605018141));
#10174=CARTESIAN_POINT('Ctrl Pts',(7.50098372212563,-0.231043388201001,
-0.329700267439733));
#10175=CARTESIAN_POINT('Ctrl Pts',(7.57650692148885,-0.198033944303807,
-0.324466929861324));
#10176=CARTESIAN_POINT('Ctrl Pts',(7.63428606454555,-0.124427394368975,
-0.319233592282916));
#10177=CARTESIAN_POINT('Ctrl Pts',(7.64841559530002,-0.0432255876523345,
-0.314000254704507));
#10178=CARTESIAN_POINT('Ctrl Pts',(7.66254512605448,0.0379762190643056,
-0.308766917126099));
#10179=CARTESIAN_POINT('Ctrl Pts',(7.63302504450671,0.126773282562755,-0.303533579547691));
#10180=CARTESIAN_POINT('Ctrl Pts',(7.57309082092558,0.183353012510955,-0.298300241969282));
#10181=CARTESIAN_POINT('Ctrl Pts',(7.51315659734445,0.239932742459157,-0.293066904390874));
#10182=CARTESIAN_POINT('Ctrl Pts',(7.42280823172995,0.264295138857109,-0.287833566812465));
#10183=CARTESIAN_POINT('Ctrl Pts',(7.34255384697395,0.245517206379848,-0.282600229234057));
#10184=CARTESIAN_POINT('Ctrl Pts',(7.26229946221796,0.226739273902587,-0.277366891655648));
#10185=CARTESIAN_POINT('Ctrl Pts',(7.19213905832046,0.164821012550114,-0.27213355407724));
#10186=CARTESIAN_POINT('Ctrl Pts',(7.16352938934256,0.0875237678523623,
-0.266900216498831));
#10187=CARTESIAN_POINT('Ctrl Pts',(7.15324834685328,0.059746576244338,-0.265019587748954));
#10188=CARTESIAN_POINT('Ctrl Pts',(7.14833301628059,0.0299833982425618,
-0.263138958999076));
#10189=CARTESIAN_POINT('Ctrl Pts',(7.14851414192891,0.000162483299119997,
-0.261258330249198));
#10190=CARTESIAN_POINT('Origin',(7.4,0.,-0.45));
#10191=CARTESIAN_POINT('',(7.1483354802531,-0.000213511019231185,-0.161258330249198));
#10192=CARTESIAN_POINT('',(7.14789741337032,-9.36993803829212E-5,-0.188741669750802));
#10193=CARTESIAN_POINT('',(7.14825,3.08304831685346E-17,-0.45));
#10194=CARTESIAN_POINT('Ctrl Pts',(7.14789741337032,-9.36993803829212E-5,
-0.188741669750802));
#10195=CARTESIAN_POINT('Ctrl Pts',(7.14827035947299,0.0768944579770298,
-0.193627618521014));
#10196=CARTESIAN_POINT('Ctrl Pts',(7.18617228508483,0.154200799589981,-0.198513567291225));
#10197=CARTESIAN_POINT('Ctrl Pts',(7.24744009054551,0.200759129579989,-0.203399516061437));
#10198=CARTESIAN_POINT('Ctrl Pts',(7.31306401002228,0.250627736350931,-0.208632853639845));
#10199=CARTESIAN_POINT('Ctrl Pts',(7.40549453487257,0.2652205555663,-0.213866191218254));
#10200=CARTESIAN_POINT('Ctrl Pts',(7.48329000647319,0.23799481444734,-0.219099528796662));
#10201=CARTESIAN_POINT('Ctrl Pts',(7.56108547807381,0.21076907332838,-0.224332866375071));
#10202=CARTESIAN_POINT('Ctrl Pts',(7.62424589642476,0.141724771875092,-0.229566203953479));
#10203=CARTESIAN_POINT('Ctrl Pts',(7.64445297975488,0.061818259925214,-0.234799541531888));
#10204=CARTESIAN_POINT('Ctrl Pts',(7.66466006308499,-0.0180882520246644,
-0.240032879110296));
#10205=CARTESIAN_POINT('Ctrl Pts',(7.64191381139426,-0.108856974471133,
-0.245266216688705));
#10206=CARTESIAN_POINT('Ctrl Pts',(7.58641261833332,-0.169791318327095,
-0.250499554267113));
#10207=CARTESIAN_POINT('Ctrl Pts',(7.53091142527237,-0.230725662183056,
-0.255732891845522));
#10208=CARTESIAN_POINT('Ctrl Pts',(7.4426552908412,-0.261825627448513,-0.26096622942393));
#10209=CARTESIAN_POINT('Ctrl Pts',(7.36121427497037,-0.24914739401983,-0.266199567002338));
#10210=CARTESIAN_POINT('Ctrl Pts',(7.27977325909954,-0.236469160591147,
-0.271432904580747));
#10211=CARTESIAN_POINT('Ctrl Pts',(7.20514736178904,-0.180012728468324,
-0.276666242159155));
#10212=CARTESIAN_POINT('Ctrl Pts',(7.1707954627004,-0.105090610545136,-0.281899579737564));
#10213=CARTESIAN_POINT('Ctrl Pts',(7.15582485155161,-0.0724394348131096,
-0.284180276408643));
#10214=CARTESIAN_POINT('Ctrl Pts',(7.14850319889059,-0.0362812006719064,
-0.286460973079723));
#10215=CARTESIAN_POINT('Ctrl Pts',(7.1486107370081,-8.15071611798959E-5,
-0.288741669750802));
#10216=CARTESIAN_POINT('Ctrl Pts',(7.14851414192891,0.000162483299119997,
-0.261258330249198));
#10217=CARTESIAN_POINT('Ctrl Pts',(7.1488370454048,-0.0530010370459997,
-0.257905621420668));
#10218=CARTESIAN_POINT('Ctrl Pts',(7.16535766681591,-0.106348058760499,
-0.254552912592137));
#10219=CARTESIAN_POINT('Ctrl Pts',(7.19655039731096,-0.148953076906415,
-0.251200203763606));
#10220=CARTESIAN_POINT('Ctrl Pts',(7.24524000831559,-0.21545644892441,-0.245966866185198));
#10221=CARTESIAN_POINT('Ctrl Pts',(7.32967816438315,-0.255786964917369,
-0.240733528606789));
#10222=CARTESIAN_POINT('Ctrl Pts',(7.41200661495652,-0.251862260678651,
-0.235500191028381));
#10223=CARTESIAN_POINT('Ctrl Pts',(7.49433506552989,-0.247937556439932,
-0.230266853449972));
#10224=CARTESIAN_POINT('Ctrl Pts',(7.57455381060907,-0.199757631969536,
-0.225033515871564));
#10225=CARTESIAN_POINT('Ctrl Pts',(7.61669638752149,-0.128924155045882,
-0.219800178293155));
#10226=CARTESIAN_POINT('Ctrl Pts',(7.65883896443392,-0.0580906781222288,
-0.214566840714747));
#10227=CARTESIAN_POINT('Ctrl Pts',(7.66290537317959,0.0353963512546822,
-0.209333503136338));
#10228=CARTESIAN_POINT('Ctrl Pts',(7.62707242700085,0.109621509538064,-0.20410016555793));
#10229=CARTESIAN_POINT('Ctrl Pts',(7.59123948082212,0.183846667821447,-0.198866827979521));
#10230=CARTESIAN_POINT('Ctrl Pts',(7.51550717971897,0.238809955011301,-0.193633490401113));
#10231=CARTESIAN_POINT('Ctrl Pts',(7.43383044982246,0.249868449747252,-0.188400152822705));
#10232=CARTESIAN_POINT('Ctrl Pts',(7.35215371992594,0.260926944483204,-0.183166815244296));
#10233=CARTESIAN_POINT('Ctrl Pts',(7.26453256123606,0.228080646765252,-0.177933477665888));
#10234=CARTESIAN_POINT('Ctrl Pts',(7.2102523694764,0.166056085274717,-0.172700140087479));
#10235=CARTESIAN_POINT('Ctrl Pts',(7.17069420843708,0.120854004878616,-0.168886203474719));
#10236=CARTESIAN_POINT('Ctrl Pts',(7.14884397070955,0.0601548797106173,
-0.165072266861959));
#10237=CARTESIAN_POINT('Ctrl Pts',(7.1483354802531,-0.000213511019231185,
-0.161258330249198));
#10238=CARTESIAN_POINT('Origin',(7.4,0.,-0.45));
#10239=CARTESIAN_POINT('',(7.14794643808389,0.00012639595204536,-0.0612583302491982));
#10240=CARTESIAN_POINT('',(7.14840641220525,0.000201202115797984,-0.0887416697508019));
#10241=CARTESIAN_POINT('',(7.14825,3.08304831685346E-17,-0.45));
#10242=CARTESIAN_POINT('',(7.59134659966651,0.163598720337495,0.));
#10243=CARTESIAN_POINT('Ctrl Pts',(7.14794643808389,0.00012639595204536,
-0.0612583302491982));
#10244=CARTESIAN_POINT('Ctrl Pts',(7.14842546082296,-0.0742619964396601,
-0.0565388995680243));
#10245=CARTESIAN_POINT('Ctrl Pts',(7.18347141764068,-0.149027219123109,
-0.0518194688868503));
#10246=CARTESIAN_POINT('Ctrl Pts',(7.24121260951448,-0.195852567382474,
-0.0471000382056764));
#10247=CARTESIAN_POINT('Ctrl Pts',(7.3052413387552,-0.247776808084922,-0.0418667006272679));
#10248=CARTESIAN_POINT('Ctrl Pts',(7.39717705575739,-0.265345038299558,
-0.0366333630488594));
#10249=CARTESIAN_POINT('Ctrl Pts',(7.47578474042289,-0.240530500580791,
-0.0314000254704509));
#10250=CARTESIAN_POINT('Ctrl Pts',(7.55439242508838,-0.215715962862024,
-0.0261666878920425));
#10251=CARTESIAN_POINT('Ctrl Pts',(7.61967207741718,-0.148518657209854,
-0.020933350313634));
#10252=CARTESIAN_POINT('Ctrl Pts',(7.64235926604704,-0.0694196478813939,
-0.0157000127352255));
#10253=CARTESIAN_POINT('Ctrl Pts',(7.66504645467691,0.00967936144706648,
-0.010466675156817));
#10254=CARTESIAN_POINT('Ctrl Pts',(7.64514117960785,0.100680074451818,-0.00523333757840849));
#10255=CARTESIAN_POINT('Ctrl Pts',(7.59134659966651,0.163598720337495,0.));
#10256=CARTESIAN_POINT('',(7.20829763049428,0.163827060994237,1.44778665420313E-16));
#10257=CARTESIAN_POINT('Origin',(7.4,0.,0.));
#10258=CARTESIAN_POINT('Ctrl Pts',(7.20829596415884,0.1638281304838,9.0205620750794E-17));
#10259=CARTESIAN_POINT('Ctrl Pts',(7.2596674427612,0.223538347845456,-0.00499978774624422));
#10260=CARTESIAN_POINT('Ctrl Pts',(7.3414071265269,0.257577506526122,-0.00999957549248853));
#10261=CARTESIAN_POINT('Ctrl Pts',(7.41991797435699,0.25134623940458,-0.0149993632387328));
#10262=CARTESIAN_POINT('Ctrl Pts',(7.50209621693749,0.24482389764862,-0.0202327008171413));
#10263=CARTESIAN_POINT('Ctrl Pts',(7.58073692780066,0.19418103958705,-0.0254660383955497));
#10264=CARTESIAN_POINT('Ctrl Pts',(7.62062911488364,0.122067692861168,-0.0306993759739582));
#10265=CARTESIAN_POINT('Ctrl Pts',(7.66052130196662,0.049954346135286,-0.0359327135523666));
#10266=CARTESIAN_POINT('Ctrl Pts',(7.6616649652694,-0.0436294892549086,
-0.0411660511307751));
#10267=CARTESIAN_POINT('Ctrl Pts',(7.62352358784103,-0.116697418725104,
-0.0463993887091835));
#10268=CARTESIAN_POINT('Ctrl Pts',(7.58538221041266,-0.1897653481953,-0.051632726287592));
#10269=CARTESIAN_POINT('Ctrl Pts',(7.50795579225314,-0.242317371745497,
-0.0568660638660004));
#10270=CARTESIAN_POINT('Ctrl Pts',(7.42597061249076,-0.250805231205967,
-0.0620994014444088));
#10271=CARTESIAN_POINT('Ctrl Pts',(7.34398543272838,-0.259293090666436,
-0.0673327390228173));
#10272=CARTESIAN_POINT('Ctrl Pts',(7.25744149136314,-0.223716786037178,
-0.0725660766012258));
#10273=CARTESIAN_POINT('Ctrl Pts',(7.20513534285944,-0.160020335565283,
-0.0777994141796342));
#10274=CARTESIAN_POINT('Ctrl Pts',(7.16868013390367,-0.11562656010828,-0.0814468327033568));
#10275=CARTESIAN_POINT('Ctrl Pts',(7.14885596689451,-0.0575733958307166,
-0.0850942512270793));
#10276=CARTESIAN_POINT('Ctrl Pts',(7.14840641220525,0.000201202115797984,
-0.0887416697508019));
#10277=CARTESIAN_POINT('Origin',(-7.4,0.,-0.45));
#10278=CARTESIAN_POINT('',(-7.65135844136173,-9.87909931464411E-6,-0.761258330249198));
#10279=CARTESIAN_POINT('',(-7.6515844849848,-0.000333784136707353,-0.788741669750802));
#10280=CARTESIAN_POINT('',(-7.65175,3.08304831685346E-17,-0.45));
#10281=CARTESIAN_POINT('',(-7.59134659966651,0.163598720337494,-0.8));
#10282=CARTESIAN_POINT('Ctrl Pts',(-7.6515844849848,-0.000333784136707353,
-0.788741669750802));
#10283=CARTESIAN_POINT('Ctrl Pts',(-7.65107118775856,0.0589216006363537,
-0.792494446500534));
#10284=CARTESIAN_POINT('Ctrl Pts',(-7.62992218280841,0.118480356030438,
-0.796247223250267));
#10285=CARTESIAN_POINT('Ctrl Pts',(-7.59134659966651,0.163598720337491,
-0.8));
#10286=CARTESIAN_POINT('',(-7.20829765525586,0.163827077455369,-0.799999999999998));
#10287=CARTESIAN_POINT('Origin',(-7.4,0.,-0.8));
#10288=CARTESIAN_POINT('Ctrl Pts',(-7.2082959906101,0.163828146011844,-0.799999999999999));
#10289=CARTESIAN_POINT('Ctrl Pts',(-7.25966747611426,0.22353839593213,-0.795000212253755));
#10290=CARTESIAN_POINT('Ctrl Pts',(-7.34140714099376,0.257577466209252,
-0.790000424507512));
#10291=CARTESIAN_POINT('Ctrl Pts',(-7.4199179741645,0.251346180862741,-0.785000636761268));
#10292=CARTESIAN_POINT('Ctrl Pts',(-7.50209620140088,0.244823820030488,
-0.779767299182859));
#10293=CARTESIAN_POINT('Ctrl Pts',(-7.58073690155091,0.194181019780683,
-0.77453396160445));
#10294=CARTESIAN_POINT('Ctrl Pts',(-7.62062908494217,0.122067693270255,
-0.769300624026042));
#10295=CARTESIAN_POINT('Ctrl Pts',(-7.64106375997351,0.0851278151438433,
-0.76661985943376));
#10296=CARTESIAN_POINT('Ctrl Pts',(-7.65133091722897,0.0425541224698544,
-0.763939094841479));
#10297=CARTESIAN_POINT('Ctrl Pts',(-7.65135844136173,-9.87909931464411E-6,
-0.761258330249198));
#10298=CARTESIAN_POINT('Origin',(-7.4,0.,-0.45));
#10299=CARTESIAN_POINT('',(-7.65201712840627,-0.000154017282173287,-0.661258330249199));
#10300=CARTESIAN_POINT('',(-7.65207346276915,0.000120387280643822,-0.688741669750802));
#10301=CARTESIAN_POINT('',(-7.65175,3.08304831685346E-17,-0.45));
#10302=CARTESIAN_POINT('Ctrl Pts',(-7.65207346276915,0.000120387280643822,
-0.688741669750802));
#10303=CARTESIAN_POINT('Ctrl Pts',(-7.65211569074847,0.00725647012215086,
-0.689194416785009));
#10304=CARTESIAN_POINT('Ctrl Pts',(-7.65183830629956,0.014389201188033,
-0.689647163819216));
#10305=CARTESIAN_POINT('Ctrl Pts',(-7.65123053408043,0.0214936402840764,
-0.690099910853423));
#10306=CARTESIAN_POINT('Ctrl Pts',(-7.64420524853858,0.103614394890392,
-0.695333248431831));
#10307=CARTESIAN_POINT('Ctrl Pts',(-7.59303611022166,0.181954995799164,
-0.700566586010239));
#10308=CARTESIAN_POINT('Ctrl Pts',(-7.52066407726933,0.221399944694366,
-0.705799923588648));
#10309=CARTESIAN_POINT('Ctrl Pts',(-7.44829204431699,0.260844893589568,
-0.711033261167056));
#10310=CARTESIAN_POINT('Ctrl Pts',(-7.35471711672925,0.261394190471199,
-0.716266598745465));
#10311=CARTESIAN_POINT('Ctrl Pts',(-7.2818960197261,0.222783627398016,-0.721499936323873));
#10312=CARTESIAN_POINT('Ctrl Pts',(-7.20907492272296,0.184173064324832,
-0.726733273902282));
#10313=CARTESIAN_POINT('Ctrl Pts',(-7.15700765630441,0.106402641296834,
-0.73196661148069));
#10314=CARTESIAN_POINT('Ctrl Pts',(-7.14903488410923,0.0243772822946468,
-0.737199949059099));
#10315=CARTESIAN_POINT('Ctrl Pts',(-7.14106211191404,-0.0576480767075406,
-0.742433286637507));
#10316=CARTESIAN_POINT('Ctrl Pts',(-7.17718383394222,-0.143928371683915,
-0.747666624215915));
#10317=CARTESIAN_POINT('Ctrl Pts',(-7.24121258230851,-0.195852606685422,
-0.752899961794324));
#10318=CARTESIAN_POINT('Ctrl Pts',(-7.3052413306748,-0.247776841686928,
-0.758133299372732));
#10319=CARTESIAN_POINT('Ctrl Pts',(-7.3971771053792,-0.265345016713566,
-0.763366636951141));
#10320=CARTESIAN_POINT('Ctrl Pts',(-7.47578476199579,-0.240530505659223,
-0.768599974529549));
#10321=CARTESIAN_POINT('Ctrl Pts',(-7.55439241861237,-0.215715994604879,
-0.773833312107958));
#10322=CARTESIAN_POINT('Ctrl Pts',(-7.61967195714114,-0.148518797469554,
-0.779066649686366));
#10323=CARTESIAN_POINT('Ctrl Pts',(-7.64235914739001,-0.0694197802053813,
-0.784299987264774));
#10324=CARTESIAN_POINT('Ctrl Pts',(-7.64877756865406,-0.0470419181253069,
-0.78578054809345));
#10325=CARTESIAN_POINT('Ctrl Pts',(-7.65178699310541,-0.0237114608368644,
-0.787261108922126));
#10326=CARTESIAN_POINT('Ctrl Pts',(-7.6515844849848,-0.000333784136707353,
-0.788741669750802));
#10327=CARTESIAN_POINT('Ctrl Pts',(-7.65135844136173,-9.87909931464411E-6,
-0.761258330249198));
#10328=CARTESIAN_POINT('Ctrl Pts',(-7.65138464931672,-0.040538510706789,
-0.758705757263071));
#10329=CARTESIAN_POINT('Ctrl Pts',(-7.64212710855812,-0.0810583558879505,
-0.756153184276944));
#10330=CARTESIAN_POINT('Ctrl Pts',(-7.62352356237588,-0.116697412903133,
-0.753600611290817));
#10331=CARTESIAN_POINT('Ctrl Pts',(-7.58538218978582,-0.189765339795041,
-0.748367273712409));
#10332=CARTESIAN_POINT('Ctrl Pts',(-7.50795577797319,-0.242317340807806,
-0.743133936134));
#10333=CARTESIAN_POINT('Ctrl Pts',(-7.42597060788136,-0.250805195601303,
-0.737900598555591));
#10334=CARTESIAN_POINT('Ctrl Pts',(-7.34398543778953,-0.2592930503948,-0.732667260977183));
#10335=CARTESIAN_POINT('Ctrl Pts',(-7.25744150941849,-0.22371675896903,
-0.727433923398775));
#10336=CARTESIAN_POINT('Ctrl Pts',(-7.20513536776807,-0.160020318362261,
-0.722200585820366));
#10337=CARTESIAN_POINT('Ctrl Pts',(-7.15282922611764,-0.0963238777554929,
-0.716967248241958));
#10338=CARTESIAN_POINT('Ctrl Pts',(-7.13476087118783,-0.00450728796772577,
-0.711733910663549));
#10339=CARTESIAN_POINT('Ctrl Pts',(-7.15903423279356,0.0742596685861753,
-0.706500573085141));
#10340=CARTESIAN_POINT('Ctrl Pts',(-7.1833075943993,0.153026625140077,-0.701267235506732));
#10341=CARTESIAN_POINT('Ctrl Pts',(-7.24992267254058,0.218743948460114,
-0.696033897928324));
#10342=CARTESIAN_POINT('Ctrl Pts',(-7.32901084118502,0.241948634523276,
-0.690800560349916));
#10343=CARTESIAN_POINT('Ctrl Pts',(-7.40809900982946,0.265153320586438,
-0.685567222771507));
#10344=CARTESIAN_POINT('Ctrl Pts',(-7.49966026897706,0.245845369392726,
-0.680333885193098));
#10345=CARTESIAN_POINT('Ctrl Pts',(-7.56264340109525,0.192680763788563,
-0.67510054761469));
#10346=CARTESIAN_POINT('Ctrl Pts',(-7.61817368758881,0.145807169522468,
-0.670486475159526));
#10347=CARTESIAN_POINT('Ctrl Pts',(-7.65148903726443,0.0726154250913533,
-0.665872402704363));
#10348=CARTESIAN_POINT('Ctrl Pts',(-7.65201712840627,-0.000154017282173287,
-0.661258330249199));
#10349=CARTESIAN_POINT('Origin',(-7.4,0.,-0.45));
#10350=CARTESIAN_POINT('',(-7.65171164790384,0.000216666439528223,-0.561258330249198));
#10351=CARTESIAN_POINT('',(-7.6513752928688,5.66816418782093E-5,-0.588741669750802));
#10352=CARTESIAN_POINT('',(-7.65175,3.08304831685346E-17,-0.45));
#10353=CARTESIAN_POINT('Ctrl Pts',(-7.6513752928688,5.66816418782093E-5,
-0.588741669750802));
#10354=CARTESIAN_POINT('Ctrl Pts',(-7.65145324746199,0.0379339415427937,
-0.591127724647891));
#10355=CARTESIAN_POINT('Ctrl Pts',(-7.64340989881181,0.0757797670326688,
-0.593513779544981));
#10356=CARTESIAN_POINT('Ctrl Pts',(-7.62707244990212,0.109621520545763,
-0.59589983444207));
#10357=CARTESIAN_POINT('Ctrl Pts',(-7.59123950011597,0.183846686360407,
-0.601133172020479));
#10358=CARTESIAN_POINT('Ctrl Pts',(-7.51550719140105,0.238809979279913,
-0.606366509598887));
#10359=CARTESIAN_POINT('Ctrl Pts',(-7.43383045324891,0.249868475051116,
-0.611599847177296));
#10360=CARTESIAN_POINT('Ctrl Pts',(-7.35215371509677,0.260926970822319,
-0.616833184755704));
#10361=CARTESIAN_POINT('Ctrl Pts',(-7.2645325475074,0.22808066944522,-0.622066522334113));
#10362=CARTESIAN_POINT('Ctrl Pts',(-7.21025235030538,0.166056101845713,
-0.627299859912521));
#10363=CARTESIAN_POINT('Ctrl Pts',(-7.15597215310335,0.104031534246204,
-0.63253319749093));
#10364=CARTESIAN_POINT('Ctrl Pts',(-7.13503292628866,0.0128287004242853,
-0.637766535069338));
#10365=CARTESIAN_POINT('Ctrl Pts',(-7.15682281406447,-0.0666606352401807,
-0.642999872647747));
#10366=CARTESIAN_POINT('Ctrl Pts',(-7.17861270184028,-0.146149970904647,
-0.648233210226155));
#10367=CARTESIAN_POINT('Ctrl Pts',(-7.24313170420659,-0.21392580841166,
-0.653466547804563));
#10368=CARTESIAN_POINT('Ctrl Pts',(-7.32145253515356,-0.23960160800038,
-0.658699885382972));
#10369=CARTESIAN_POINT('Ctrl Pts',(-7.39977336610052,-0.2652774075891,-0.66393322296138));
#10370=CARTESIAN_POINT('Ctrl Pts',(-7.49189602562815,-0.248853169259528,
-0.669166560539789));
#10371=CARTESIAN_POINT('Ctrl Pts',(-7.55651663900859,-0.197690595942813,
-0.674399898118197));
#10372=CARTESIAN_POINT('Ctrl Pts',(-7.61554678729514,-0.150954204385727,
-0.679180488662399));
#10373=CARTESIAN_POINT('Ctrl Pts',(-7.65162757430742,-0.0752300569569674,
-0.6839610792066));
#10374=CARTESIAN_POINT('Ctrl Pts',(-7.65207346276915,0.000120387280643822,
-0.688741669750802));
#10375=CARTESIAN_POINT('Ctrl Pts',(-7.65201712840627,-0.000154017282173287,
-0.661258330249199));
#10376=CARTESIAN_POINT('Ctrl Pts',(-7.65208800471547,-0.00992056909464737,
-0.660639065125954));
#10377=CARTESIAN_POINT('Ctrl Pts',(-7.65156828634817,-0.0196795140086419,
-0.66001980000271));
#10378=CARTESIAN_POINT('Ctrl Pts',(-7.65043241411917,-0.0293662054698359,
-0.659400534879465));
#10379=CARTESIAN_POINT('Ctrl Pts',(-7.6408332899361,-0.11122730910946,-0.654167197301057));
#10380=CARTESIAN_POINT('Ctrl Pts',(-7.58723003648116,-0.187928256374095,
-0.648933859722648));
#10381=CARTESIAN_POINT('Ctrl Pts',(-7.5136561047022,-0.225080013667832,
-0.643700522144239));
#10382=CARTESIAN_POINT('Ctrl Pts',(-7.44008217292323,-0.26223177096157,
-0.638467184565831));
#10383=CARTESIAN_POINT('Ctrl Pts',(-7.34653756282023,-0.25983433828441,
-0.633233846987423));
#10384=CARTESIAN_POINT('Ctrl Pts',(-7.27496336219634,-0.218962514901155,
-0.628000509409015));
#10385=CARTESIAN_POINT('Ctrl Pts',(-7.20338916157245,-0.178090691517901,
-0.622767171830606));
#10386=CARTESIAN_POINT('Ctrl Pts',(-7.15378537042767,-0.0987444774285509,
-0.617533834252197));
#10387=CARTESIAN_POINT('Ctrl Pts',(-7.14839212952851,-0.0164991784990361,
-0.612300496673789));
#10388=CARTESIAN_POINT('Ctrl Pts',(-7.14299888862934,0.0657461204304788,
-0.60706715909538));
#10389=CARTESIAN_POINT('Ctrl Pts',(-7.1818161979758,0.150890504200159,-0.601833821516972));
#10390=CARTESIAN_POINT('Ctrl Pts',(-7.24744010936701,0.200759104807884,
-0.596600483938564));
#10391=CARTESIAN_POINT('Ctrl Pts',(-7.31306402075823,0.250627705415608,
-0.591367146360155));
#10392=CARTESIAN_POINT('Ctrl Pts',(-7.40549453419421,0.265220522861378,
-0.586133808781746));
#10393=CARTESIAN_POINT('Ctrl Pts',(-7.4832899961977,0.23799478510693,-0.580900471203338));
#10394=CARTESIAN_POINT('Ctrl Pts',(-7.56108545820118,0.210769047352483,
-0.575667133624929));
#10395=CARTESIAN_POINT('Ctrl Pts',(-7.62424586877218,0.141724754397818,
-0.570433796046521));
#10396=CARTESIAN_POINT('Ctrl Pts',(-7.64445294961248,0.0618182522979024,
-0.565200458468113));
#10397=CARTESIAN_POINT('Ctrl Pts',(-7.64952676101288,0.0417544675026141,
-0.563886415728475));
#10398=CARTESIAN_POINT('Ctrl Pts',(-7.65189251219152,0.0210058576497331,
-0.562572372988837));
#10399=CARTESIAN_POINT('Ctrl Pts',(-7.65171164790384,0.000216666439528223,
-0.561258330249198));
#10400=CARTESIAN_POINT('Origin',(-7.4,0.,-0.45));
#10401=CARTESIAN_POINT('',(-7.65145417026957,-0.000143789196739241,-0.461258330249198));
#10402=CARTESIAN_POINT('',(-7.65189502578968,-0.000198275244604145,-0.488741669750802));
#10403=CARTESIAN_POINT('',(-7.65175,3.08304831685346E-17,-0.45));
#10404=CARTESIAN_POINT('Ctrl Pts',(-7.65189502578968,-0.000198275244604145,
-0.488741669750802));
#10405=CARTESIAN_POINT('Ctrl Pts',(-7.65130644308897,0.068009450109477,
-0.493061032510774));
#10406=CARTESIAN_POINT('Ctrl Pts',(-7.62255787077756,0.13665464789974,-0.497380395270746));
#10407=CARTESIAN_POINT('Ctrl Pts',(-7.57309083838734,0.183353031006997,
-0.501699758030718));
#10408=CARTESIAN_POINT('Ctrl Pts',(-7.51315660875997,0.239932766664044,
-0.506933095609127));
#10409=CARTESIAN_POINT('Ctrl Pts',(-7.4228082340312,0.264295165523682,-0.512166433187536));
#10410=CARTESIAN_POINT('Ctrl Pts',(-7.34255384117878,0.245517231150252,
-0.517399770765944));
#10411=CARTESIAN_POINT('Ctrl Pts',(-7.26229944832636,0.226739296776823,
-0.522633108344353));
#10412=CARTESIAN_POINT('Ctrl Pts',(-7.19213903735029,0.164821029170327,
-0.527866445922761));
#10413=CARTESIAN_POINT('Ctrl Pts',(-7.16352936548653,0.0875237766780772,
-0.533099783501169));
#10414=CARTESIAN_POINT('Ctrl Pts',(-7.13491969362278,0.0102265241858273,
-0.538333121079577));
#10415=CARTESIAN_POINT('Ctrl Pts',(-7.14786076087134,-0.0824497131921767,
-0.543566458657986));
#10416=CARTESIAN_POINT('Ctrl Pts',(-7.19655037678711,-0.148953091925709,
-0.548799796236394));
#10417=CARTESIAN_POINT('Ctrl Pts',(-7.24523999270288,-0.215456470659241,
-0.554033133814803));
#10418=CARTESIAN_POINT('Ctrl Pts',(-7.32967815728587,-0.255786990748301,
-0.559266471393211));
#10419=CARTESIAN_POINT('Ctrl Pts',(-7.41200661616639,-0.251862286101345,
-0.56449980897162));
#10420=CARTESIAN_POINT('Ctrl Pts',(-7.49433507504691,-0.247937581454389,
-0.569733146550028));
#10421=CARTESIAN_POINT('Ctrl Pts',(-7.57455382822498,-0.199757652071417,
-0.574966484128437));
#10422=CARTESIAN_POINT('Ctrl Pts',(-7.61669640938532,-0.12892416802504,
-0.580199821706845));
#10423=CARTESIAN_POINT('Ctrl Pts',(-7.63962476814035,-0.090386055518247,
-0.583047104388164));
#10424=CARTESIAN_POINT('Ctrl Pts',(-7.65128226954256,-0.0451423061363344,
-0.585894387069483));
#10425=CARTESIAN_POINT('Ctrl Pts',(-7.6513752928688,5.66816418782093E-5,
-0.588741669750802));
#10426=CARTESIAN_POINT('Ctrl Pts',(-7.65171164790384,0.000216666439528223,
-0.561258330249198));
#10427=CARTESIAN_POINT('Ctrl Pts',(-7.65117219781758,-0.0617896651313866,
-0.557339035410428));
#10428=CARTESIAN_POINT('Ctrl Pts',(-7.62797794621862,-0.124157010215117,
-0.553419740571658));
#10429=CARTESIAN_POINT('Ctrl Pts',(-7.58641259534448,-0.169791297387043,
-0.549500445732887));
#10430=CARTESIAN_POINT('Ctrl Pts',(-7.5309114091266,-0.23072563372691,-0.544267108154479));
#10431=CARTESIAN_POINT('Ctrl Pts',(-7.44265528558124,-0.261825595161477,
-0.539033770576071));
#10432=CARTESIAN_POINT('Ctrl Pts',(-7.36121427975392,-0.249147363297231,
-0.533800432997662));
#10433=CARTESIAN_POINT('Ctrl Pts',(-7.2797732739266,-0.236469131432985,
-0.528567095419254));
#10434=CARTESIAN_POINT('Ctrl Pts',(-7.20514738581732,-0.180012706269927,
-0.523333757840845));
#10435=CARTESIAN_POINT('Ctrl Pts',(-7.1707954909645,-0.105090597585267,
-0.518100420262437));
#10436=CARTESIAN_POINT('Ctrl Pts',(-7.13644359611167,-0.0301684889006052,
-0.512867082684028));
#10437=CARTESIAN_POINT('Ctrl Pts',(-7.14236569451531,0.0632193033056596,
-0.50763374510562));
#10438=CARTESIAN_POINT('Ctrl Pts',(-7.18590658463152,0.133201914806981,
-0.502400407527211));
#10439=CARTESIAN_POINT('Ctrl Pts',(-7.22944747474773,0.203184526308302,
-0.497167069948803));
#10440=CARTESIAN_POINT('Ctrl Pts',(-7.31060715657653,0.24976195710468,-0.491933732370395));
#10441=CARTESIAN_POINT('Ctrl Pts',(-7.39299729762207,0.252050992493053,
-0.486700394791986));
#10442=CARTESIAN_POINT('Ctrl Pts',(-7.47538743866762,0.254340027881427,
-0.481467057213578));
#10443=CARTESIAN_POINT('Ctrl Pts',(-7.55900803892991,0.212340667861795,
-0.476233719635169));
#10444=CARTESIAN_POINT('Ctrl Pts',(-7.60636740109344,0.144883527052185,
-0.471000382056761));
#10445=CARTESIAN_POINT('Ctrl Pts',(-7.6357544702348,0.103025538040317,-0.46775303145424));
#10446=CARTESIAN_POINT('Ctrl Pts',(-7.65117967263087,0.0513653977049828,
-0.464505680851719));
#10447=CARTESIAN_POINT('Ctrl Pts',(-7.65145417026957,-0.000143789196739241,
-0.461258330249198));
#10448=CARTESIAN_POINT('Origin',(-7.4,0.,-0.45));
#10449=CARTESIAN_POINT('',(-7.65214708790382,-1.47686313733716E-5,-0.361258330249198));
#10450=CARTESIAN_POINT('',(-7.65184733409926,0.000207924010478792,-0.388741669750802));
#10451=CARTESIAN_POINT('',(-7.65175,3.08304831685346E-17,-0.45));
#10452=CARTESIAN_POINT('Ctrl Pts',(-7.65184733409926,0.000207924010478792,
-0.388741669750802));
#10453=CARTESIAN_POINT('Ctrl Pts',(-7.65198960979724,0.0163122642644074,
-0.389761002795248));
#10454=CARTESIAN_POINT('Ctrl Pts',(-7.65057389537345,0.0323917047289323,
-0.390780335839695));
#10455=CARTESIAN_POINT('Ctrl Pts',(-7.64750824943319,0.0481501680948176,
-0.391799668884141));
#10456=CARTESIAN_POINT('Ctrl Pts',(-7.63176897737814,0.129055382499451,
-0.39703300646255));
#10457=CARTESIAN_POINT('Ctrl Pts',(-7.57253952466095,0.201500032408553,
-0.402266344040958));
#10458=CARTESIAN_POINT('Ctrl Pts',(-7.49637570051745,0.233003211517073,
-0.407499681619367));
#10459=CARTESIAN_POINT('Ctrl Pts',(-7.42021187637395,0.264506390625591,
-0.412733019197775));
#10460=CARTESIAN_POINT('Ctrl Pts',(-7.32711368080414,0.255068098933529,
-0.417966356776183));
#10461=CARTESIAN_POINT('Ctrl Pts',(-7.25882213636153,0.208920039824769,
-0.423199694354592));
#10462=CARTESIAN_POINT('Ctrl Pts',(-7.19053059191893,0.162771980716008,
-0.428433031933));
#10463=CARTESIAN_POINT('Ctrl Pts',(-7.14704569860354,0.0799141541905499,
-0.433666369511409));
#10464=CARTESIAN_POINT('Ctrl Pts',(-7.14786411692674,-0.00250373583704704,
-0.438899707089817));
#10465=CARTESIAN_POINT('Ctrl Pts',(-7.14868253524993,-0.0849216258646429,
-0.444133044668226));
#10466=CARTESIAN_POINT('Ctrl Pts',(-7.1938042652117,-0.166899579394378,
-0.449366382246634));
#10467=CARTESIAN_POINT('Ctrl Pts',(-7.26299876273194,-0.211682387612474,
-0.454599719825042));
#10468=CARTESIAN_POINT('Ctrl Pts',(-7.33219326025219,-0.256465195830571,
-0.459833057403451));
#10469=CARTESIAN_POINT('Ctrl Pts',(-7.4254605253309,-0.264052858737029,
-0.465066394981859));
#10470=CARTESIAN_POINT('Ctrl Pts',(-7.5009837323131,-0.231043411509504,
-0.470299732560268));
#10471=CARTESIAN_POINT('Ctrl Pts',(-7.57650693929529,-0.19803396428198,
-0.475533070138676));
#10472=CARTESIAN_POINT('Ctrl Pts',(-7.63428608818096,-0.124427406920472,
-0.480766407717085));
#10473=CARTESIAN_POINT('Ctrl Pts',(-7.64841562036082,-0.0432255920124892,
-0.485999745295493));
#10474=CARTESIAN_POINT('Ctrl Pts',(-7.65088326866655,-0.0290441231266644,
-0.48691372011393));
#10475=CARTESIAN_POINT('Ctrl Pts',(-7.65201956957008,-0.0146309929533726,
-0.487827694932366));
#10476=CARTESIAN_POINT('Ctrl Pts',(-7.65189502578968,-0.000198275244604145,
-0.488741669750802));
#10477=CARTESIAN_POINT('Ctrl Pts',(-7.65145417026957,-0.000143789196739241,
-0.461258330249198));
#10478=CARTESIAN_POINT('Ctrl Pts',(-7.6516220451935,-0.0316453382582933,
-0.459272343273311));
#10479=CARTESIAN_POINT('Ctrl Pts',(-7.64612325866364,-0.0630904277678157,
-0.457286356297423));
#10480=CARTESIAN_POINT('Ctrl Pts',(-7.63468587616665,-0.0922023870006976,
-0.455300369321535));
#10481=CARTESIAN_POINT('Ctrl Pts',(-7.60454686501157,-0.168916238644387,
-0.450067031743127));
#10482=CARTESIAN_POINT('Ctrl Pts',(-7.53317071863662,-0.229429020332177,
-0.444833694164719));
#10483=CARTESIAN_POINT('Ctrl Pts',(-7.45255927462588,-0.246609536103531,
-0.43960035658631));
#10484=CARTESIAN_POINT('Ctrl Pts',(-7.37194783061514,-0.263790051874886,
-0.434367019007902));
#10485=CARTESIAN_POINT('Ctrl Pts',(-7.28210108896861,-0.237638301729805,
-0.429133681429493));
#10486=CARTESIAN_POINT('Ctrl Pts',(-7.22330226728795,-0.179879548304771,
-0.423900343851085));
#10487=CARTESIAN_POINT('Ctrl Pts',(-7.16450344560729,-0.122120794879737,
-0.418667006272676));
#10488=CARTESIAN_POINT('Ctrl Pts',(-7.13675254389251,-0.0327550381747478,
-0.413433668694268));
#10489=CARTESIAN_POINT('Ctrl Pts',(-7.15249181203852,0.048150156136099,
-0.408200331115859));
#10490=CARTESIAN_POINT('Ctrl Pts',(-7.16823108018453,0.129055350446945,
-0.402966993537451));
#10491=CARTESIAN_POINT('Ctrl Pts',(-7.22746051819134,0.201499982363649,
-0.397733655959043));
#10492=CARTESIAN_POINT('Ctrl Pts',(-7.30362432341862,0.233003153647928,
-0.392500318380634));
#10493=CARTESIAN_POINT('Ctrl Pts',(-7.37978812864591,0.264506324932207,
-0.387266980802226));
#10494=CARTESIAN_POINT('Ctrl Pts',(-7.47288630109367,0.255068035584059,
-0.382033643223817));
#10495=CARTESIAN_POINT('Ctrl Pts',(-7.54117782857522,0.20891998793682,-0.376800305645408));
#10496=CARTESIAN_POINT('Ctrl Pts',(-7.60878192914431,0.163236469508371,
-0.371619647180005));
#10497=CARTESIAN_POINT('Ctrl Pts',(-7.65207628176844,0.0815785187217153,
-0.366438988714602));
#10498=CARTESIAN_POINT('Ctrl Pts',(-7.65214708790382,-1.47686313733716E-5,
-0.361258330249198));
#10499=CARTESIAN_POINT('Origin',(-7.4,0.,-0.45));
#10500=CARTESIAN_POINT('',(-7.65148582098249,0.000162483271353819,-0.261258330249198));
#10501=CARTESIAN_POINT('',(-7.65138929442701,-8.15071719056464E-5,-0.288741669750802));
#10502=CARTESIAN_POINT('',(-7.65175,3.08304831685346E-17,-0.45));
#10503=CARTESIAN_POINT('Ctrl Pts',(-7.65138929442701,-8.15071719056464E-5,
-0.288741669750802));
#10504=CARTESIAN_POINT('Ctrl Pts',(-7.65125007315824,0.0467834313418686,
-0.291694310658131));
#10505=CARTESIAN_POINT('Ctrl Pts',(-7.63865917700223,0.0937178577187305,
-0.29464695156546));
#10506=CARTESIAN_POINT('Ctrl Pts',(-7.61409346854159,0.133201947889911,
-0.297599592472789));
#10507=CARTESIAN_POINT('Ctrl Pts',(-7.57055256761178,0.203184576772822,
-0.302832930051198));
#10508=CARTESIAN_POINT('Ctrl Pts',(-7.48939286562526,0.249762019136108,
-0.308066267629606));
#10509=CARTESIAN_POINT('Ctrl Pts',(-7.40700270411694,0.252051055092709,
-0.313299605208014));
#10510=CARTESIAN_POINT('Ctrl Pts',(-7.32461254260861,0.254340091049311,
-0.318532942786423));
#10511=CARTESIAN_POINT('Ctrl Pts',(-7.2409919215785,0.212340720599228,-0.323766280364831));
#10512=CARTESIAN_POINT('Ctrl Pts',(-7.19363254765278,0.144883563035952,
-0.32899961794324));
#10513=CARTESIAN_POINT('Ctrl Pts',(-7.14627317372706,0.0774264054726766,
-0.334232955521648));
#10514=CARTESIAN_POINT('Ctrl Pts',(-7.13517504690573,-0.0154885392037914,
-0.339466293100057));
#10515=CARTESIAN_POINT('Ctrl Pts',(-7.16531406554617,-0.0922024099003809,
-0.344699630678465));
#10516=CARTESIAN_POINT('Ctrl Pts',(-7.1954530841866,-0.168916280596969,
-0.349932968256874));
#10517=CARTESIAN_POINT('Ctrl Pts',(-7.2668292482888,-0.22942907731368,-0.355166305835282));
#10518=CARTESIAN_POINT('Ctrl Pts',(-7.3474407123204,-0.246609597351995,
-0.36039964341369));
#10519=CARTESIAN_POINT('Ctrl Pts',(-7.42805217635201,-0.263790117390309,
-0.365632980992099));
#10520=CARTESIAN_POINT('Ctrl Pts',(-7.51789894031303,-0.237638360750227,
-0.370866318570507));
#10521=CARTESIAN_POINT('Ctrl Pts',(-7.57669777659709,-0.179879592980104,
-0.376099656148916));
#10522=CARTESIAN_POINT('Ctrl Pts',(-7.6240439603623,-0.133370896452756,
-0.380313660682878));
#10523=CARTESIAN_POINT('Ctrl Pts',(-7.65125915495639,-0.0663687098152037,
-0.38452766521684));
#10524=CARTESIAN_POINT('Ctrl Pts',(-7.65184733409926,0.000207924010478792,
-0.388741669750802));
#10525=CARTESIAN_POINT('Ctrl Pts',(-7.65214708790382,-1.47686313733716E-5,
-0.361258330249198));
#10526=CARTESIAN_POINT('Ctrl Pts',(-7.65214780789037,-0.000844443475530506,
-0.361205651136193));
#10527=CARTESIAN_POINT('Ctrl Pts',(-7.65214405870171,-0.00167411163369731,
-0.361152972023188));
#10528=CARTESIAN_POINT('Ctrl Pts',(-7.65213582045222,-0.00250373521502267,
-0.361100292910183));
#10529=CARTESIAN_POINT('Ctrl Pts',(-7.6513174023323,-0.0849216047732982,
-0.355866955331775));
#10530=CARTESIAN_POINT('Ctrl Pts',(-7.60619568357711,-0.166899537943519,
-0.350633617753367));
#10531=CARTESIAN_POINT('Ctrl Pts',(-7.53700120324214,-0.211682335038927,
-0.345400280174958));
#10532=CARTESIAN_POINT('Ctrl Pts',(-7.46780672290718,-0.256465132134335,
-0.34016694259655));
#10533=CARTESIAN_POINT('Ctrl Pts',(-7.37453948099245,-0.264052793154931,
-0.334933605018141));
#10534=CARTESIAN_POINT('Ctrl Pts',(-7.29901629276741,-0.231043354126343,
-0.329700267439733));
#10535=CARTESIAN_POINT('Ctrl Pts',(-7.22349310454237,-0.198033915097754,
-0.324466929861324));
#10536=CARTESIAN_POINT('Ctrl Pts',(-7.16571397000702,-0.12442737601998,
-0.319233592282916));
#10537=CARTESIAN_POINT('Ctrl Pts',(-7.15158444133632,-0.0432255812782405,
-0.314000254704507));
#10538=CARTESIAN_POINT('Ctrl Pts',(-7.13745491266562,0.0379762134634984,
-0.308766917126099));
#10539=CARTESIAN_POINT('Ctrl Pts',(-7.16697498985957,0.126773263869202,
-0.303533579547691));
#10540=CARTESIAN_POINT('Ctrl Pts',(-7.22690920460173,0.183352985471641,
-0.298300241969282));
#10541=CARTESIAN_POINT('Ctrl Pts',(-7.28684341934389,0.239932707074081,
-0.293066904390874));
#10542=CARTESIAN_POINT('Ctrl Pts',(-7.37719177163426,0.264295099873255,
-0.287833566812465));
#10543=CARTESIAN_POINT('Ctrl Pts',(-7.45744614455411,0.245517170168018,
-0.282600229234057));
#10544=CARTESIAN_POINT('Ctrl Pts',(-7.53770051747395,0.226739240462782,
-0.277366891655648));
#10545=CARTESIAN_POINT('Ctrl Pts',(-7.60786091102327,0.164820988253137,
-0.27213355407724));
#10546=CARTESIAN_POINT('Ctrl Pts',(-7.63647057578236,0.0875237549501118,
-0.266900216498831));
#10547=CARTESIAN_POINT('Ctrl Pts',(-7.64675161675558,0.0597465674368453,
-0.265019587748954));
#10548=CARTESIAN_POINT('Ctrl Pts',(-7.65166694660374,0.029983393820629,
-0.263138958999076));
#10549=CARTESIAN_POINT('Ctrl Pts',(-7.65148582098249,0.000162483271353819,
-0.261258330249198));
#10550=CARTESIAN_POINT('Origin',(-7.4,0.,-0.45));
#10551=CARTESIAN_POINT('',(-7.65166448275063,-0.000213511554003356,-0.161258330249198));
#10552=CARTESIAN_POINT('',(-7.65210261813639,-9.36994259479408E-5,-0.188741669750802));
#10553=CARTESIAN_POINT('',(-7.65175,3.08304831685346E-17,-0.45));
#10554=CARTESIAN_POINT('Ctrl Pts',(-7.65210261813639,-9.36994259479408E-5,
-0.188741669750802));
#10555=CARTESIAN_POINT('Ctrl Pts',(-7.65172967198033,0.0768944675440526,
-0.193627618521014));
#10556=CARTESIAN_POINT('Ctrl Pts',(-7.61382774165573,0.154200818874978,
-0.198513567291225));
#10557=CARTESIAN_POINT('Ctrl Pts',(-7.55255992854019,0.20075915469979,-0.203399516061437));
#10558=CARTESIAN_POINT('Ctrl Pts',(-7.48693600086431,0.250627767720387,
-0.208632853639845));
#10559=CARTESIAN_POINT('Ctrl Pts',(-7.39450546443956,0.265220588730429,
-0.213866191218254));
#10560=CARTESIAN_POINT('Ctrl Pts',(-7.31670998310708,0.23799484419977,-0.219099528796662));
#10561=CARTESIAN_POINT('Ctrl Pts',(-7.2389145017746,0.210769099669111,-0.224332866375071));
#10562=CARTESIAN_POINT('Ctrl Pts',(-7.17575407553438,0.141724789597751,
-0.229566203953479));
#10563=CARTESIAN_POINT('Ctrl Pts',(-7.15554698967948,0.0618182676595837,
-0.234799541531888));
#10564=CARTESIAN_POINT('Ctrl Pts',(-7.13533990382458,-0.0180882542785847,
-0.240032879110296));
#10565=CARTESIAN_POINT('Ctrl Pts',(-7.15808615835499,-0.108856988083561,
-0.245266216688704));
#10566=CARTESIAN_POINT('Ctrl Pts',(-7.21358735835509,-0.169791339561135,
-0.250499554267113));
#10567=CARTESIAN_POINT('Ctrl Pts',(-7.26908855835519,-0.230725691038708,
-0.255732891845522));
#10568=CARTESIAN_POINT('Ctrl Pts',(-7.35734470382498,-0.261825660188879,
-0.26096622942393));
#10569=CARTESIAN_POINT('Ctrl Pts',(-7.43878572988034,-0.249147425173802,
-0.266199567002338));
#10570=CARTESIAN_POINT('Ctrl Pts',(-7.5202267559357,-0.236469190158724,
-0.271432904580747));
#10571=CARTESIAN_POINT('Ctrl Pts',(-7.59485266257662,-0.180012750978398,
-0.276666242159155));
#10572=CARTESIAN_POINT('Ctrl Pts',(-7.62920456596055,-0.105090623686967,
-0.281899579737564));
#10573=CARTESIAN_POINT('Ctrl Pts',(-7.64417517898123,-0.0724394438722447,
-0.284180276408643));
#10574=CARTESIAN_POINT('Ctrl Pts',(-7.65149683255786,-0.0362812052094826,
-0.286460973079722));
#10575=CARTESIAN_POINT('Ctrl Pts',(-7.65138929442701,-8.15071719056464E-5,
-0.288741669750802));
#10576=CARTESIAN_POINT('Ctrl Pts',(-7.65148582098249,0.000162483271353819,
-0.261258330249198));
#10577=CARTESIAN_POINT('Ctrl Pts',(-7.65116291755486,-0.0530010292400235,
-0.257905621420667));
#10578=CARTESIAN_POINT('Ctrl Pts',(-7.63464229858077,-0.106348043093427,
-0.254552912592137));
#10579=CARTESIAN_POINT('Ctrl Pts',(-7.60344957268528,-0.148953054949818,
-0.251200203763606));
#10580=CARTESIAN_POINT('Ctrl Pts',(-7.55475996886024,-0.215456417150318,
-0.245966866185197));
#10581=CARTESIAN_POINT('Ctrl Pts',(-7.47032182524129,-0.255786927154911,
-0.240733528606789));
#10582=CARTESIAN_POINT('Ctrl Pts',(-7.38799338681216,-0.251862223513114,
-0.235500191028381));
#10583=CARTESIAN_POINT('Ctrl Pts',(-7.30566494838303,-0.247937519871316,
-0.230266853449972));
#10584=CARTESIAN_POINT('Ctrl Pts',(-7.22544621514372,-0.199757602583128,
-0.225033515871564));
#10585=CARTESIAN_POINT('Ctrl Pts',(-7.18330364444125,-0.128924136071955,
-0.219800178293155));
#10586=CARTESIAN_POINT('Ctrl Pts',(-7.14116107373879,-0.0580906695607829,
-0.214566840714747));
#10587=CARTESIAN_POINT('Ctrl Pts',(-7.13709466557317,0.0353963461733736,
-0.209333503136338));
#10588=CARTESIAN_POINT('Ctrl Pts',(-7.17292760647834,0.109621493446434,
-0.20410016555793));
#10589=CARTESIAN_POINT('Ctrl Pts',(-7.20876054738351,0.183846640719495,
-0.198866827979521));
#10590=CARTESIAN_POINT('Ctrl Pts',(-7.28449283735947,0.23880991953146,-0.193633490401113));
#10591=CARTESIAN_POINT('Ctrl Pts',(-7.36616955518689,0.249868412754667,
-0.188400152822705));
#10592=CARTESIAN_POINT('Ctrl Pts',(-7.44784627301432,0.260926905977874,
-0.183166815244296));
#10593=CARTESIAN_POINT('Ctrl Pts',(-7.53546741869321,0.228080613612323,
-0.177933477665888));
#10594=CARTESIAN_POINT('Ctrl Pts',(-7.58974760249707,0.166056061051272,
-0.172700140087479));
#10595=CARTESIAN_POINT('Ctrl Pts',(-7.62930575773839,0.120853987162775,
-0.168886203474719));
#10596=CARTESIAN_POINT('Ctrl Pts',(-7.65115599235281,0.0601548704022266,
-0.165072266861958));
#10597=CARTESIAN_POINT('Ctrl Pts',(-7.65166448275063,-0.000213511554003356,
-0.161258330249198));
#10598=CARTESIAN_POINT('Origin',(-7.4,0.,-0.45));
#10599=CARTESIAN_POINT('',(-7.65205352925247,0.000126382978640343,-0.0612583302491982));
#10600=CARTESIAN_POINT('',(-7.65159361924534,0.000201202514259572,-0.0887416697508019));
#10601=CARTESIAN_POINT('',(-7.65175,3.08304831685346E-17,-0.45));
#10602=CARTESIAN_POINT('',(-7.20865340033349,0.163598720337495,0.));
#10603=CARTESIAN_POINT('Ctrl Pts',(-7.65205352925247,0.000126382978640343,
-0.0612583302491982));
#10604=CARTESIAN_POINT('Ctrl Pts',(-7.65157449481833,-0.0742619827859457,
-0.0565388995680243));
#10605=CARTESIAN_POINT('Ctrl Pts',(-7.61652851723279,-0.14902715398977,
-0.0518194688868503));
#10606=CARTESIAN_POINT('Ctrl Pts',(-7.55878735064402,-0.195852509824499,
-0.0471000382056764));
#10607=CARTESIAN_POINT('Ctrl Pts',(-7.49475864944166,-0.247776758927207,
-0.0418667006272679));
#10608=CARTESIAN_POINT('Ctrl Pts',(-7.40282301710629,-0.26534507015853,
-0.0366333630488594));
#10609=CARTESIAN_POINT('Ctrl Pts',(-7.3242152913777,-0.240530493415837,
-0.0314000254704509));
#10610=CARTESIAN_POINT('Ctrl Pts',(-7.24560756564911,-0.215715916673145,
-0.0261666878920424));
#10611=CARTESIAN_POINT('Ctrl Pts',(-7.18032774652728,-0.148518451956437,
-0.020933350313634));
#10612=CARTESIAN_POINT('Ctrl Pts',(-7.15764056021304,-0.0694194541751962,
-0.0157000127352255));
#10613=CARTESIAN_POINT('Ctrl Pts',(-7.1349533738988,0.00967954360604439,
-0.010466675156817));
#10614=CARTESIAN_POINT('Ctrl Pts',(-7.15485882039215,0.100680074451818,
-0.00523333757840849));
#10615=CARTESIAN_POINT('Ctrl Pts',(-7.20865340033349,0.163598720337495,
0.));
#10616=CARTESIAN_POINT('',(-7.59170239456967,0.163827044623994,1.51684295230343E-16));
#10617=CARTESIAN_POINT('Origin',(-7.4,0.,0.));
#10618=CARTESIAN_POINT('Ctrl Pts',(-7.59170406260212,0.163828115050569,
9.71445146547012E-17));
#10619=CARTESIAN_POINT('Ctrl Pts',(-7.54033259098557,0.223538299415699,
-0.00499978774624421));
#10620=CARTESIAN_POINT('Ctrl Pts',(-7.45859288812061,0.257577547385412,
-0.00999957549248855));
#10621=CARTESIAN_POINT('Ctrl Pts',(-7.3800820254476,0.251346298664483,-0.0149993632387328));
#10622=CARTESIAN_POINT('Ctrl Pts',(-7.29790376733084,0.244823976168664,
-0.0202327008171413));
#10623=CARTESIAN_POINT('Ctrl Pts',(-7.21926304559467,0.19418105970145,-0.0254660383955497));
#10624=CARTESIAN_POINT('Ctrl Pts',(-7.17937085476038,0.122067692519252,
-0.0306993759739582));
#10625=CARTESIAN_POINT('Ctrl Pts',(-7.13947866392609,0.0499543253370541,
-0.0359327135523666));
#10626=CARTESIAN_POINT('Ctrl Pts',(-7.13833500399368,-0.0436294925601266,
-0.0411660511307751));
#10627=CARTESIAN_POINT('Ctrl Pts',(-7.17647638632986,-0.116697424671654,
-0.0463993887091836));
#10628=CARTESIAN_POINT('Ctrl Pts',(-7.21461776866604,-0.189765356783182,
-0.051632726287592));
#10629=CARTESIAN_POINT('Ctrl Pts',(-7.29204419327081,-0.242317403109057,
-0.0568660638660004));
#10630=CARTESIAN_POINT('Ctrl Pts',(-7.37402938284013,-0.25080526728572,
-0.0620994014444088));
#10631=CARTESIAN_POINT('Ctrl Pts',(-7.45601457240945,-0.259293131462382,
-0.0673327390228173));
#10632=CARTESIAN_POINT('Ctrl Pts',(-7.54255852694332,-0.223716813489832,
-0.0725660766012258));
#10633=CARTESIAN_POINT('Ctrl Pts',(-7.59486468239543,-0.160020353024002,
-0.0777994141796342));
#10634=CARTESIAN_POINT('Ctrl Pts',(-7.63131989619396,-0.11562657060164,
-0.0814468327033568));
#10635=CARTESIAN_POINT('Ctrl Pts',(-7.65114406502439,-0.0575734009856725,
-0.0850942512270794));
#10636=CARTESIAN_POINT('Ctrl Pts',(-7.65159361924534,0.000201202514259572,
-0.0887416697508019));
#10637=CARTESIAN_POINT('Origin',(0.,7.4,0.220842344717745));
#10638=CARTESIAN_POINT('',(-0.307744900822632,7.40014697529577,-0.720842344717746));
#10639=CARTESIAN_POINT('',(-0.306871987992451,7.39998793159208,-0.729157655282255));
#10640=CARTESIAN_POINT('',(-0.30735,7.40000000000001,0.220842344717745));
#10641=CARTESIAN_POINT('',(0.0793799282532798,7.10307770462543,-0.8));
#10642=CARTESIAN_POINT('Ctrl Pts',(-0.306871987992451,7.39998793159208,
-0.729157655282255));
#10643=CARTESIAN_POINT('Ctrl Pts',(-0.306838385861804,7.45195236281704,
-0.731838419874536));
#10644=CARTESIAN_POINT('Ctrl Pts',(-0.269833682477504,7.60539570033716,
-0.739752522045226));
#10645=CARTESIAN_POINT('Ctrl Pts',(-0.0286357467853838,7.76072171687769,
-0.752899961794324));
#10646=CARTESIAN_POINT('Ctrl Pts',(0.285303569958047,7.62301619686966,-0.76859997452955));
#10647=CARTESIAN_POINT('Ctrl Pts',(0.342929470763259,7.28476159359493,-0.784299987264775));
#10648=CARTESIAN_POINT('Ctrl Pts',(0.177014005842301,7.12917943627315,-0.794766662421592));
#10649=CARTESIAN_POINT('Ctrl Pts',(0.0793799282532802,7.10307770462543,
-0.8));
#10650=CARTESIAN_POINT('',(-0.0795800004915529,7.10260193843563,-0.8));
#10651=CARTESIAN_POINT('Origin',(0.,7.4,-0.8));
#10652=CARTESIAN_POINT('Ctrl Pts',(-0.307744900822632,7.40014697529577,
-0.720842344717746));
#10653=CARTESIAN_POINT('Ctrl Pts',(-0.307796455021018,7.40885909073305,
-0.721295091751952));
#10654=CARTESIAN_POINT('Ctrl Pts',(-0.303543375023605,7.51822382240117,
-0.726981176364568));
#10655=CARTESIAN_POINT('Ctrl Pts',(-0.173198863217152,7.71778292610997,
-0.73790059855559));
#10656=CARTESIAN_POINT('Ctrl Pts',(0.169525116851479,7.71979476003134,-0.753600611290817));
#10657=CARTESIAN_POINT('Ctrl Pts',(0.360224711692468,7.43495575882791,-0.769300624026041));
#10658=CARTESIAN_POINT('Ctrl Pts',(0.229894698648723,7.12364967101413,-0.784767086929103));
#10659=CARTESIAN_POINT('Ctrl Pts',(0.0133964428701133,7.07805035355335,
-0.795000212253756));
#10660=CARTESIAN_POINT('Ctrl Pts',(-0.0795809384672905,7.10259970795555,
-0.8));
#10661=CARTESIAN_POINT('Origin',(0.,7.4,0.220842344717745));
#10662=CARTESIAN_POINT('',(-0.306892537291858,7.40006920001046,-0.620842344717746));
#10663=CARTESIAN_POINT('',(-0.307676148864859,7.39981196746108,-0.629157655282254));
#10664=CARTESIAN_POINT('',(-0.30735,7.40000000000001,0.220842344717745));
#10665=CARTESIAN_POINT('Ctrl Pts',(-0.307676148864859,7.39981196746108,
-0.629157655282254));
#10666=CARTESIAN_POINT('Ctrl Pts',(-0.307031426701065,7.48865284062119,
-0.633771727737418));
#10667=CARTESIAN_POINT('Ctrl Pts',(-0.220226223500933,7.67935845555228,
-0.643619137770991));
#10668=CARTESIAN_POINT('Ctrl Pts',(0.101895231555572,7.74728571705174,-0.658699885382972));
#10669=CARTESIAN_POINT('Ctrl Pts',(0.345877106706635,7.50659191670458,-0.674399898118198));
#10670=CARTESIAN_POINT('Ctrl Pts',(0.279700633697489,7.17030794277179,-0.690099910853422));
#10671=CARTESIAN_POINT('Ctrl Pts',(-0.0372719056216933,7.04000753659561,
-0.705799923588649));
#10672=CARTESIAN_POINT('Ctrl Pts',(-0.27243006304546,7.19961759943849,-0.718819171731592));
#10673=CARTESIAN_POINT('Ctrl Pts',(-0.306903983301257,7.35050838990976,
-0.726605082296127));
#10674=CARTESIAN_POINT('Ctrl Pts',(-0.306871987992451,7.39998793159208,
-0.729157655282255));
#10675=CARTESIAN_POINT('Ctrl Pts',(-0.306892537291858,7.40006920001046,
-0.620842344717746));
#10676=CARTESIAN_POINT('Ctrl Pts',(-0.306987708470476,7.44631180509704,
-0.623228399614835));
#10677=CARTESIAN_POINT('Ctrl Pts',(-0.275630272390186,7.59385583250629,
-0.630847792090333));
#10678=CARTESIAN_POINT('Ctrl Pts',(-0.0485593254958618,7.75865428087583,
-0.643700522144239));
#10679=CARTESIAN_POINT('Ctrl Pts',(0.27235863905538,7.63835266345873,-0.659400534879465));
#10680=CARTESIAN_POINT('Ctrl Pts',(0.349049856868627,7.30431662403272,-0.67510054761469));
#10681=CARTESIAN_POINT('Ctrl Pts',(0.112745006295209,7.05608341261925,-0.690800560349915));
#10682=CARTESIAN_POINT('Ctrl Pts',(-0.214930081152626,7.11450349903993,
-0.706047826050933));
#10683=CARTESIAN_POINT('Ctrl Pts',(-0.307200536100844,7.30815508240031,
-0.716061754173544));
#10684=CARTESIAN_POINT('Ctrl Pts',(-0.307744900822632,7.40014697529577,
-0.720842344717746));
#10685=CARTESIAN_POINT('Origin',(0.,7.4,0.220842344717745));
#10686=CARTESIAN_POINT('',(-0.307527055318605,7.3997579348702,-0.520842344717746));
#10687=CARTESIAN_POINT('',(-0.307303201782415,7.40026451811874,-0.529157655282254));
#10688=CARTESIAN_POINT('',(-0.30735,7.40000000000001,0.220842344717745));
#10689=CARTESIAN_POINT('Ctrl Pts',(-0.307303201782415,7.40026451811874,
-0.529157655282254));
#10690=CARTESIAN_POINT('Ctrl Pts',(-0.307524010692625,7.42564508780896,
-0.530471698021893));
#10691=CARTESIAN_POINT('Ctrl Pts',(-0.293133012622773,7.55186005371301,
-0.537019078339939));
#10692=CARTESIAN_POINT('Ctrl Pts',(-0.119552197626099,7.74161126864207,
-0.548799796236395));
#10693=CARTESIAN_POINT('Ctrl Pts',(0.21898032116491,7.68816416491483,-0.56449980897162));
#10694=CARTESIAN_POINT('Ctrl Pts',(0.361151136941273,7.37631755024098,-0.580199821706846));
#10695=CARTESIAN_POINT('Ctrl Pts',(0.17947415907044,7.08570709394078,-0.59589983444207));
#10696=CARTESIAN_POINT('Ctrl Pts',(-0.163138808425949,7.0769263467909,-0.611599847177296));
#10697=CARTESIAN_POINT('Ctrl Pts',(-0.301766089733603,7.27528825889535,
-0.622685787457357));
#10698=CARTESIAN_POINT('Ctrl Pts',(-0.307762678487899,7.38788843249251,
-0.62853839015901));
#10699=CARTESIAN_POINT('Ctrl Pts',(-0.307676148864859,7.39981196746108,
-0.629157655282254));
#10700=CARTESIAN_POINT('Ctrl Pts',(-0.307527055318605,7.3997579348702,-0.520842344717746));
#10701=CARTESIAN_POINT('Ctrl Pts',(-0.306808481761244,7.48302961068977,
-0.525161707477718));
#10702=CARTESIAN_POINT('Ctrl Pts',(-0.229186183907421,7.66837439690706,
-0.534714407816098));
#10703=CARTESIAN_POINT('Ctrl Pts',(0.0824566524067525,7.75240874841395,
-0.549500445732887));
#10704=CARTESIAN_POINT('Ctrl Pts',(0.339423512150486,7.52562925031437,-0.565200458468112));
#10705=CARTESIAN_POINT('Ctrl Pts',(0.292026050158285,7.1861967789166,-0.580900471203337));
#10706=CARTESIAN_POINT('Ctrl Pts',(-0.0172339683272763,7.03848374595487,
-0.596600483938563));
#10707=CARTESIAN_POINT('Ctrl Pts',(-0.26638808838325,7.18812740699665,-0.609914441776699));
#10708=CARTESIAN_POINT('Ctrl Pts',(-0.30677896938989,7.34488783399801,-0.617995062036427));
#10709=CARTESIAN_POINT('Ctrl Pts',(-0.306892537291858,7.40006920001046,
-0.620842344717746));
#10710=CARTESIAN_POINT('Origin',(0.,7.4,0.220842344717745));
#10711=CARTESIAN_POINT('',(-0.307468830726541,7.40025384486444,-0.420842344717745));
#10712=CARTESIAN_POINT('',(-0.306988859154633,7.39982445436712,-0.429157655282254));
#10713=CARTESIAN_POINT('',(-0.30735,7.40000000000001,0.220842344717745));
#10714=CARTESIAN_POINT('Ctrl Pts',(-0.306988859154633,7.39982445436712,
-0.429157655282254));
#10715=CARTESIAN_POINT('Ctrl Pts',(-0.306653737582139,7.462709657289,-0.432405005884775));
#10716=CARTESIAN_POINT('Ctrl Pts',(-0.257472827761211,7.62742015105949,
-0.440885694065705));
#10717=CARTESIAN_POINT('Ctrl Pts',(0.0100514892332193,7.76178716191776,
-0.454599719825043));
#10718=CARTESIAN_POINT('Ctrl Pts',(0.307303884459003,7.59119441739787,-0.470299732560268));
#10719=CARTESIAN_POINT('Ctrl Pts',(0.328993939119635,7.24915580545685,-0.485999745295493));
#10720=CARTESIAN_POINT('Ctrl Pts',(0.0556719707952805,7.04238062809055,
-0.501699758030718));
#10721=CARTESIAN_POINT('Ctrl Pts',(-0.240517094087265,7.14675263225517,
-0.516085728026306));
#10722=CARTESIAN_POINT('Ctrl Pts',(-0.30664461192378,7.32456383290414,-0.525238360443484));
#10723=CARTESIAN_POINT('Ctrl Pts',(-0.307303201782415,7.40026451811874,
-0.529157655282254));
#10724=CARTESIAN_POINT('Ctrl Pts',(-0.307468830726541,7.40025384486444,
-0.420842344717745));
#10725=CARTESIAN_POINT('Ctrl Pts',(-0.307642528584636,7.41991489343264,
-0.421861677762192));
#10726=CARTESIAN_POINT('Ctrl Pts',(-0.297040503111005,7.54033087178353,
-0.428114348385046));
#10727=CARTESIAN_POINT('Ctrl Pts',(-0.138335057048331,7.73444646717113,
-0.43960035658631));
#10728=CARTESIAN_POINT('Ctrl Pts',(0.202642862416027,7.69987813805627,-0.455300369321535));
#10729=CARTESIAN_POINT('Ctrl Pts',(0.361908983097054,7.39640620579093,-0.47100038205676));
#10730=CARTESIAN_POINT('Ctrl Pts',(0.196647846607491,7.09615686298222,-0.486700394791986));
#10731=CARTESIAN_POINT('Ctrl Pts',(-0.144949300426615,7.06836657665492,
-0.502400407527211));
#10732=CARTESIAN_POINT('Ctrl Pts',(-0.298348535773798,7.26378637486166,
-0.513781057502464));
#10733=CARTESIAN_POINT('Ctrl Pts',(-0.307679105093796,7.38213769340927,
-0.519928369899309));
#10734=CARTESIAN_POINT('Ctrl Pts',(-0.307527055318605,7.3997579348702,-0.520842344717746));
#10735=CARTESIAN_POINT('Origin',(0.,7.4,0.220842344717745));
#10736=CARTESIAN_POINT('',(-0.306909631150515,7.39990049164138,-0.320842344717745));
#10737=CARTESIAN_POINT('',(-0.307834810501565,7.3999819696555,-0.329157655282254));
#10738=CARTESIAN_POINT('',(-0.30735,7.40000000000001,0.220842344717745));
#10739=CARTESIAN_POINT('Ctrl Pts',(-0.307834810501565,7.3999819696555,-0.329157655282254));
#10740=CARTESIAN_POINT('Ctrl Pts',(-0.307748366539647,7.49959547048682,
-0.334338313747658));
#10741=CARTESIAN_POINT('Ctrl Pts',(-0.201498726273864,7.69999407607993,
-0.34475230979147));
#10742=CARTESIAN_POINT('Ctrl Pts',(0.138335033537924,7.73444641033119,-0.36039964341369));
#10743=CARTESIAN_POINT('Ctrl Pts',(0.355266543354486,7.46911342881649,-0.376099656148916));
#10744=CARTESIAN_POINT('Ctrl Pts',(0.25362713547982,7.1418057726863,-0.391799668884141));
#10745=CARTESIAN_POINT('Ctrl Pts',(-0.0754421579893288,7.0460233571473,
-0.407499681619367));
#10746=CARTESIAN_POINT('Ctrl Pts',(-0.282790383856574,7.22181342935611,
-0.419952343752071));
#10747=CARTESIAN_POINT('Ctrl Pts',(-0.307193809946764,7.36136565848536,
-0.427171668306367));
#10748=CARTESIAN_POINT('Ctrl Pts',(-0.306988859154633,7.39982445436712,
-0.429157655282254));
#10749=CARTESIAN_POINT('Ctrl Pts',(-0.306909631150515,7.39990049164138,
-0.320842344717745));
#10750=CARTESIAN_POINT('Ctrl Pts',(-0.306739662304611,7.45711574030953,
-0.323794985625074));
#10751=CARTESIAN_POINT('Ctrl Pts',(-0.264122910345685,7.61597598206296,
-0.331980964110812));
#10752=CARTESIAN_POINT('Ctrl Pts',(-0.0100514909408711,7.76178722340353,
-0.345400280174958));
#10753=CARTESIAN_POINT('Ctrl Pts',(0.296214223541038,7.60796192241644,-0.361100292910183));
#10754=CARTESIAN_POINT('Ctrl Pts',(0.336861801835373,7.26765517072256,-0.376800305645408));
#10755=CARTESIAN_POINT('Ctrl Pts',(0.0754421708108413,7.04602329698811,
-0.392500318380633));
#10756=CARTESIAN_POINT('Ctrl Pts',(-0.232262147395604,7.13558699513454,
-0.407180998071413));
#10757=CARTESIAN_POINT('Ctrl Pts',(-0.30675074985441,7.31897349369731,-0.416628340183783));
#10758=CARTESIAN_POINT('Ctrl Pts',(-0.307468830726541,7.40025384486444,
-0.420842344717745));
#10759=CARTESIAN_POINT('Origin',(0.,7.4,0.220842344717745));
#10760=CARTESIAN_POINT('',(-0.307780495269994,7.39988560667899,-0.220842344717745));
#10761=CARTESIAN_POINT('',(-0.307027500057518,7.40019836837334,-0.229157655282254));
#10762=CARTESIAN_POINT('',(-0.30735,7.40000000000001,0.220842344717745));
#10763=CARTESIAN_POINT('Ctrl Pts',(-0.307027500057518,7.40019836837334,
-0.229157655282254));
#10764=CARTESIAN_POINT('Ctrl Pts',(-0.307248628018252,7.43660534980473,
-0.231038284032132));
#10765=CARTESIAN_POINT('Ctrl Pts',(-0.284548663759526,7.57405756525429,
-0.238152250360418));
#10766=CARTESIAN_POINT('Ctrl Pts',(-0.0824566383942325,7.75240868850505,
-0.250499554267113));
#10767=CARTESIAN_POINT('Ctrl Pts',(0.248449835333973,7.66317990580525,-0.266199567002338));
#10768=CARTESIAN_POINT('Ctrl Pts',(0.356568958714344,7.3379551719626,-0.281899579737564));
#10769=CARTESIAN_POINT('Ctrl Pts',(0.144949275792185,7.0683666330192,-0.297599592472788));
#10770=CARTESIAN_POINT('Ctrl Pts',(-0.196647813186698,7.09615691462004,
-0.313299605208015));
#10771=CARTESIAN_POINT('Ctrl Pts',(-0.30737639510771,7.29733055204229,-0.323818959477836));
#10772=CARTESIAN_POINT('Ctrl Pts',(-0.307835689500107,7.39896905770576,
-0.329104976169249));
#10773=CARTESIAN_POINT('Ctrl Pts',(-0.307834810501565,7.3999819696555,-0.329157655282254));
#10774=CARTESIAN_POINT('Ctrl Pts',(-0.307780495269994,7.39988560667899,
-0.220842344717745));
#10775=CARTESIAN_POINT('Ctrl Pts',(-0.307325182455431,7.49387691995895,
-0.225728293487957));
#10776=CARTESIAN_POINT('Ctrl Pts',(-0.211489763984475,7.68934681995645,
-0.235847579836577));
#10777=CARTESIAN_POINT('Ctrl Pts',(0.119552217972776,7.7416113266484,-0.251200203763606));
#10778=CARTESIAN_POINT('Ctrl Pts',(0.350881199163606,7.48873225573956,-0.266900216498831));
#10779=CARTESIAN_POINT('Ctrl Pts',(0.267571630187383,7.15628613456826,-0.282600229234056));
#10780=CARTESIAN_POINT('Ctrl Pts',(-0.0556719802611724,7.04238056731933,
-0.298300241969282));
#10781=CARTESIAN_POINT('Ctrl Pts',(-0.277591376746854,7.21026836224977,
-0.311047613797178));
#10782=CARTESIAN_POINT('Ctrl Pts',(-0.307040919510058,7.35570594470255,
-0.318561648046666));
#10783=CARTESIAN_POINT('Ctrl Pts',(-0.306909631150515,7.39990049164138,
-0.320842344717745));
#10784=CARTESIAN_POINT('Origin',(0.,7.4,0.220842344717745));
#10785=CARTESIAN_POINT('',(-0.307159081926734,7.40024563889874,-0.120842344717745));
#10786=CARTESIAN_POINT('',(-0.307245619935592,7.39973933390828,-0.129157655282254));
#10787=CARTESIAN_POINT('',(-0.30735,7.40000000000001,0.220842344717745));
#10788=CARTESIAN_POINT('Ctrl Pts',(-0.307245619935592,7.39973933390828,
-0.129157655282254));
#10789=CARTESIAN_POINT('Ctrl Pts',(-0.306624827350326,7.47344032150659,
-0.132971591895015));
#10790=CARTESIAN_POINT('Ctrl Pts',(-0.243345164403822,7.64922880659321,
-0.142018866086184));
#10791=CARTESIAN_POINT('Ctrl Pts',(0.0485593171240025,7.7586542191763,-0.156299477855761));
#10792=CARTESIAN_POINT('Ctrl Pts',(0.325933551193656,7.55734778288709,-0.171999490590986));
#10793=CARTESIAN_POINT('Ctrl Pts',(0.311040077773849,7.21494575887322,-0.187699503326212));
#10794=CARTESIAN_POINT('Ctrl Pts',(0.0172339654105937,7.03848380750682,
-0.203399516061437));
#10795=CARTESIAN_POINT('Ctrl Pts',(-0.254981241847562,7.16850298693634,
-0.217218900046784));
#10796=CARTESIAN_POINT('Ctrl Pts',(-0.306633282077901,7.33529347522358,
-0.225804946453723));
#10797=CARTESIAN_POINT('Ctrl Pts',(-0.307027500057518,7.40019836837334,
-0.229157655282254));
#10798=CARTESIAN_POINT('Ctrl Pts',(-0.307159081926734,7.40024563889874,
-0.120842344717745));
#10799=CARTESIAN_POINT('Ctrl Pts',(-0.307397720825203,7.43091439273595,
-0.122428263772431));
#10800=CARTESIAN_POINT('Ctrl Pts',(-0.28919541585723,7.56250979326726,-0.129247520405525));
#10801=CARTESIAN_POINT('Ctrl Pts',(-0.101895250628719,7.74728578061798,
-0.141300114617028));
#10802=CARTESIAN_POINT('Ctrl Pts',(0.233453631148172,7.67656918324398,-0.157000127352253));
#10803=CARTESIAN_POINT('Ctrl Pts',(0.359464126606772,7.35784834370038,-0.172700140087479));
#10804=CARTESIAN_POINT('Ctrl Pts',(0.163138836475842,7.07692629120202,-0.188400152822704));
#10805=CARTESIAN_POINT('Ctrl Pts',(-0.179474189751402,7.08570704088486,
-0.20410016555793));
#10806=CARTESIAN_POINT('Ctrl Pts',(-0.304612100383046,7.28587761682761,
-0.214914229522943));
#10807=CARTESIAN_POINT('Ctrl Pts',(-0.307812867810814,7.39320286565227,
-0.220494955909548));
#10808=CARTESIAN_POINT('Ctrl Pts',(-0.307780495269994,7.39988560667899,
-0.220842344717745));
#10809=CARTESIAN_POINT('Origin',(0.,7.4,0.220842344717745));
#10810=CARTESIAN_POINT('',(-0.30701976654778,7.39969382919393,-0.0208423447177451));
#10811=CARTESIAN_POINT('',(-0.307720586104713,7.40015430359934,-0.0291576552822542));
#10812=CARTESIAN_POINT('',(-0.30735,7.40000000000001,0.220842344717745));
#10813=CARTESIAN_POINT('',(-0.0793799282532889,7.10307770462543,0.));
#10814=CARTESIAN_POINT('Ctrl Pts',(-0.0793799282532879,7.10307770462543,
5.55111512312578E-17));
#10815=CARTESIAN_POINT('Ctrl Pts',(-0.177014005842308,7.12917943627315,
-0.00523333757840839));
#10816=CARTESIAN_POINT('Ctrl Pts',(-0.287143377782575,7.23245041729098,
-0.0121807858176568));
#10817=CARTESIAN_POINT('Ctrl Pts',(-0.307246205355195,7.36652716202022,
-0.0191282340569052));
#10818=CARTESIAN_POINT('Ctrl Pts',(-0.30701976654778,7.39969382919393,-0.0208423447177451));
#10819=CARTESIAN_POINT('',(0.0795799507667233,7.10260193953608,6.20619955657751E-17));
#10820=CARTESIAN_POINT('Origin',(0.,7.4,0.));
#10821=CARTESIAN_POINT('Ctrl Pts',(0.0795808873001328,7.10259971193733,
-3.33392168039293E-18));
#10822=CARTESIAN_POINT('Ctrl Pts',(-0.0133965346091573,7.07805031897846,
-0.00499978774624427));
#10823=CARTESIAN_POINT('Ctrl Pts',(-0.219022047825184,7.12135984424409,
-0.0147190061736623));
#10824=CARTESIAN_POINT('Ctrl Pts',(-0.307135762589409,7.30933695078315,
-0.0244382246010804));
#10825=CARTESIAN_POINT('Ctrl Pts',(-0.307720586104713,7.40015430359934,
-0.0291576552822542));
#10826=CARTESIAN_POINT('Origin',(7.4,0.,0.220842344717745));
#10827=CARTESIAN_POINT('',(7.09225513659108,0.000146978884224908,-0.720842344717746));
#10828=CARTESIAN_POINT('',(7.0931279909255,-1.20749723882283E-5,-0.729157655282255));
#10829=CARTESIAN_POINT('',(7.09265,5.61065397787037E-15,0.220842344717745));
#10830=CARTESIAN_POINT('',(7.47937992825329,-0.29692229537457,-0.8));
#10831=CARTESIAN_POINT('Ctrl Pts',(7.0931279909255,-1.20749723881847E-5,
-0.729157655282255));
#10832=CARTESIAN_POINT('Ctrl Pts',(7.09316159233691,0.0519523551408496,
-0.731838419874536));
#10833=CARTESIAN_POINT('Ctrl Pts',(7.13016629582236,0.205395693670095,-0.739752522045226));
#10834=CARTESIAN_POINT('Ctrl Pts',(7.37136424992534,0.360721809373367,-0.752899961794324));
#10835=CARTESIAN_POINT('Ctrl Pts',(7.68530360759964,0.223016092822843,-0.768599974529549));
#10836=CARTESIAN_POINT('Ctrl Pts',(7.74292942723977,-0.115238123859802,
-0.784299987264775));
#10837=CARTESIAN_POINT('Ctrl Pts',(7.57701400584231,-0.270820563726849,
-0.794766662421592));
#10838=CARTESIAN_POINT('Ctrl Pts',(7.47937992825329,-0.29692229537457,-0.8));
#10839=CARTESIAN_POINT('',(7.32042003604622,-0.297398060701823,-0.799999999999999));
#10840=CARTESIAN_POINT('Origin',(7.4,0.,-0.8));
#10841=CARTESIAN_POINT('Ctrl Pts',(7.09225513659108,0.000146978884224968,
-0.720842344717746));
#10842=CARTESIAN_POINT('Ctrl Pts',(7.09220358244584,0.00885909314624902,
-0.721295091751953));
#10843=CARTESIAN_POINT('Ctrl Pts',(7.09645666272727,0.118223809389764,-0.726981176364568));
#10844=CARTESIAN_POINT('Ctrl Pts',(7.22680116614257,0.317782866086405,-0.737900598555591));
#10845=CARTESIAN_POINT('Ctrl Pts',(7.56952507950631,0.319794755380677,-0.753600611290817));
#10846=CARTESIAN_POINT('Ctrl Pts',(7.76022470046591,0.0349556943853752,
-0.769300624026041));
#10847=CARTESIAN_POINT('Ctrl Pts',(7.62989460038476,-0.276350197541752,
-0.784767086929103));
#10848=CARTESIAN_POINT('Ctrl Pts',(7.41339651031425,-0.321949671834906,
-0.795000212253756));
#10849=CARTESIAN_POINT('Ctrl Pts',(7.32041909912987,-0.297400289065614,
-0.8));
#10850=CARTESIAN_POINT('Origin',(7.4,0.,0.220842344717745));
#10851=CARTESIAN_POINT('',(7.09310750107417,6.92000663027048E-5,-0.620842344717746));
#10852=CARTESIAN_POINT('',(7.09232382992685,-0.000188032469277442,-0.629157655282255));
#10853=CARTESIAN_POINT('',(7.09265,5.61065397787037E-15,0.220842344717745));
#10854=CARTESIAN_POINT('Ctrl Pts',(7.09232382992685,-0.000188032469277427,
-0.629157655282255));
#10855=CARTESIAN_POINT('Ctrl Pts',(7.09296855206387,0.088652846655831,-0.633771727737419));
#10856=CARTESIAN_POINT('Ctrl Pts',(7.17977376091732,0.279358473971188,-0.643619137770991));
#10857=CARTESIAN_POINT('Ctrl Pts',(7.50189523930833,0.347285742890038,-0.658699885382972));
#10858=CARTESIAN_POINT('Ctrl Pts',(7.74587712940208,0.10659192062098,-0.674399898118197));
#10859=CARTESIAN_POINT('Ctrl Pts',(7.67970065492672,-0.229692066723022,
-0.690099910853423));
#10860=CARTESIAN_POINT('Ctrl Pts',(7.36272808895739,-0.359992499947249,
-0.705799923588647));
#10861=CARTESIAN_POINT('Ctrl Pts',(7.1275699207301,-0.200382398818872,-0.718819171731592));
#10862=CARTESIAN_POINT('Ctrl Pts',(7.09309599630155,-0.0494916155961562,
-0.726605082296128));
#10863=CARTESIAN_POINT('Ctrl Pts',(7.0931279909255,-1.20749723881847E-5,
-0.729157655282255));
#10864=CARTESIAN_POINT('Ctrl Pts',(7.09310750107417,6.92000663027083E-5,
-0.620842344717746));
#10865=CARTESIAN_POINT('Ctrl Pts',(7.09301232990392,0.0463117993985499,
-0.623228399614835));
#10866=CARTESIAN_POINT('Ctrl Pts',(7.12436976205869,0.193855808404846,-0.630847792090333));
#10867=CARTESIAN_POINT('Ctrl Pts',(7.35144068066377,0.358654235479558,-0.643700522144239));
#10868=CARTESIAN_POINT('Ctrl Pts',(7.67235860481237,0.238352634675404,-0.659400534879465));
#10869=CARTESIAN_POINT('Ctrl Pts',(7.74904981361332,-0.0956833658965494,
-0.675100547614689));
#10870=CARTESIAN_POINT('Ctrl Pts',(7.51274499136877,-0.343916540891515,
-0.690800560349916));
#10871=CARTESIAN_POINT('Ctrl Pts',(7.18506994739396,-0.285496471322637,
-0.706047826050933));
#10872=CARTESIAN_POINT('Ctrl Pts',(7.09279950075169,-0.0918449016015606,
-0.716061754173544));
#10873=CARTESIAN_POINT('Ctrl Pts',(7.09225513659108,0.000146978884224968,
-0.720842344717746));
#10874=CARTESIAN_POINT('Origin',(7.4,0.,0.220842344717745));
#10875=CARTESIAN_POINT('',(7.09247298313668,-0.000242065099788365,-0.520842344717745));
#10876=CARTESIAN_POINT('',(7.09269677699397,0.000264518140442497,-0.529157655282254));
#10877=CARTESIAN_POINT('',(7.09265,5.61065397787037E-15,0.220842344717745));
#10878=CARTESIAN_POINT('Ctrl Pts',(7.09269677699397,0.000264518140442521,
-0.529157655282254));
#10879=CARTESIAN_POINT('Ctrl Pts',(7.09247596806863,0.0256450895838866,
-0.530471698021893));
#10880=CARTESIAN_POINT('Ctrl Pts',(7.10686696713217,0.151860064204999,-0.537019078339939));
#10881=CARTESIAN_POINT('Ctrl Pts',(7.28044779410479,0.341611292216308,-0.548799796236394));
#10882=CARTESIAN_POINT('Ctrl Pts',(7.61898033631151,0.288164184858654,-0.564499808971621));
#10883=CARTESIAN_POINT('Ctrl Pts',(7.76115116184634,-0.0236824514715945,
-0.580199821706845));
#10884=CARTESIAN_POINT('Ctrl Pts',(7.57947417153963,-0.314292927621228,
-0.595899834442071));
#10885=CARTESIAN_POINT('Ctrl Pts',(7.23686118017403,-0.323073675801685,
-0.611599847177295));
#10886=CARTESIAN_POINT('Ctrl Pts',(7.09823388955116,-0.12471174942936,-0.622685787457357));
#10887=CARTESIAN_POINT('Ctrl Pts',(7.0922373003074,-0.0121115682384182,
-0.62853839015901));
#10888=CARTESIAN_POINT('Ctrl Pts',(7.09232382992685,-0.000188032469277427,
-0.629157655282255));
#10889=CARTESIAN_POINT('Ctrl Pts',(7.09247298313668,-0.000242065099788339,
-0.520842344717745));
#10890=CARTESIAN_POINT('Ctrl Pts',(7.09319155660411,0.0830296003080465,
-0.525161707477718));
#10891=CARTESIAN_POINT('Ctrl Pts',(7.17081384475125,0.268374363352796,-0.534714407816098));
#10892=CARTESIAN_POINT('Ctrl Pts',(7.4824566420967,0.352408704334569,-0.549500445732887));
#10893=CARTESIAN_POINT('Ctrl Pts',(7.73942346970471,0.125629234627381,-0.565200458468113));
#10894=CARTESIAN_POINT('Ctrl Pts',(7.69202601364555,-0.213803194390989,
-0.580900471203338));
#10895=CARTESIAN_POINT('Ctrl Pts',(7.38276603381877,-0.361516208756931,
-0.596600483938563));
#10896=CARTESIAN_POINT('Ctrl Pts',(7.13361194494272,-0.211872566628196,
-0.609914441776699));
#10897=CARTESIAN_POINT('Ctrl Pts',(7.09322106896615,-0.0551121590794967,
-0.617995062036427));
#10898=CARTESIAN_POINT('Ctrl Pts',(7.09310750107417,6.92000663027083E-5,
-0.620842344717746));
#10899=CARTESIAN_POINT('Origin',(7.4,0.,0.220842344717745));
#10900=CARTESIAN_POINT('',(7.09253120772146,0.000253844832670602,-0.420842344717745));
#10901=CARTESIAN_POINT('',(7.09301111964154,-0.000175545644984122,-0.429157655282254));
#10902=CARTESIAN_POINT('',(7.09265,5.61065397787037E-15,0.220842344717745));
#10903=CARTESIAN_POINT('Ctrl Pts',(7.09301111964154,-0.000175545644984097,
-0.429157655282254));
#10904=CARTESIAN_POINT('Ctrl Pts',(7.0933462412372,0.0627096616204277,-0.432405005884775));
#10905=CARTESIAN_POINT('Ctrl Pts',(7.14252715445512,0.227420166767621,-0.440885694065704));
#10906=CARTESIAN_POINT('Ctrl Pts',(7.41005148992723,0.36178718690615,-0.454599719825043));
#10907=CARTESIAN_POINT('Ctrl Pts',(7.70730390568508,0.191194430604527,-0.470299732560268));
#10908=CARTESIAN_POINT('Ctrl Pts',(7.72899396184246,-0.150844204963527,
-0.485999745295493));
#10909=CARTESIAN_POINT('Ctrl Pts',(7.45567197464232,-0.357619396607422,
-0.501699758030719));
#10910=CARTESIAN_POINT('Ctrl Pts',(7.15948288929725,-0.253247385241686,
-0.516085728026305));
#10911=CARTESIAN_POINT('Ctrl Pts',(7.09335536689775,-0.0754361723033938,
-0.525238360443484));
#10912=CARTESIAN_POINT('Ctrl Pts',(7.09269677699397,0.000264518140442521,
-0.529157655282254));
#10913=CARTESIAN_POINT('Ctrl Pts',(7.09253120772146,0.000253844832670647,
-0.420842344717745));
#10914=CARTESIAN_POINT('Ctrl Pts',(7.09235750988509,0.019914890942319,-0.421861677762192));
#10915=CARTESIAN_POINT('Ctrl Pts',(7.10295953403298,0.140330854235573,-0.428114348385046));
#10916=CARTESIAN_POINT('Ctrl Pts',(7.26166496025002,0.334446425349789,-0.43960035658631));
#10917=CARTESIAN_POINT('Ctrl Pts',(7.60264283707619,0.299878100557217,-0.455300369321535));
#10918=CARTESIAN_POINT('Ctrl Pts',(7.76190893784147,-0.00359379375923244,
-0.47100038205676));
#10919=CARTESIAN_POINT('Ctrl Pts',(7.59664782201734,-0.303843099024022,
-0.486700394791986));
#10920=CARTESIAN_POINT('Ctrl Pts',(7.25505071769875,-0.33163338187372,-0.502400407527211));
#10921=CARTESIAN_POINT('Ctrl Pts',(7.10165150153385,-0.136213608107123,
-0.513781057502464));
#10922=CARTESIAN_POINT('Ctrl Pts',(7.09232093338052,-0.0178623043576069,
-0.519928369899309));
#10923=CARTESIAN_POINT('Ctrl Pts',(7.09247298313668,-0.000242065099788339,
-0.520842344717745));
#10924=CARTESIAN_POINT('Origin',(7.4,0.,0.220842344717745));
#10925=CARTESIAN_POINT('',(7.09309040722717,-9.95083455336276E-5,-0.320842344717745));
#10926=CARTESIAN_POINT('',(7.09216516823616,-1.80303458139274E-5,-0.329157655282254));
#10927=CARTESIAN_POINT('',(7.09265,5.61065397787037E-15,0.220842344717745));
#10928=CARTESIAN_POINT('Ctrl Pts',(7.09216516823616,-1.80303458139253E-5,
-0.329157655282254));
#10929=CARTESIAN_POINT('Ctrl Pts',(7.09225161220405,0.0995954773657983,
-0.334338313747658));
#10930=CARTESIAN_POINT('Ctrl Pts',(7.19850125980854,0.299994096800775,-0.34475230979147));
#10931=CARTESIAN_POINT('Ctrl Pts',(7.53833504309277,0.334446433431464,-0.36039964341369));
#10932=CARTESIAN_POINT('Ctrl Pts',(7.75526656789289,0.0691134335902364,
-0.376099656148916));
#10933=CARTESIAN_POINT('Ctrl Pts',(7.65362715299794,-0.25819424514732,-0.391799668884141));
#10934=CARTESIAN_POINT('Ctrl Pts',(7.32455783679988,-0.353976667301946,
-0.407499681619366));
#10935=CARTESIAN_POINT('Ctrl Pts',(7.11720959661094,-0.178186582951383,
-0.419952343752071));
#10936=CARTESIAN_POINT('Ctrl Pts',(7.09280616883524,-0.0386343441831341,
-0.427171668306367));
#10937=CARTESIAN_POINT('Ctrl Pts',(7.09301111964154,-0.000175545644984097,
-0.429157655282254));
#10938=CARTESIAN_POINT('Ctrl Pts',(7.09309040722717,-9.95083455336103E-5,
-0.320842344717745));
#10939=CARTESIAN_POINT('Ctrl Pts',(7.09326037605201,0.0571157331677331,
-0.323794985625074));
#10940=CARTESIAN_POINT('Ctrl Pts',(7.13587712268272,0.215975955054746,-0.331980964110812));
#10941=CARTESIAN_POINT('Ctrl Pts',(7.38994851031558,0.361787178163918,-0.345400280174957));
#10942=CARTESIAN_POINT('Ctrl Pts',(7.69621418650062,0.207961896411083,-0.361100292910183));
#10943=CARTESIAN_POINT('Ctrl Pts',(7.73686175971175,-0.132344812727946,
-0.376800305645408));
#10944=CARTESIAN_POINT('Ctrl Pts',(7.47544216137711,-0.353976658748332,
-0.392500318380634));
#10945=CARTESIAN_POINT('Ctrl Pts',(7.16773788164802,-0.264412971801384,
-0.407180998071412));
#10946=CARTESIAN_POINT('Ctrl Pts',(7.09324928850379,-0.0810264961705937,
-0.416628340183783));
#10947=CARTESIAN_POINT('Ctrl Pts',(7.09253120772146,0.000253844832670647,
-0.420842344717745));
#10948=CARTESIAN_POINT('Origin',(7.4,0.,0.220842344717745));
#10949=CARTESIAN_POINT('',(7.0922195431951,-0.00011439326538178,-0.220842344717745));
#10950=CARTESIAN_POINT('',(7.09297247873625,0.000198368389210363,-0.229157655282254));
#10951=CARTESIAN_POINT('',(7.09265,5.61065397787037E-15,0.220842344717745));
#10952=CARTESIAN_POINT('Ctrl Pts',(7.09297247873625,0.000198368389210352,
-0.229157655282254));
#10953=CARTESIAN_POINT('Ctrl Pts',(7.09275135076004,0.0366053523330718,
-0.231038284032132));
#10954=CARTESIAN_POINT('Ctrl Pts',(7.11545131658584,0.174057577268075,-0.238152250360418));
#10955=CARTESIAN_POINT('Ctrl Pts',(7.31754335591095,0.352408712852604,-0.250499554267113));
#10956=CARTESIAN_POINT('Ctrl Pts',(7.64844985249427,0.263179923979787,-0.266199567002338));
#10957=CARTESIAN_POINT('Ctrl Pts',(7.75656898334281,-0.062044832321089,
-0.281899579737564));
#10958=CARTESIAN_POINT('Ctrl Pts',(7.54494928580385,-0.331633389887768,
-0.297599592472789));
#10959=CARTESIAN_POINT('Ctrl Pts',(7.20335217323078,-0.303843106366043,
-0.313299605208014));
#10960=CARTESIAN_POINT('Ctrl Pts',(7.09262358366168,-0.102669455049145,
-0.323818959477836));
#10961=CARTESIAN_POINT('Ctrl Pts',(7.09216428923756,-0.00103094236550998,
-0.329104976169249));
#10962=CARTESIAN_POINT('Ctrl Pts',(7.09216516823616,-1.80303458139253E-5,
-0.329157655282254));
#10963=CARTESIAN_POINT('Ctrl Pts',(7.0922195431951,-0.000114393265381769,
-0.220842344717745));
#10964=CARTESIAN_POINT('Ctrl Pts',(7.09267485594448,0.0938769082790096,
-0.225728293487957));
#10965=CARTESIAN_POINT('Ctrl Pts',(7.1885102624992,0.28934678370451,-0.235847579836577));
#10966=CARTESIAN_POINT('Ctrl Pts',(7.51955220300225,0.341611283968803,-0.251200203763605));
#10967=CARTESIAN_POINT('Ctrl Pts',(7.7508811552982,0.0887322446241938,-0.266900216498831));
#10968=CARTESIAN_POINT('Ctrl Pts',(7.66757159672246,-0.243713834945875,
-0.282600229234056));
#10969=CARTESIAN_POINT('Ctrl Pts',(7.34432802670357,-0.357619387966788,
-0.298300241969282));
#10970=CARTESIAN_POINT('Ctrl Pts',(7.12240865796432,-0.189731614023667,
-0.311047613797178));
#10971=CARTESIAN_POINT('Ctrl Pts',(7.0929591188839,-0.044294049757736,-0.318561648046666));
#10972=CARTESIAN_POINT('Ctrl Pts',(7.09309040722717,-9.95083455336103E-5,
-0.320842344717745));
#10973=CARTESIAN_POINT('Origin',(7.4,0.,0.220842344717745));
#10974=CARTESIAN_POINT('',(7.09284095646985,0.00024563841227826,-0.120842344717745));
#10975=CARTESIAN_POINT('',(7.09275435891078,-0.00026066578654145,-0.129157655282254));
#10976=CARTESIAN_POINT('',(7.09265,5.61065397787037E-15,0.220842344717745));
#10977=CARTESIAN_POINT('Ctrl Pts',(7.09275435891078,-0.000260665786541426,
-0.129157655282254));
#10978=CARTESIAN_POINT('Ctrl Pts',(7.09337515152961,0.0734403268284316,
-0.132971591895015));
#10979=CARTESIAN_POINT('Ctrl Pts',(7.15665481869895,0.249228823319743,-0.142018866086184));
#10980=CARTESIAN_POINT('Ctrl Pts',(7.4485593205266,0.358654244252335,-0.156299477855761));
#10981=CARTESIAN_POINT('Ctrl Pts',(7.72593357368315,0.157347793593328,-0.171999490590986));
#10982=CARTESIAN_POINT('Ctrl Pts',(7.71104009926825,-0.185054253822684,
-0.187699503326212));
#10983=CARTESIAN_POINT('Ctrl Pts',(7.41723396659593,-0.361516217508599,
-0.203399516061437));
#10984=CARTESIAN_POINT('Ctrl Pts',(7.14501874054224,-0.231497029037679,
-0.217218900046785));
#10985=CARTESIAN_POINT('Ctrl Pts',(7.09336669674346,-0.0647065292396766,
-0.225804946453724));
#10986=CARTESIAN_POINT('Ctrl Pts',(7.09297247873625,0.000198368389210352,
-0.229157655282254));
#10987=CARTESIAN_POINT('Ctrl Pts',(7.09284095646985,0.000245638412278346,
-0.120842344717745));
#10988=CARTESIAN_POINT('Ctrl Pts',(7.09260231732278,0.0309143893015408,
-0.122428263772431));
#10989=CARTESIAN_POINT('Ctrl Pts',(7.11080461894951,0.162509776943659,-0.129247520405525));
#10990=CARTESIAN_POINT('Ctrl Pts',(7.2981047634038,0.347285733851148,-0.141300114617028));
#10991=CARTESIAN_POINT('Ctrl Pts',(7.63345360120587,0.276569150443068,-0.157000127352253));
#10992=CARTESIAN_POINT('Ctrl Pts',(7.75946408208296,-0.0421516519758924,
-0.172700140087479));
#10993=CARTESIAN_POINT('Ctrl Pts',(7.56313881583769,-0.323073667897745,
-0.188400152822704));
#10994=CARTESIAN_POINT('Ctrl Pts',(7.22052583282271,-0.314292920077652,
-0.20410016555793));
#10995=CARTESIAN_POINT('Ctrl Pts',(7.09538793769919,-0.11412236888846,-0.214914229522943));
#10996=CARTESIAN_POINT('Ctrl Pts',(7.09218717065892,-0.00679713345771461,
-0.220494955909548));
#10997=CARTESIAN_POINT('Ctrl Pts',(7.0922195431951,-0.000114393265381769,
-0.220842344717745));
#10998=CARTESIAN_POINT('Origin',(7.4,0.,0.220842344717745));
#10999=CARTESIAN_POINT('',(7.09298021495369,-0.000306384811325694,-0.0208423447177452));
#11000=CARTESIAN_POINT('',(7.09227939521384,0.000154311006394861,-0.0291576552822542));
#11001=CARTESIAN_POINT('',(7.09265,5.61065397787037E-15,0.220842344717745));
#11002=CARTESIAN_POINT('',(7.32062007174671,-0.29692229537457,0.));
#11003=CARTESIAN_POINT('Ctrl Pts',(7.32062007174671,-0.29692229537457,0.));
#11004=CARTESIAN_POINT('Ctrl Pts',(7.22298599415769,-0.270820563726849,
-0.00523333757840845));
#11005=CARTESIAN_POINT('Ctrl Pts',(7.11285656998777,-0.167549921885641,
-0.0121807858176569));
#11006=CARTESIAN_POINT('Ctrl Pts',(7.09275376795427,-0.0334730859377096,
-0.0191282340569053));
#11007=CARTESIAN_POINT('Ctrl Pts',(7.09298021495369,-0.000306384811325677,
-0.0208423447177452));
#11008=CARTESIAN_POINT('',(7.47957997103547,-0.297398060845569,-1.37807245336141E-17));
#11009=CARTESIAN_POINT('Origin',(7.4,0.,0.));
#11010=CARTESIAN_POINT('Ctrl Pts',(7.47958090815733,-0.297400289619931,
-6.50521303491303E-19));
#11011=CARTESIAN_POINT('Ctrl Pts',(7.38660350274273,-0.321949666906663,
-0.00499978774624428));
#11012=CARTESIAN_POINT('Ctrl Pts',(7.18097790240557,-0.278640224120542,
-0.0147190061736624));
#11013=CARTESIAN_POINT('Ctrl Pts',(7.09286421205138,-0.0906630570237555,
-0.0244382246010804));
#11014=CARTESIAN_POINT('Ctrl Pts',(7.09227939521384,0.000154311006394901,
-0.0291576552822542));
#11015=CARTESIAN_POINT('Origin',(-7.4,0.,0.220842344717745));
#11016=CARTESIAN_POINT('',(-7.70774490082263,0.000146975295764101,-0.720842344717746));
#11017=CARTESIAN_POINT('',(-7.70687196406169,-1.20609381283741E-5,-0.729157655282255));
#11018=CARTESIAN_POINT('',(-7.70735,5.61059503063532E-15,0.220842344717745));
#11019=CARTESIAN_POINT('',(-7.32062007174671,-0.296922295374569,-0.8));
#11020=CARTESIAN_POINT('Ctrl Pts',(-7.70687196406169,-1.20609381283332E-5,
-0.729157655282254));
#11021=CARTESIAN_POINT('Ctrl Pts',(-7.7068383611135,0.0519523715634962,
-0.731838419874536));
#11022=CARTESIAN_POINT('Ctrl Pts',(-7.66983365783928,0.205395707970149,
-0.739752522045225));
#11023=CARTESIAN_POINT('Ctrl Pts',(-7.42863574303655,0.360721611690756,
-0.752899961794324));
#11024=CARTESIAN_POINT('Ctrl Pts',(-7.1146964728348,0.223016315327006,-0.768599974529548));
#11025=CARTESIAN_POINT('Ctrl Pts',(-7.05707047975879,-0.115238727497404,
-0.784299987264776));
#11026=CARTESIAN_POINT('Ctrl Pts',(-7.22298599415769,-0.270820563726849,
-0.794766662421592));
#11027=CARTESIAN_POINT('Ctrl Pts',(-7.32062007174671,-0.29692229537457,
-0.8));
#11028=CARTESIAN_POINT('',(-7.47958000049154,-0.297398061564379,-0.8));
#11029=CARTESIAN_POINT('Origin',(-7.4,0.,-0.8));
#11030=CARTESIAN_POINT('Ctrl Pts',(-7.70774490082263,0.000146975295764138,
-0.720842344717746));
#11031=CARTESIAN_POINT('Ctrl Pts',(-7.70779645502102,0.00885909073304824,
-0.721295091751952));
#11032=CARTESIAN_POINT('Ctrl Pts',(-7.7035433750236,0.118223822401162,-0.726981176364568));
#11033=CARTESIAN_POINT('Ctrl Pts',(-7.57319886321716,0.317782926109968,
-0.737900598555591));
#11034=CARTESIAN_POINT('Ctrl Pts',(-7.23047488314852,0.319794760031351,
-0.753600611290816));
#11035=CARTESIAN_POINT('Ctrl Pts',(-7.03977528830754,0.0349557588279105,
-0.769300624026042));
#11036=CARTESIAN_POINT('Ctrl Pts',(-7.17010530135127,-0.276350328985862,
-0.784767086929102));
#11037=CARTESIAN_POINT('Ctrl Pts',(-7.38660355712988,-0.321949646446656,
-0.795000212253755));
#11038=CARTESIAN_POINT('Ctrl Pts',(-7.47958093846728,-0.297400292044456,
-0.799999999999999));
#11039=CARTESIAN_POINT('Origin',(-7.4,0.,0.220842344717745));
#11040=CARTESIAN_POINT('',(-7.70689253729186,6.92000104607349E-5,-0.620842344717746));
#11041=CARTESIAN_POINT('',(-7.70767612478914,-0.000188032618375286,-0.629157655282255));
#11042=CARTESIAN_POINT('',(-7.70735,5.61059503063532E-15,0.220842344717745));
#11043=CARTESIAN_POINT('Ctrl Pts',(-7.70767612478914,-0.000188032618375274,
-0.629157655282255));
#11044=CARTESIAN_POINT('Ctrl Pts',(-7.70703140259473,0.0886528337709136,
-0.633771727737419));
#11045=CARTESIAN_POINT('Ctrl Pts',(-7.62022620581121,0.27935843464658,-0.643619137770991));
#11046=CARTESIAN_POINT('Ctrl Pts',(-7.29810477724755,0.347285687712531,
-0.658699885382972));
#11047=CARTESIAN_POINT('Ctrl Pts',(-7.05412291905423,0.106591912271656,
-0.674399898118197));
#11048=CARTESIAN_POINT('Ctrl Pts',(-7.12029939040689,-0.229692046472377,
-0.690099910853423));
#11049=CARTESIAN_POINT('Ctrl Pts',(-7.43727189946158,-0.359992421881043,
-0.705799923588648));
#11050=CARTESIAN_POINT('Ctrl Pts',(-7.67243004463156,-0.200382402588913,
-0.718819171731592));
#11051=CARTESIAN_POINT('Ctrl Pts',(-7.70690396014894,-0.0494916038360727,
-0.726605082296127));
#11052=CARTESIAN_POINT('Ctrl Pts',(-7.70687196406169,-1.20609381283332E-5,
-0.729157655282254));
#11053=CARTESIAN_POINT('Ctrl Pts',(-7.70689253729186,6.92000104607314E-5,
-0.620842344717745));
#11054=CARTESIAN_POINT('Ctrl Pts',(-7.70698770847048,0.0463118050970373,
-0.623228399614835));
#11055=CARTESIAN_POINT('Ctrl Pts',(-7.67563027239018,0.193855832506279,
-0.630847792090332));
#11056=CARTESIAN_POINT('Ctrl Pts',(-7.44855932549587,0.358654280875835,
-0.643700522144239));
#11057=CARTESIAN_POINT('Ctrl Pts',(-7.12764136094462,0.238352663458736,
-0.659400534879464));
#11058=CARTESIAN_POINT('Ctrl Pts',(-7.05095014313138,-0.0956833759672795,
-0.675100547614689));
#11059=CARTESIAN_POINT('Ctrl Pts',(-7.28725499370478,-0.34391658738075,
-0.690800560349915));
#11060=CARTESIAN_POINT('Ctrl Pts',(-7.61493008115263,-0.285496500960074,
-0.706047826050934));
#11061=CARTESIAN_POINT('Ctrl Pts',(-7.70720053610084,-0.0918449175996906,
-0.716061754173544));
#11062=CARTESIAN_POINT('Ctrl Pts',(-7.70774490082263,0.000146975295764138,
-0.720842344717746));
#11063=CARTESIAN_POINT('Origin',(-7.4,0.,0.220842344717745));
#11064=CARTESIAN_POINT('',(-7.70752705531861,-0.000242065129798921,-0.520842344717746));
#11065=CARTESIAN_POINT('',(-7.70730317768915,0.000264518094095117,-0.529157655282254));
#11066=CARTESIAN_POINT('',(-7.70735,5.61059503063532E-15,0.220842344717745));
#11067=CARTESIAN_POINT('Ctrl Pts',(-7.70730317768915,0.000264518094095133,
-0.529157655282254));
#11068=CARTESIAN_POINT('Ctrl Pts',(-7.70752398658218,0.0256450857940224,
-0.530471698021893));
#11069=CARTESIAN_POINT('Ctrl Pts',(-7.69313298964038,0.151860041802368,
-0.53701907833994));
#11070=CARTESIAN_POINT('Ctrl Pts',(-7.51955218823887,0.341611241880446,
-0.548799796236394));
#11071=CARTESIAN_POINT('Ctrl Pts',(-7.18101969602976,0.288164142274201,
-0.56449980897162));
#11072=CARTESIAN_POINT('Ctrl Pts',(-7.03884889133106,-0.0236824478145123,
-0.580199821706845));
#11073=CARTESIAN_POINT('Ctrl Pts',(-7.22052585508497,-0.314292881582478,
-0.595899834442071));
#11074=CARTESIAN_POINT('Ctrl Pts',(-7.56313879548406,-0.323073627560531,
-0.611599847177296));
#11075=CARTESIAN_POINT('Ctrl Pts',(-7.70176606621786,-0.124711731655602,
-0.622685787457357));
#11076=CARTESIAN_POINT('Ctrl Pts',(-7.70776265441629,-0.0121115666782128,
-0.62853839015901));
#11077=CARTESIAN_POINT('Ctrl Pts',(-7.70767612478914,-0.000188032618375274,
-0.629157655282255));
#11078=CARTESIAN_POINT('Ctrl Pts',(-7.70752705531861,-0.000242065129798906,
-0.520842344717745));
#11079=CARTESIAN_POINT('Ctrl Pts',(-7.70680848176124,0.0830296106897686,
-0.525161707477718));
#11080=CARTESIAN_POINT('Ctrl Pts',(-7.62918618390742,0.268374396907059,
-0.534714407816098));
#11081=CARTESIAN_POINT('Ctrl Pts',(-7.31754334759326,0.352408748413955,
-0.549500445732887));
#11082=CARTESIAN_POINT('Ctrl Pts',(-7.06057648784951,0.125629250314373,
-0.565200458468112));
#11083=CARTESIAN_POINT('Ctrl Pts',(-7.10797394984171,-0.213803221083396,
-0.580900471203338));
#11084=CARTESIAN_POINT('Ctrl Pts',(-7.41723396832727,-0.361516254045136,
-0.596600483938562));
#11085=CARTESIAN_POINT('Ctrl Pts',(-7.66638808838325,-0.211872593003345,
-0.609914441776699));
#11086=CARTESIAN_POINT('Ctrl Pts',(-7.70677896938989,-0.0551121660019896,
-0.617995062036427));
#11087=CARTESIAN_POINT('Ctrl Pts',(-7.70689253729186,6.92000104607314E-5,
-0.620842344717745));
#11088=CARTESIAN_POINT('Origin',(-7.4,0.,0.220842344717745));
#11089=CARTESIAN_POINT('',(-7.70746883072654,0.000253844864433833,-0.420842344717745));
#11090=CARTESIAN_POINT('',(-7.70698883508382,-0.000175545619141625,-0.429157655282254));
#11091=CARTESIAN_POINT('',(-7.70735,5.61059503063532E-15,0.220842344717745));
#11092=CARTESIAN_POINT('Ctrl Pts',(-7.70698883508383,-0.000175545619141616,
-0.429157655282254));
#11093=CARTESIAN_POINT('Ctrl Pts',(-7.70665371353763,0.0627096523718999,
-0.432405005884775));
#11094=CARTESIAN_POINT('Ctrl Pts',(-7.65747280757301,0.227420133227449,
-0.440885694065705));
#11095=CARTESIAN_POINT('Ctrl Pts',(-7.38994851155463,0.361787133550707,
-0.454599719825042));
#11096=CARTESIAN_POINT('Ctrl Pts',(-7.09269613963708,0.191194402405521,
-0.470299732560268));
#11097=CARTESIAN_POINT('Ctrl Pts',(-7.07100608667554,-0.15084418271379,
-0.485999745295493));
#11098=CARTESIAN_POINT('Ctrl Pts',(-7.34432803357192,-0.357619343872072,
-0.501699758030719));
#11099=CARTESIAN_POINT('Ctrl Pts',(-7.64051707522517,-0.253247347882201,
-0.516085728026305));
#11100=CARTESIAN_POINT('Ctrl Pts',(-7.70664458788177,-0.0754361611842396,
-0.525238360443484));
#11101=CARTESIAN_POINT('Ctrl Pts',(-7.70730317768915,0.000264518094095133,
-0.529157655282254));
#11102=CARTESIAN_POINT('Ctrl Pts',(-7.70746883072654,0.000253844864433892,
-0.420842344717745));
#11103=CARTESIAN_POINT('Ctrl Pts',(-7.70764252858464,0.0199148934326357,
-0.421861677762192));
#11104=CARTESIAN_POINT('Ctrl Pts',(-7.69704050311101,0.140330871783531,
-0.428114348385046));
#11105=CARTESIAN_POINT('Ctrl Pts',(-7.53833505704833,0.334446467171126,
-0.43960035658631));
#11106=CARTESIAN_POINT('Ctrl Pts',(-7.19735713758398,0.299878138056265,
-0.455300369321535));
#11107=CARTESIAN_POINT('Ctrl Pts',(-7.03809101690294,-0.0035937942090703,
-0.47100038205676));
#11108=CARTESIAN_POINT('Ctrl Pts',(-7.20335215339251,-0.30384313701778,
-0.486700394791986));
#11109=CARTESIAN_POINT('Ctrl Pts',(-7.54494930042661,-0.331633423345088,
-0.50240040752721));
#11110=CARTESIAN_POINT('Ctrl Pts',(-7.6983485357738,-0.136213625138345,
-0.513781057502464));
#11111=CARTESIAN_POINT('Ctrl Pts',(-7.7076791050938,-0.0178623065907353,
-0.519928369899309));
#11112=CARTESIAN_POINT('Ctrl Pts',(-7.70752705531861,-0.000242065129798906,
-0.520842344717745));
#11113=CARTESIAN_POINT('Origin',(-7.4,0.,0.220842344717745));
#11114=CARTESIAN_POINT('',(-7.70690963115052,-9.95083586281809E-5,-0.320842344717745));
#11115=CARTESIAN_POINT('',(-7.7078347863644,-1.80303430137119E-5,-0.329157655282254));
#11116=CARTESIAN_POINT('',(-7.70735,5.61059503063532E-15,0.220842344717745));
#11117=CARTESIAN_POINT('Ctrl Pts',(-7.70783478636441,-1.80303430137095E-5,
-0.329157655282254));
#11118=CARTESIAN_POINT('Ctrl Pts',(-7.70774834240926,0.0995954626777301,
-0.334338313747658));
#11119=CARTESIAN_POINT('Ctrl Pts',(-7.60149871047448,0.299994052557417,
-0.34475230979147));
#11120=CARTESIAN_POINT('Ctrl Pts',(-7.26166497730884,0.334446384107517,
-0.36039964341369));
#11121=CARTESIAN_POINT('Ctrl Pts',(-7.04473348450178,0.0691134233972956,
-0.376099656148916));
#11122=CARTESIAN_POINT('Ctrl Pts',(-7.14637288440692,-0.258194207068779,
-0.391799668884141));
#11123=CARTESIAN_POINT('Ctrl Pts',(-7.47544215207399,-0.353976615097665,
-0.407499681619366));
#11124=CARTESIAN_POINT('Ctrl Pts',(-7.68279036168308,-0.178186556672294,
-0.419952343752071));
#11125=CARTESIAN_POINT('Ctrl Pts',(-7.70719378585987,-0.0386343384853514,
-0.427171668306367));
#11126=CARTESIAN_POINT('Ctrl Pts',(-7.70698883508383,-0.000175545619141616,
-0.429157655282254));
#11127=CARTESIAN_POINT('Ctrl Pts',(-7.70690963115052,-9.95083586281427E-5,
-0.320842344717745));
#11128=CARTESIAN_POINT('Ctrl Pts',(-7.70673966230461,0.0571157403095281,
-0.323794985625074));
#11129=CARTESIAN_POINT('Ctrl Pts',(-7.66412291034569,0.215975982062961,
-0.331980964110812));
#11130=CARTESIAN_POINT('Ctrl Pts',(-7.41005149094087,0.36178722340353,-0.345400280174957));
#11131=CARTESIAN_POINT('Ctrl Pts',(-7.10378577645897,0.207961922416443,
-0.361100292910183));
#11132=CARTESIAN_POINT('Ctrl Pts',(-7.06313819816462,-0.132344829277446,
-0.376800305645408));
#11133=CARTESIAN_POINT('Ctrl Pts',(-7.32455782918916,-0.35397670301188,
-0.392500318380633));
#11134=CARTESIAN_POINT('Ctrl Pts',(-7.6322621473956,-0.264413004865462,
-0.407180998071413));
#11135=CARTESIAN_POINT('Ctrl Pts',(-7.70675074985441,-0.081026506302691,
-0.416628340183783));
#11136=CARTESIAN_POINT('Ctrl Pts',(-7.70746883072654,0.000253844864433892,
-0.420842344717745));
#11137=CARTESIAN_POINT('Origin',(-7.4,0.,0.220842344717745));
#11138=CARTESIAN_POINT('',(-7.70778049527,-0.000114393321009997,-0.220842344717745));
#11139=CARTESIAN_POINT('',(-7.70702747598399,0.000198368355311817,-0.229157655282254));
#11140=CARTESIAN_POINT('',(-7.70735,5.61059503063532E-15,0.220842344717745));
#11141=CARTESIAN_POINT('Ctrl Pts',(-7.70702747598399,0.000198368355311809,
-0.229157655282254));
#11142=CARTESIAN_POINT('Ctrl Pts',(-7.70724860392715,0.0366053469345374,
-0.231038284032132));
#11143=CARTESIAN_POINT('Ctrl Pts',(-7.68454864144738,0.17405755161616,-0.238152250360418));
#11144=CARTESIAN_POINT('Ctrl Pts',(-7.48245663192943,0.352408660865427,
-0.250499554267113));
#11145=CARTESIAN_POINT('Ctrl Pts',(-7.15155018414657,0.263179885173358,
-0.266199567002338));
#11146=CARTESIAN_POINT('Ctrl Pts',(-7.04343106924415,-0.0620448231745263,
-0.281899579737564));
#11147=CARTESIAN_POINT('Ctrl Pts',(-7.25505073557315,-0.331633340976559,
-0.297599592472789));
#11148=CARTESIAN_POINT('Ctrl Pts',(-7.59664779776768,-0.303843061556337,
-0.313299605208015));
#11149=CARTESIAN_POINT('Ctrl Pts',(-7.7073763710065,-0.102669439907453,
-0.323818959477836));
#11150=CARTESIAN_POINT('Ctrl Pts',(-7.70783566536288,-0.00103094221332684,
-0.329104976169249));
#11151=CARTESIAN_POINT('Ctrl Pts',(-7.70783478636441,-1.80303430137095E-5,
-0.329157655282254));
#11152=CARTESIAN_POINT('Ctrl Pts',(-7.70778049527,-0.000114393321009984,
-0.220842344717745));
#11153=CARTESIAN_POINT('Ctrl Pts',(-7.70732518245543,0.0938769199589478,
-0.225728293487957));
#11154=CARTESIAN_POINT('Ctrl Pts',(-7.61148976398448,0.289346819956445,
-0.235847579836577));
#11155=CARTESIAN_POINT('Ctrl Pts',(-7.28044778202723,0.341611326648396,
-0.251200203763605));
#11156=CARTESIAN_POINT('Ctrl Pts',(-7.04911880083639,0.0887322557395692,
-0.266900216498831));
#11157=CARTESIAN_POINT('Ctrl Pts',(-7.13242836981262,-0.243713865431744,
-0.282600229234056));
#11158=CARTESIAN_POINT('Ctrl Pts',(-7.45567198026117,-0.357619432680664,
-0.298300241969282));
#11159=CARTESIAN_POINT('Ctrl Pts',(-7.67759137674685,-0.189731637750237,
-0.311047613797178));
#11160=CARTESIAN_POINT('Ctrl Pts',(-7.70704091951006,-0.0442940552974542,
-0.318561648046666));
#11161=CARTESIAN_POINT('Ctrl Pts',(-7.70690963115052,-9.95083586281427E-5,
-0.320842344717745));
#11162=CARTESIAN_POINT('Origin',(-7.4,0.,0.220842344717745));
#11163=CARTESIAN_POINT('',(-7.70715908192673,0.00024563889874174,-0.120842344717745));
#11164=CARTESIAN_POINT('',(-7.70724559592217,-0.000260666439420178,-0.129157655282254));
#11165=CARTESIAN_POINT('',(-7.70735,5.61059503063532E-15,0.220842344717745));
#11166=CARTESIAN_POINT('Ctrl Pts',(-7.70724559592217,-0.000260666439420156,
-0.129157655282254));
#11167=CARTESIAN_POINT('Ctrl Pts',(-7.70662480337493,0.0734403154642453,
-0.132971591895015));
#11168=CARTESIAN_POINT('Ctrl Pts',(-7.64334514522135,0.249228787607049,
-0.142018866086183));
#11169=CARTESIAN_POINT('Ctrl Pts',(-7.351440686739,0.358654190708449,-0.156299477855761));
#11170=CARTESIAN_POINT('Ctrl Pts',(-7.07406647433649,0.15734777073398,-0.171999490590986));
#11171=CARTESIAN_POINT('Ctrl Pts',(-7.08895994662689,-0.185054226714597,
-0.187699503326211));
#11172=CARTESIAN_POINT('Ctrl Pts',(-7.38276603593497,-0.36151616409523,
-0.203399516061437));
#11173=CARTESIAN_POINT('Ctrl Pts',(-7.65498122185629,-0.231496994929852,
-0.217218900046784));
#11174=CARTESIAN_POINT('Ctrl Pts',(-7.70663325803569,-0.0647065197097194,
-0.225804946453724));
#11175=CARTESIAN_POINT('Ctrl Pts',(-7.70702747598399,0.000198368355311809,
-0.229157655282254));
#11176=CARTESIAN_POINT('Ctrl Pts',(-7.70715908192673,0.000245638898741782,
-0.120842344717745));
#11177=CARTESIAN_POINT('Ctrl Pts',(-7.7073977208252,0.0309143927359499,
-0.122428263772431));
#11178=CARTESIAN_POINT('Ctrl Pts',(-7.68919541585723,0.162509793267262,
-0.129247520405525));
#11179=CARTESIAN_POINT('Ctrl Pts',(-7.50189525062872,0.347285780617978,
-0.141300114617028));
#11180=CARTESIAN_POINT('Ctrl Pts',(-7.16654636885183,0.276569183243976,
-0.157000127352254));
#11181=CARTESIAN_POINT('Ctrl Pts',(-7.04053587339322,-0.0421516562996225,
-0.172700140087479));
#11182=CARTESIAN_POINT('Ctrl Pts',(-7.23686116352416,-0.323073708797981,
-0.188400152822704));
#11183=CARTESIAN_POINT('Ctrl Pts',(-7.5794741897514,-0.314292959115147,
-0.204100165557929));
#11184=CARTESIAN_POINT('Ctrl Pts',(-7.70461210038305,-0.114122383172389,
-0.214914229522943));
#11185=CARTESIAN_POINT('Ctrl Pts',(-7.70781286781081,-0.00679713434773683,
-0.220494955909549));
#11186=CARTESIAN_POINT('Ctrl Pts',(-7.70778049527,-0.000114393321009984,
-0.220842344717745));
#11187=CARTESIAN_POINT('Origin',(-7.4,0.,0.220842344717745));
#11188=CARTESIAN_POINT('',(-7.70701976654778,-0.00030617080607008,-0.0208423447177452));
#11189=CARTESIAN_POINT('',(-7.70772056490863,0.000154295167761162,-0.0291576552822542));
#11190=CARTESIAN_POINT('',(-7.70735,5.61059503063532E-15,0.220842344717745));
#11191=CARTESIAN_POINT('',(-7.47937992825329,-0.29692229537457,0.));
#11192=CARTESIAN_POINT('Ctrl Pts',(-7.47937992825329,-0.29692229537457,
0.));
#11193=CARTESIAN_POINT('Ctrl Pts',(-7.57701400584231,-0.270820563726849,
-0.00523333757840845));
#11194=CARTESIAN_POINT('Ctrl Pts',(-7.68714337778258,-0.167549582709018,
-0.0121807858176569));
#11195=CARTESIAN_POINT('Ctrl Pts',(-7.7072462053552,-0.0334728379797751,
-0.0191282340569053));
#11196=CARTESIAN_POINT('Ctrl Pts',(-7.70701976654778,-0.000306170806070059,
-0.0208423447177452));
#11197=CARTESIAN_POINT('',(-7.3204200723426,-0.297398060139812,-2.068740934409E-17));
#11198=CARTESIAN_POINT('Origin',(-7.4,0.,0.));
#11199=CARTESIAN_POINT('Ctrl Pts',(-7.32041913648099,-0.297400286396329,
-1.35525271560688E-19));
#11200=CARTESIAN_POINT('Ctrl Pts',(-7.413396577125,-0.321949697150244,-0.00499978774624428));
#11201=CARTESIAN_POINT('Ctrl Pts',(-7.61902199122377,-0.278640078019593,
-0.0147190061736623));
#11202=CARTESIAN_POINT('Ctrl Pts',(-7.70713573379311,-0.0906630403545633,
-0.0244382246010804));
#11203=CARTESIAN_POINT('Ctrl Pts',(-7.70772056490863,0.000154295167761189,
-0.0291576552822542));
#11204=CARTESIAN_POINT('Origin',(0.,-7.4,0.220842344717745));
#11205=CARTESIAN_POINT('',(-0.307744883519712,-7.39985302304706,-0.720842344717745));
#11206=CARTESIAN_POINT('',(-0.306872009074495,-7.40001207497238,-0.729157655282255));
#11207=CARTESIAN_POINT('',(-0.30735,-7.4,0.220842344717745));
#11208=CARTESIAN_POINT('',(0.079379928253284,-7.69692229537457,-0.8));
#11209=CARTESIAN_POINT('Ctrl Pts',(-0.306872009074495,-7.40001207497238,
-0.729157655282255));
#11210=CARTESIAN_POINT('Ctrl Pts',(-0.306838407663091,-7.34804764485915,
-0.731838419874537));
#11211=CARTESIAN_POINT('Ctrl Pts',(-0.269833704177636,-7.1946043063299,
-0.739752522045226));
#11212=CARTESIAN_POINT('Ctrl Pts',(-0.0286357500746574,-7.03927819062664,
-0.752899961794323));
#11213=CARTESIAN_POINT('Ctrl Pts',(0.285303607599647,-7.17698390717715,
-0.76859997452955));
#11214=CARTESIAN_POINT('Ctrl Pts',(0.342929427239765,-7.51523812385981,
-0.784299987264775));
#11215=CARTESIAN_POINT('Ctrl Pts',(0.177014005842305,-7.67082056372685,
-0.794766662421592));
#11216=CARTESIAN_POINT('Ctrl Pts',(0.0793799282532836,-7.69692229537457,
-0.8));
#11217=CARTESIAN_POINT('',(-0.0795799836281317,-7.69739806112894,-0.8));
#11218=CARTESIAN_POINT('Origin',(0.,-7.4,-0.8));
#11219=CARTESIAN_POINT('Ctrl Pts',(-0.307744883519712,-7.39985302304706,
-0.720842344717745));
#11220=CARTESIAN_POINT('Ctrl Pts',(-0.30779643769355,-7.39114090815323,
-0.721295091751952));
#11221=CARTESIAN_POINT('Ctrl Pts',(-0.303543357565344,-7.28177618361729,
-0.726981176364567));
#11222=CARTESIAN_POINT('Ctrl Pts',(-0.173198849645488,-7.08221710163593,
-0.737900598555592));
#11223=CARTESIAN_POINT('Ctrl Pts',(0.169525099592154,-7.08020524213913,
-0.753600611290816));
#11224=CARTESIAN_POINT('Ctrl Pts',(0.360224706479889,-7.36504427094214,
-0.769300624026043));
#11225=CARTESIAN_POINT('Ctrl Pts',(0.229894653244661,-7.67635026824636,
-0.784767086929102));
#11226=CARTESIAN_POINT('Ctrl Pts',(0.0133964740216469,-7.72194965815218,
-0.795000212253756));
#11227=CARTESIAN_POINT('Ctrl Pts',(-0.0795809211152242,-7.69740029063291,
-0.8));
#11228=CARTESIAN_POINT('Origin',(0.,-7.4,0.220842344717745));
#11229=CARTESIAN_POINT('',(-0.306892519549444,-7.39993079996377,-0.620842344717746));
#11230=CARTESIAN_POINT('',(-0.307676170073155,-7.40018803246927,-0.629157655282255));
#11231=CARTESIAN_POINT('',(-0.30735,-7.4,0.220842344717745));
#11232=CARTESIAN_POINT('Ctrl Pts',(-0.307676170073155,-7.40018803246927,
-0.629157655282255));
#11233=CARTESIAN_POINT('Ctrl Pts',(-0.307031447936131,-7.31134715334416,
-0.633771727737419));
#11234=CARTESIAN_POINT('Ctrl Pts',(-0.22022623908268,-7.12064152602881,
-0.643619137770991));
#11235=CARTESIAN_POINT('Ctrl Pts',(0.101895239308332,-7.05271425710996,
-0.658699885382973));
#11236=CARTESIAN_POINT('Ctrl Pts',(0.345877129402089,-7.29340807937902,
-0.674399898118197));
#11237=CARTESIAN_POINT('Ctrl Pts',(0.279700654926715,-7.62969206672302,
-0.690099910853423));
#11238=CARTESIAN_POINT('Ctrl Pts',(-0.0372719110426151,-7.75999249994725,
-0.705799923588648));
#11239=CARTESIAN_POINT('Ctrl Pts',(-0.272430079269896,-7.60038239881887,
-0.718819171731592));
#11240=CARTESIAN_POINT('Ctrl Pts',(-0.306904003698451,-7.44949161559615,
-0.726605082296128));
#11241=CARTESIAN_POINT('Ctrl Pts',(-0.306872009074495,-7.40001207497238,
-0.729157655282255));
#11242=CARTESIAN_POINT('Ctrl Pts',(-0.306892519549444,-7.39993079996377,
-0.620842344717746));
#11243=CARTESIAN_POINT('Ctrl Pts',(-0.306987690724187,-7.35368819753831,
-0.623228399614835));
#11244=CARTESIAN_POINT('Ctrl Pts',(-0.27563025645925,-7.20614417863957,
-0.630847792090333));
#11245=CARTESIAN_POINT('Ctrl Pts',(-0.0485593226474429,-7.04134574011728,
-0.643700522144239));
#11246=CARTESIAN_POINT('Ctrl Pts',(0.272358623219876,-7.16164734985291,
-0.659400534879465));
#11247=CARTESIAN_POINT('Ctrl Pts',(0.349049836864763,-7.49568337130869,
-0.675100547614689));
#11248=CARTESIAN_POINT('Ctrl Pts',(0.11274499939327,-7.74391656588417,-0.690800560349915));
#11249=CARTESIAN_POINT('Ctrl Pts',(-0.21493006795272,-7.68549648725022,
-0.706047826050934));
#11250=CARTESIAN_POINT('Ctrl Pts',(-0.307200519057126,-7.4918449102041,
-0.716061754173544));
#11251=CARTESIAN_POINT('Ctrl Pts',(-0.307744883519712,-7.39985302304706,
-0.720842344717745));
#11252=CARTESIAN_POINT('Origin',(0.,-7.4,0.220842344717745));
#11253=CARTESIAN_POINT('',(-0.307527037534926,-7.40024206511592,-0.520842344717746));
#11254=CARTESIAN_POINT('',(-0.30730322300603,-7.39973548185956,-0.529157655282254));
#11255=CARTESIAN_POINT('',(-0.30735,-7.4,0.220842344717745));
#11256=CARTESIAN_POINT('Ctrl Pts',(-0.30730322300603,-7.39973548185956,
-0.529157655282254));
#11257=CARTESIAN_POINT('Ctrl Pts',(-0.307524031931375,-7.37435491041612,
-0.530471698021893));
#11258=CARTESIAN_POINT('Ctrl Pts',(-0.293133032867834,-7.248139935795,-0.537019078339939));
#11259=CARTESIAN_POINT('Ctrl Pts',(-0.119552205895206,-7.05838870778368,
-0.548799796236395));
#11260=CARTESIAN_POINT('Ctrl Pts',(0.21898033631151,-7.11183581514136,-0.56449980897162));
#11261=CARTESIAN_POINT('Ctrl Pts',(0.361151161846345,-7.42368245147158,
-0.580199821706845));
#11262=CARTESIAN_POINT('Ctrl Pts',(0.179474171539626,-7.71429292762124,
-0.595899834442071));
#11263=CARTESIAN_POINT('Ctrl Pts',(-0.16313881982596,-7.72307367580168,
-0.611599847177296));
#11264=CARTESIAN_POINT('Ctrl Pts',(-0.301766110448845,-7.52471174942935,
-0.622685787457358));
#11265=CARTESIAN_POINT('Ctrl Pts',(-0.307762699692601,-7.41211156823841,
-0.62853839015901));
#11266=CARTESIAN_POINT('Ctrl Pts',(-0.307676170073155,-7.40018803246927,
-0.629157655282255));
#11267=CARTESIAN_POINT('Ctrl Pts',(-0.307527037534926,-7.40024206511592,
-0.520842344717745));
#11268=CARTESIAN_POINT('Ctrl Pts',(-0.306808464019153,-7.31697039411127,
-0.525161707477718));
#11269=CARTESIAN_POINT('Ctrl Pts',(-0.229186170654196,-7.13162561861014,
-0.534714407816098));
#11270=CARTESIAN_POINT('Ctrl Pts',(0.0824566476388583,-7.04759127197059,
-0.549500445732887));
#11271=CARTESIAN_POINT('Ctrl Pts',(0.3394234925214,-7.27437075694011,-0.565200458468112));
#11272=CARTESIAN_POINT('Ctrl Pts',(0.292026033272937,-7.61380320873943,
-0.580900471203338));
#11273=CARTESIAN_POINT('Ctrl Pts',(-0.0172339673348224,-7.76151623310164,
-0.596600483938563));
#11274=CARTESIAN_POINT('Ctrl Pts',(-0.266388072971644,-7.61187258080603,
-0.609914441776699));
#11275=CARTESIAN_POINT('Ctrl Pts',(-0.306778951652101,-7.4551121628007,
-0.617995062036427));
#11276=CARTESIAN_POINT('Ctrl Pts',(-0.306892519549444,-7.39993079996377,
-0.620842344717746));
#11277=CARTESIAN_POINT('Origin',(0.,-7.4,0.220842344717745));
#11278=CARTESIAN_POINT('',(-0.307468812946229,-7.39974615515026,-0.420842344717745));
#11279=CARTESIAN_POINT('',(-0.306988880358463,-7.40017554564499,-0.429157655282254));
#11280=CARTESIAN_POINT('',(-0.30735,-7.4,0.220842344717745));
#11281=CARTESIAN_POINT('Ctrl Pts',(-0.306988880358463,-7.40017554564498,
-0.429157655282254));
#11282=CARTESIAN_POINT('Ctrl Pts',(-0.306653758762801,-7.33729033837957,
-0.432405005884775));
#11283=CARTESIAN_POINT('Ctrl Pts',(-0.25747284554488,-7.17257983323238,
-0.440885694065705));
#11284=CARTESIAN_POINT('Ctrl Pts',(0.010051489927223,-7.03821281309385,
-0.454599719825043));
#11285=CARTESIAN_POINT('Ctrl Pts',(0.307303905685085,-7.20880556939548,
-0.470299732560268));
#11286=CARTESIAN_POINT('Ctrl Pts',(0.328993961842462,-7.55084420496352,
-0.485999745295494));
#11287=CARTESIAN_POINT('Ctrl Pts',(0.0556719746423119,-7.75761939660742,
-0.501699758030718));
#11288=CARTESIAN_POINT('Ctrl Pts',(-0.240517110702747,-7.65324738524168,
-0.516085728026306));
#11289=CARTESIAN_POINT('Ctrl Pts',(-0.306644633102251,-7.47543617230339,
-0.525238360443484));
#11290=CARTESIAN_POINT('Ctrl Pts',(-0.30730322300603,-7.39973548185956,
-0.529157655282254));
#11291=CARTESIAN_POINT('Ctrl Pts',(-0.307468812946229,-7.39974615515026,
-0.420842344717745));
#11292=CARTESIAN_POINT('Ctrl Pts',(-0.307642510794279,-7.38008510771902,
-0.421861677762192));
#11293=CARTESIAN_POINT('Ctrl Pts',(-0.29704048593374,-7.25966913633154,
-0.428114348385046));
#11294=CARTESIAN_POINT('Ctrl Pts',(-0.138335049048699,-7.06555355216919,
-0.43960035658631));
#11295=CARTESIAN_POINT('Ctrl Pts',(0.202642850697595,-7.1001218792852,-0.455300369321535));
#11296=CARTESIAN_POINT('Ctrl Pts',(0.361908962168568,-7.40359379400104,
-0.47100038205676));
#11297=CARTESIAN_POINT('Ctrl Pts',(0.196647835235759,-7.70384311944753,
-0.486700394791986));
#11298=CARTESIAN_POINT('Ctrl Pts',(-0.144949292044521,-7.73163340416662,
-0.502400407527211));
#11299=CARTESIAN_POINT('Ctrl Pts',(-0.298348518520842,-7.53621361726224,
-0.513781057502464));
#11300=CARTESIAN_POINT('Ctrl Pts',(-0.307679087301317,-7.41786230555802,
-0.519928369899309));
#11301=CARTESIAN_POINT('Ctrl Pts',(-0.307527037534926,-7.40024206511592,
-0.520842344717745));
#11302=CARTESIAN_POINT('Origin',(0.,-7.4,0.220842344717745));
#11303=CARTESIAN_POINT('',(-0.306909613402721,-7.40009950835258,-0.320842344717745));
#11304=CARTESIAN_POINT('',(-0.307834831763841,-7.40001803034581,-0.329157655282254));
#11305=CARTESIAN_POINT('',(-0.30735,-7.4,0.220842344717745));
#11306=CARTESIAN_POINT('Ctrl Pts',(-0.307834831763841,-7.40001803034581,
-0.329157655282254));
#11307=CARTESIAN_POINT('Ctrl Pts',(-0.307748387795955,-7.3004045226342,
-0.334338313747658));
#11308=CARTESIAN_POINT('Ctrl Pts',(-0.201498740191458,-7.10000590319923,
-0.34475230979147));
#11309=CARTESIAN_POINT('Ctrl Pts',(0.13833504309277,-7.06555356656853,-0.36039964341369));
#11310=CARTESIAN_POINT('Ctrl Pts',(0.355266567892898,-7.33088656640977,
-0.376099656148916));
#11311=CARTESIAN_POINT('Ctrl Pts',(0.253627152997932,-7.65819424514732,
-0.391799668884141));
#11312=CARTESIAN_POINT('Ctrl Pts',(-0.0754421632001089,-7.75397666730194,
-0.407499681619367));
#11313=CARTESIAN_POINT('Ctrl Pts',(-0.282790403389065,-7.57818658295138,
-0.419952343752071));
#11314=CARTESIAN_POINT('Ctrl Pts',(-0.307193831164762,-7.43863434418313,
-0.427171668306367));
#11315=CARTESIAN_POINT('Ctrl Pts',(-0.306988880358463,-7.40017554564498,
-0.429157655282254));
#11316=CARTESIAN_POINT('Ctrl Pts',(-0.306909613402721,-7.40009950835258,
-0.320842344717745));
#11317=CARTESIAN_POINT('Ctrl Pts',(-0.30673964456656,-7.3428842629932,-0.323794985625074));
#11318=CARTESIAN_POINT('Ctrl Pts',(-0.264122895071672,-7.18402403042701,
-0.331980964110812));
#11319=CARTESIAN_POINT('Ctrl Pts',(-0.0100514903598289,-7.03821279751757,
-0.345400280174958));
#11320=CARTESIAN_POINT('Ctrl Pts',(0.296214206411665,-7.19203808960976,
-0.361100292910183));
#11321=CARTESIAN_POINT('Ctrl Pts',(0.336861782355269,-7.53234482162411,
-0.376800305645408));
#11322=CARTESIAN_POINT('Ctrl Pts',(0.0754421664482044,-7.75397668254217,
-0.392500318380634));
#11323=CARTESIAN_POINT('Ctrl Pts',(-0.232262133964356,-7.66441298957495,
-0.407180998071413));
#11324=CARTESIAN_POINT('Ctrl Pts',(-0.306750732115625,-7.4810265016171,
-0.416628340183783));
#11325=CARTESIAN_POINT('Ctrl Pts',(-0.307468812946229,-7.39974615515026,
-0.420842344717745));
#11326=CARTESIAN_POINT('Origin',(0.,-7.4,0.220842344717745));
#11327=CARTESIAN_POINT('',(-0.30778047748176,-7.40011439329532,-0.220842344717745));
#11328=CARTESIAN_POINT('',(-0.307027521263749,-7.39980163161079,-0.229157655282254));
#11329=CARTESIAN_POINT('',(-0.30735,-7.4,0.220842344717745));
#11330=CARTESIAN_POINT('Ctrl Pts',(-0.307027521263749,-7.39980163161079,
-0.229157655282254));
#11331=CARTESIAN_POINT('Ctrl Pts',(-0.30724864923996,-7.36339464766693,
-0.231038284032132));
#11332=CARTESIAN_POINT('Ctrl Pts',(-0.284548683414164,-7.22594242273193,
-0.238152250360418));
#11333=CARTESIAN_POINT('Ctrl Pts',(-0.0824566440890477,-7.04759128714739,
-0.250499554267113));
#11334=CARTESIAN_POINT('Ctrl Pts',(0.248449852494269,-7.13682007602022,
-0.266199567002339));
#11335=CARTESIAN_POINT('Ctrl Pts',(0.356568983342811,-7.46204483232109,
-0.281899579737564));
#11336=CARTESIAN_POINT('Ctrl Pts',(0.144949285803845,-7.73163338988777,
-0.297599592472789));
#11337=CARTESIAN_POINT('Ctrl Pts',(-0.196647826769216,-7.70384310636604,
-0.313299605208015));
#11338=CARTESIAN_POINT('Ctrl Pts',(-0.30737641633832,-7.50266945504914,
-0.323818959477836));
#11339=CARTESIAN_POINT('Ctrl Pts',(-0.307835710762444,-7.40103094236551,
-0.329104976169249));
#11340=CARTESIAN_POINT('Ctrl Pts',(-0.307834831763841,-7.40001803034581,
-0.329157655282254));
#11341=CARTESIAN_POINT('Ctrl Pts',(-0.30778047748176,-7.40011439329532,
-0.220842344717745));
#11342=CARTESIAN_POINT('Ctrl Pts',(-0.307325164697339,-7.3061230854425,
-0.225728293487957));
#11343=CARTESIAN_POINT('Ctrl Pts',(-0.211489751737109,-7.11065319680823,
-0.235847579836577));
#11344=CARTESIAN_POINT('Ctrl Pts',(0.119552211049655,-7.05838869308885,
-0.251200203763606));
#11345=CARTESIAN_POINT('Ctrl Pts',(0.350881178877997,-7.31126774940073,
-0.266900216498831));
#11346=CARTESIAN_POINT('Ctrl Pts',(0.267571614711511,-7.64371385133353,
-0.282600229234056));
#11347=CARTESIAN_POINT('Ctrl Pts',(-0.0556719770403169,-7.75761941200269,
-0.298300241969282));
#11348=CARTESIAN_POINT('Ctrl Pts',(-0.277591360694641,-7.58973162677787,
-0.311047613797178));
#11349=CARTESIAN_POINT('Ctrl Pts',(-0.307040901754737,-7.44429405273561,
-0.318561648046666));
#11350=CARTESIAN_POINT('Ctrl Pts',(-0.306909613402721,-7.40009950835258,
-0.320842344717745));
#11351=CARTESIAN_POINT('Origin',(0.,-7.4,0.220842344717745));
#11352=CARTESIAN_POINT('',(-0.307159064170147,-7.39975436132604,-0.120842344717745));
#11353=CARTESIAN_POINT('',(-0.307245641089215,-7.40026066578654,-0.129157655282254));
#11354=CARTESIAN_POINT('',(-0.30735,-7.4,0.220842344717745));
#11355=CARTESIAN_POINT('Ctrl Pts',(-0.307245641089215,-7.40026066578654,
-0.129157655282254));
#11356=CARTESIAN_POINT('Ctrl Pts',(-0.306624848470386,-7.32655967317157,
-0.132971591895015));
#11357=CARTESIAN_POINT('Ctrl Pts',(-0.24334518130105,-7.15077117668026,
-0.142018866086184));
#11358=CARTESIAN_POINT('Ctrl Pts',(0.0485593205265976,-7.04134575574766,
-0.156299477855761));
#11359=CARTESIAN_POINT('Ctrl Pts',(0.32593357368315,-7.24265220640667,-0.171999490590986));
#11360=CARTESIAN_POINT('Ctrl Pts',(0.311040099268243,-7.58505425382268,
-0.187699503326212));
#11361=CARTESIAN_POINT('Ctrl Pts',(0.017233966595936,-7.7615162175086,-0.203399516061437));
#11362=CARTESIAN_POINT('Ctrl Pts',(-0.25498125945776,-7.63149702903767,
-0.217218900046785));
#11363=CARTESIAN_POINT('Ctrl Pts',(-0.306633303256541,-7.46470652923967,
-0.225804946453724));
#11364=CARTESIAN_POINT('Ctrl Pts',(-0.307027521263749,-7.39980163161079,
-0.229157655282254));
#11365=CARTESIAN_POINT('Ctrl Pts',(-0.307159064170147,-7.39975436132604,
-0.120842344717745));
#11366=CARTESIAN_POINT('Ctrl Pts',(-0.307397703183449,-7.3690856088527,
-0.122428263772431));
#11367=CARTESIAN_POINT('Ctrl Pts',(-0.289195399760154,-7.23749021428436,
-0.129247520405525));
#11368=CARTESIAN_POINT('Ctrl Pts',(-0.101895244140074,-7.05271424100694,
-0.141300114617028));
#11369=CARTESIAN_POINT('Ctrl Pts',(0.233453617301762,-7.1234308319262,-0.157000127352253));
#11370=CARTESIAN_POINT('Ctrl Pts',(0.359464106016436,-7.44215165429935,
-0.172700140087479));
#11371=CARTESIAN_POINT('Ctrl Pts',(0.163138826931865,-7.72307368988404,
-0.188400152822704));
#11372=CARTESIAN_POINT('Ctrl Pts',(-0.179474179312067,-7.714292941062,-0.204100165557929));
#11373=CARTESIAN_POINT('Ctrl Pts',(-0.304612082771875,-7.51412237656679,
-0.214914229522943));
#11374=CARTESIAN_POINT('Ctrl Pts',(-0.307812850020437,-7.40679713393618,
-0.220494955909548));
#11375=CARTESIAN_POINT('Ctrl Pts',(-0.30778047748176,-7.40011439329532,
-0.220842344717745));
#11376=CARTESIAN_POINT('Origin',(0.,-7.4,0.220842344717745));
#11377=CARTESIAN_POINT('',(-0.307019775097118,-7.40030626975107,-0.0208423447177452));
#11378=CARTESIAN_POINT('',(-0.307720604786163,-7.39984568899361,-0.0291576552822545));
#11379=CARTESIAN_POINT('',(-0.30735,-7.4,0.220842344717745));
#11380=CARTESIAN_POINT('',(-0.0793799282532844,-7.69692229537457,0.));
#11381=CARTESIAN_POINT('Ctrl Pts',(-0.0793799282532839,-7.69692229537457,
2.77555756156289E-17));
#11382=CARTESIAN_POINT('Ctrl Pts',(-0.177014005842305,-7.67082056372685,
-0.00523333757840842));
#11383=CARTESIAN_POINT('Ctrl Pts',(-0.287143401920737,-7.56754973948506,
-0.0121807858176568));
#11384=CARTESIAN_POINT('Ctrl Pts',(-0.307246217690486,-7.43347295261345,
-0.0191282340569052));
#11385=CARTESIAN_POINT('Ctrl Pts',(-0.307019775097118,-7.40030626975107,
-0.0208423447177452));
#11386=CARTESIAN_POINT('',(0.0795799710354742,-7.69739806084557,-1.93091915593928E-16));
#11387=CARTESIAN_POINT('Origin',(0.,-7.4,0.));
#11388=CARTESIAN_POINT('Ctrl Pts',(0.0795809081573368,-7.69740028961993,
2.49366499671666E-17));
#11389=CARTESIAN_POINT('Ctrl Pts',(-0.0133964972572649,-7.72194966690666,
-0.00499978774624427));
#11390=CARTESIAN_POINT('Ctrl Pts',(-0.21902209759443,-7.67864022412054,
-0.0147190061736624));
#11391=CARTESIAN_POINT('Ctrl Pts',(-0.307135787948618,-7.49066305702376,
-0.0244382246010806));
#11392=CARTESIAN_POINT('Ctrl Pts',(-0.307720604786163,-7.39984568899361,
-0.0291576552822545));
#11393=CARTESIAN_POINT('Origin',(0.,0.,0.));
#11394=CARTESIAN_POINT('',(-6.35,-7.77650717458569E-16,0.));
#11395=CARTESIAN_POINT('Origin',(0.,0.,0.));
#11396=CARTESIAN_POINT('',(-6.35,-7.77650717458569E-16,-0.2));
#11397=CARTESIAN_POINT('',(-6.35,7.77650717458569E-16,0.));
#11398=CARTESIAN_POINT('Origin',(0.,0.,-0.2));
#11399=CARTESIAN_POINT('Origin',(0.,0.,0.));
#11400=CARTESIAN_POINT('',(-6.85,-8.38883057415937E-16,0.));
#11401=CARTESIAN_POINT('Origin',(0.,0.,0.));
#11402=CARTESIAN_POINT('',(-6.85,-8.38883057415937E-16,-0.2));
#11403=CARTESIAN_POINT('',(-6.85,8.38883057415937E-16,0.));
#11404=CARTESIAN_POINT('Origin',(0.,0.,-0.2));
#11405=CARTESIAN_POINT('Origin',(0.,0.,-0.2));
#11406=CARTESIAN_POINT('Origin',(0.,0.,0.));
#11407=CARTESIAN_POINT('',(-1.68151315379565,-2.11246621596943,0.));
#11408=CARTESIAN_POINT('',(-2.7,-3.30654635769785E-16,0.));
#11409=CARTESIAN_POINT('Origin',(0.,0.,0.));
#11410=CARTESIAN_POINT('',(-1.68151315379564,2.11246621596944,0.));
#11411=CARTESIAN_POINT('Origin',(0.,0.,0.));
#11412=CARTESIAN_POINT('',(-1.37718656791819,1.58535710713571,1.11022302462516E-16));
#11413=CARTESIAN_POINT('',(-1.89641016151378,2.48467875173176,0.));
#11414=CARTESIAN_POINT('',(-1.37718656791819,-1.58535710713571,0.));
#11415=CARTESIAN_POINT('Origin',(0.,0.,0.));
#11416=CARTESIAN_POINT('',(-1.29641016151378,-1.44544826719043,0.));
#11417=CARTESIAN_POINT('',(-0.988692830768093,2.51246621596944,0.));
#11418=CARTESIAN_POINT('',(2.67020598456374,0.4,0.));
#11419=CARTESIAN_POINT('Origin',(0.,0.,0.));
#11420=CARTESIAN_POINT('',(2.06155281280883,0.4,0.));
#11421=CARTESIAN_POINT('',(3.1,0.4,0.));
#11422=CARTESIAN_POINT('',(-0.684366244890639,1.98535710713571,1.11022302462516E-16));
#11423=CARTESIAN_POINT('Origin',(0.,0.,0.));
#11424=CARTESIAN_POINT('',(-0.603589838486224,1.84544826719043,0.));
#11425=CARTESIAN_POINT('',(-0.988692830768095,-2.51246621596944,0.));
#11426=CARTESIAN_POINT('',(-0.684366244890641,-1.98535710713571,0.));
#11427=CARTESIAN_POINT('',(-1.20358983848623,-2.88467875173176,0.));
#11428=CARTESIAN_POINT('',(2.06155281280883,-0.4,0.));
#11429=CARTESIAN_POINT('Origin',(0.,0.,0.));
#11430=CARTESIAN_POINT('',(2.67020598456374,-0.4,0.));
#11431=CARTESIAN_POINT('',(1.9,-0.4,0.));
#11432=CARTESIAN_POINT('Origin',(0.,0.,0.));
#11433=CARTESIAN_POINT('',(-1.7,-2.0818995585505E-16,0.));
#11434=CARTESIAN_POINT('Origin',(0.,0.,0.));
#11435=CARTESIAN_POINT('Origin',(0.,-7.4,0.220842344717745));
#11436=CARTESIAN_POINT('Ctrl Pts',(-0.307720604786163,-7.39984568899361,
-0.0291576552822545));
#11437=CARTESIAN_POINT('Ctrl Pts',(-0.307784286494135,-7.38995643010364,
-0.0296715621794891));
#11438=CARTESIAN_POINT('Ctrl Pts',(-0.302900314845739,-7.27942155055893,
-0.0354188066551321));
#11439=CARTESIAN_POINT('Ctrl Pts',(-0.169525086729888,-7.08020524373302,
-0.0463993887091836));
#11440=CARTESIAN_POINT('Ctrl Pts',(0.1731988395346,-7.0822171223069,-0.0620994014444089));
#11441=CARTESIAN_POINT('Ctrl Pts',(0.360608974721706,-7.3691443808669,-0.0777994141796343));
#11442=CARTESIAN_POINT('Ctrl Pts',(0.224659927796838,-7.6837617716103,-0.0934994269148595));
#11443=CARTESIAN_POINT('Ctrl Pts',(-0.112744994253697,-7.74391654987674,
-0.109199439650085));
#11444=CARTESIAN_POINT('Ctrl Pts',(-0.291645305847843,-7.55598558781012,
-0.12108551577255));
#11445=CARTESIAN_POINT('Ctrl Pts',(-0.307476676298265,-7.42768934924628,
-0.127738254316606));
#11446=CARTESIAN_POINT('Ctrl Pts',(-0.307245641089215,-7.40026066578654,
-0.129157655282254));
#11447=CARTESIAN_POINT('Ctrl Pts',(-0.307019775097118,-7.40030626975107,
-0.0208423447177452));
#11448=CARTESIAN_POINT('Ctrl Pts',(-0.306554867615898,-7.33221201786739,
-0.0243615716353137));
#11449=CARTESIAN_POINT('Ctrl Pts',(-0.25102806371146,-7.16194939514258,
-0.0331141361312906));
#11450=CARTESIAN_POINT('Ctrl Pts',(0.0286357521188298,-7.03927813304723,
-0.047100038205676));
#11451=CARTESIAN_POINT('Ctrl Pts',(0.31666225793602,-7.22476085896309,-0.0628000509409014));
#11452=CARTESIAN_POINT('Ctrl Pts',(0.320850989126134,-7.56751742991046,
-0.0785000636761266));
#11453=CARTESIAN_POINT('Ctrl Pts',(0.0372719144191142,-7.75999252270946,
-0.0942000764113521));
#11454=CARTESIAN_POINT('Ctrl Pts',(-0.247682040721021,-7.64285422545096,
-0.108314170091892));
#11455=CARTESIAN_POINT('Ctrl Pts',(-0.306610223827363,-7.4702887152328,
-0.117194926194023));
#11456=CARTESIAN_POINT('Ctrl Pts',(-0.307159064170147,-7.39975436132604,
-0.120842344717745));
#11457=CARTESIAN_POINT('Ctrl Pts',(0.191346599666505,-7.2364012796625,0.));
#11458=CARTESIAN_POINT('Ctrl Pts',(0.245141179607852,-7.29931992554818,
-0.00523333757840845));
#11459=CARTESIAN_POINT('Ctrl Pts',(0.284951729745964,-7.48132135155768,
-0.0157000127352253));
#11460=CARTESIAN_POINT('Ctrl Pts',(0.0891127727595961,-7.6829132685142,
-0.0314000254704507));
#11461=CARTESIAN_POINT('Ctrl Pts',(-0.186694378247,-7.63020857787028,-0.047100038205676));
#11462=CARTESIAN_POINT('Ctrl Pts',(-0.295059602684748,-7.37136782429952,
-0.0628000509409014));
#11463=CARTESIAN_POINT('Ctrl Pts',(-0.138857786185943,-7.13805651573056,
-0.0785000636761267));
#11464=CARTESIAN_POINT('Ctrl Pts',(0.141866952506379,-7.13970444295027,
-0.0942000764113521));
#11465=CARTESIAN_POINT('Ctrl Pts',(0.295374359480038,-7.37472620101916,
-0.109900089146577));
#11466=CARTESIAN_POINT('Ctrl Pts',(0.184018665439577,-7.63242891167365,
-0.125600101881803));
#11467=CARTESIAN_POINT('Ctrl Pts',(-0.0923492835639111,-7.68170161519918,
-0.141300114617028));
#11468=CARTESIAN_POINT('Ctrl Pts',(-0.285906271942125,-7.47837412674206,
-0.157000127352253));
#11469=CARTESIAN_POINT('Ctrl Pts',(-0.223088597453814,-7.20476565095269,
-0.172700140087479));
#11470=CARTESIAN_POINT('Ctrl Pts',(0.0397748786158152,-7.10622675779884,
-0.188400152822704));
#11471=CARTESIAN_POINT('Ctrl Pts',(0.266971781925274,-7.2711166193684,-0.20410016555793));
#11472=CARTESIAN_POINT('Ctrl Pts',(0.254772555688239,-7.55157770749914,
-0.219800178293155));
#11473=CARTESIAN_POINT('Ctrl Pts',(0.0141163204507142,-7.69611748091033,
-0.23550019102838));
#11474=CARTESIAN_POINT('Ctrl Pts',(-0.239198147751981,-7.57512593293145,
-0.251200203763606));
#11475=CARTESIAN_POINT('Ctrl Pts',(-0.27802134557703,-7.29709724880236,
-0.266900216498831));
#11476=CARTESIAN_POINT('Ctrl Pts',(-0.0675401338845549,-7.11134246474494,
-0.282600229234056));
#11477=CARTESIAN_POINT('Ctrl Pts',(0.203504962958946,-7.18442965393879,
-0.298300241969281));
#11478=CARTESIAN_POINT('Ctrl Pts',(0.292065207602253,-7.45082084443414,
-0.314000254704507));
#11479=CARTESIAN_POINT('Ctrl Pts',(0.11872777843214,-7.67164049423864,-0.329700267439732));
#11480=CARTESIAN_POINT('Ctrl Pts',(-0.161073988577029,-7.64887750781731,
-0.345400280174958));
#11481=CARTESIAN_POINT('Ctrl Pts',(-0.296439164806322,-7.40294367203764,
-0.361100292910183));
#11482=CARTESIAN_POINT('Ctrl Pts',(-0.165984498020776,-7.15437021753843,
-0.376800305645409));
#11483=CARTESIAN_POINT('Ctrl Pts',(0.113310060512786,-7.12605534531845,
-0.392500318380633));
#11484=CARTESIAN_POINT('Ctrl Pts',(0.290998400738692,-7.34338927312074,
-0.408200331115859));
#11485=CARTESIAN_POINT('Ctrl Pts',(0.207745683316185,-7.61148658277481,
-0.423900343851084));
#11486=CARTESIAN_POINT('Ctrl Pts',(-0.0617945813750686,-7.68994184478043,
-0.439600356586309));
#11487=CARTESIAN_POINT('Ctrl Pts',(-0.275923052079717,-7.50840347294413,
-0.455300369321535));
#11488=CARTESIAN_POINT('Ctrl Pts',(-0.242628674974808,-7.22965866703555,
-0.47100038205676));
#11489=CARTESIAN_POINT('Ctrl Pts',(0.00823316280845383,-7.10366056839557,
-0.486700394791985));
#11490=CARTESIAN_POINT('Ctrl Pts',(0.251712244204393,-7.2433928813903,-0.502400407527211));
#11491=CARTESIAN_POINT('Ctrl Pts',(0.269478542032991,-7.52355629933161,
-0.518100420262436));
#11492=CARTESIAN_POINT('Ctrl Pts',(0.0456008446923772,-7.6929255997915,
-0.533800432997662));
#11493=CARTESIAN_POINT('Ctrl Pts',(-0.21916756500053,-7.59962570174306,
-0.549500445732887));
#11494=CARTESIAN_POINT('Ctrl Pts',(-0.287406321718959,-7.32731952781878,
-0.565200458468112));
#11495=CARTESIAN_POINT('Ctrl Pts',(-0.097925062092462,-7.12018661846282,
-0.580900471203338));
#11496=CARTESIAN_POINT('Ctrl Pts',(0.179366519168448,-7.16396507714928,
-0.596600483938563));
#11497=CARTESIAN_POINT('Ctrl Pts',(0.295818464274662,-7.41939826633471,
-0.612300496673789));
#11498=CARTESIAN_POINT('Ctrl Pts',(0.147007069090942,-7.65743694331754,
-0.628000509409014));
#11499=CARTESIAN_POINT('Ctrl Pts',(-0.13362680296465,-7.66462924315299,
-0.643700522144239));
#11500=CARTESIAN_POINT('Ctrl Pts',(-0.294436586401099,-7.43452636601645,
-0.659400534879464));
#11501=CARTESIAN_POINT('Ctrl Pts',(-0.191221557053218,-7.17346255012345,
-0.675100547614691));
#11502=CARTESIAN_POINT('Ctrl Pts',(0.0834622628790381,-7.11553868302403,
-0.690800560349915));
#11503=CARTESIAN_POINT('Ctrl Pts',(0.28330752343249,-7.31269069134103,-0.706500573085141));
#11504=CARTESIAN_POINT('Ctrl Pts',(0.229102456085247,-7.58814048413055,
-0.722200585820366));
#11505=CARTESIAN_POINT('Ctrl Pts',(-0.0305293756465861,-7.6948694057645,
-0.737900598555591));
#11506=CARTESIAN_POINT('Ctrl Pts',(-0.26280863385947,-7.53721332189184,
-0.753600611290817));
#11507=CARTESIAN_POINT('Ctrl Pts',(-0.25937764590646,-7.25646182589342,
-0.769300624026042));
#11508=CARTESIAN_POINT('Ctrl Pts',(-0.0234555070157643,-7.10453321779813,
-0.785000636761267));
#11509=CARTESIAN_POINT('Ctrl Pts',(0.233691827601142,-7.21732779772848,
-0.800700649496493));
#11510=CARTESIAN_POINT('Ctrl Pts',(0.280893064283751,-7.49439140290128,
-0.816400662231719));
#11511=CARTESIAN_POINT('Ctrl Pts',(0.144991950449976,-7.62182878450703,
-0.826867337388535));
#11512=CARTESIAN_POINT('Ctrl Pts',(0.0650199997975086,-7.64320868020351,
-0.832100674966944));
#11513=CARTESIAN_POINT('Ctrl Pts',(0.205433155034208,-7.22435746787732,
0.0107002249889811));
#11514=CARTESIAN_POINT('Ctrl Pts',(0.263187984753429,-7.291908059094,0.00546688741057261));
#11515=CARTESIAN_POINT('Ctrl Pts',(0.305929308261523,-7.48730806740887,
-0.00499978774624425));
#11516=CARTESIAN_POINT('Ctrl Pts',(0.0956730775135631,-7.70374077957594,
-0.0206998004814697));
#11517=CARTESIAN_POINT('Ctrl Pts',(-0.200438446344363,-7.64715607463241,
-0.0363998132166949));
#11518=CARTESIAN_POINT('Ctrl Pts',(-0.316781302663923,-7.36925998058027,
-0.0520998259519204));
#11519=CARTESIAN_POINT('Ctrl Pts',(-0.149080219700592,-7.11877275839805,
-0.0677998386871456));
#11520=CARTESIAN_POINT('Ctrl Pts',(0.152310914849119,-7.12054200273581,
-0.0834998514223711));
#11521=CARTESIAN_POINT('Ctrl Pts',(0.31711923122726,-7.37286559430175,-0.0991998641575963));
#11522=CARTESIAN_POINT('Ctrl Pts',(0.197565752891998,-7.64953986498586,
-0.114899876892822));
#11523=CARTESIAN_POINT('Ctrl Pts',(-0.0991478537938397,-7.70243992675837,
-0.130599889628047));
#11524=CARTESIAN_POINT('Ctrl Pts',(-0.306954121952032,-7.48414387377529,
-0.146299902363272));
#11525=CARTESIAN_POINT('Ctrl Pts',(-0.23951193544578,-7.19039288722277,
-0.161999915098498));
#11526=CARTESIAN_POINT('Ctrl Pts',(0.0427030259194093,-7.08459975711512,
-0.177699927833723));
#11527=CARTESIAN_POINT('Ctrl Pts',(0.286625712511232,-7.26162848171449,
-0.193399940568948));
#11528=CARTESIAN_POINT('Ctrl Pts',(0.273528403548241,-7.56273655627365,
-0.209099953304174));
#11529=CARTESIAN_POINT('Ctrl Pts',(0.0151555358324549,-7.71791705977642,
-0.224799966039399));
#11530=CARTESIAN_POINT('Ctrl Pts',(-0.256807438735113,-7.58801835513732,
-0.240499978774624));
#11531=CARTESIAN_POINT('Ctrl Pts',(-0.29848872302037,-7.28952175331532,
-0.25619999150985));
#11532=CARTESIAN_POINT('Ctrl Pts',(-0.0725123039527193,-7.09009207221242,
-0.271900004245075));
#11533=CARTESIAN_POINT('Ctrl Pts',(0.218486592804054,-7.1685597946326,-0.287600016980301));
#11534=CARTESIAN_POINT('Ctrl Pts',(0.313566466182439,-7.45456217372979,
-0.303300029715526));
#11535=CARTESIAN_POINT('Ctrl Pts',(0.127468280889375,-7.69163812612169,
-0.319000042450751));
#11536=CARTESIAN_POINT('Ctrl Pts',(-0.172931934641091,-7.66719937400022,
-0.334700055185977));
#11537=CARTESIAN_POINT('Ctrl Pts',(-0.31826242539981,-7.40316037930715,
-0.350400067921202));
#11538=CARTESIAN_POINT('Ctrl Pts',(-0.178203946004828,-7.13628744242441,
-0.366100080656428));
#11539=CARTESIAN_POINT('Ctrl Pts',(0.12165172137278,-7.10588808573515,-0.381800093391652));
#11540=CARTESIAN_POINT('Ctrl Pts',(0.312421123123427,-7.33922170421708,
-0.397500106126878));
#11541=CARTESIAN_POINT('Ctrl Pts',(0.223039506543434,-7.62705580356564,
-0.413200118862103));
#11542=CARTESIAN_POINT('Ctrl Pts',(-0.0663437753167488,-7.71128678562093,
-0.428900131597329));
#11543=CARTESIAN_POINT('Ctrl Pts',(-0.296235957337091,-7.51638392060476,
-0.444600144332554));
#11544=CARTESIAN_POINT('Ctrl Pts',(-0.260490514536012,-7.21711847754488,
-0.460300157067779));
#11545=CARTESIAN_POINT('Ctrl Pts',(0.0088392718480435,-7.08184464996167,
-0.476000169803005));
#11546=CARTESIAN_POINT('Ctrl Pts',(0.27024279803129,-7.23186377739202,-0.49170018253823));
#11547=CARTESIAN_POINT('Ctrl Pts',(0.289317015302814,-7.53265226787559,
-0.507400195273456));
#11548=CARTESIAN_POINT('Ctrl Pts',(0.0489578880090222,-7.71449019873013,
-0.52310020800868));
#11549=CARTESIAN_POINT('Ctrl Pts',(-0.235302244396795,-7.61432174810773,
-0.538800220743907));
#11550=CARTESIAN_POINT('Ctrl Pts',(-0.308564602404261,-7.32196893628847,
-0.554500233479131));
#11551=CARTESIAN_POINT('Ctrl Pts',(-0.10513411002671,-7.0995873149031,-0.570200246214357));
#11552=CARTESIAN_POINT('Ctrl Pts',(0.192571124882802,-7.14658865647997,
-0.585900258949582));
#11553=CARTESIAN_POINT('Ctrl Pts',(0.317596030131889,-7.42082632804701,
-0.601600271684808));
#11554=CARTESIAN_POINT('Ctrl Pts',(0.157829436573836,-7.67638893808543,
-0.617300284420033));
#11555=CARTESIAN_POINT('Ctrl Pts',(-0.14346414191842,-7.68411072070256,
-0.633000297155258));
#11556=CARTESIAN_POINT('Ctrl Pts',(-0.316112421162968,-7.43706812828128,
-0.648700309890484));
#11557=CARTESIAN_POINT('Ctrl Pts',(-0.205298907032905,-7.15678531448872,
-0.664400322625708));
#11558=CARTESIAN_POINT('Ctrl Pts',(0.0896065883554691,-7.09459720771934,
-0.680100335360935));
#11559=CARTESIAN_POINT('Ctrl Pts',(0.30416405875569,-7.30626315402036,-0.69580034809616));
#11560=CARTESIAN_POINT('Ctrl Pts',(0.245968522365736,-7.60199101166138,
-0.711500360831385));
#11561=CARTESIAN_POINT('Ctrl Pts',(-0.0327768874452623,-7.71657710382541,
-0.72720037356661));
#11562=CARTESIAN_POINT('Ctrl Pts',(-0.282156081780803,-7.54731469322211,
-0.742900386301835));
#11563=CARTESIAN_POINT('Ctrl Pts',(-0.278472511331682,-7.24589483154675,
-0.758600399037061));
#11564=CARTESIAN_POINT('Ctrl Pts',(-0.025182254702062,-7.0827815420743,
-0.774300411772286));
#11565=CARTESIAN_POINT('Ctrl Pts',(0.25089575426731,-7.20387983421137,-0.790000424507512));
#11566=CARTESIAN_POINT('Ctrl Pts',(0.301571851935755,-7.50134030988745,
-0.805700437242737));
#11567=CARTESIAN_POINT('Ctrl Pts',(0.155665968914086,-7.6381593775803,-0.816167112399554));
#11568=CARTESIAN_POINT('Ctrl Pts',(0.0698066426161003,-7.66111321859386,
-0.821400449977962));
#11569=CARTESIAN_POINT('Ctrl Pts',(0.219519710401911,-7.21231365609212,
0.0214004499779621));
#11570=CARTESIAN_POINT('Ctrl Pts',(0.281234789899005,-7.28449619263982,
0.0161671123995537));
#11571=CARTESIAN_POINT('Ctrl Pts',(0.326906886777081,-7.49329478326005,
0.0057004372427368));
#11572=CARTESIAN_POINT('Ctrl Pts',(0.10223338226753,-7.7245682906377,-0.00999957549248859));
#11573=CARTESIAN_POINT('Ctrl Pts',(-0.214182514441725,-7.66410357139452,
-0.0256995882277139));
#11574=CARTESIAN_POINT('Ctrl Pts',(-0.338503002643098,-7.36715213686105,
-0.0413996009629393));
#11575=CARTESIAN_POINT('Ctrl Pts',(-0.15930265321524,-7.09948900106554,
-0.0570996136981646));
#11576=CARTESIAN_POINT('Ctrl Pts',(0.162754877191859,-7.10137956252136,
-0.07279962643339));
#11577=CARTESIAN_POINT('Ctrl Pts',(0.338864102974484,-7.37100498758432,
-0.0884996391686153));
#11578=CARTESIAN_POINT('Ctrl Pts',(0.211112840344417,-7.66665081829808,
-0.104199651903841));
#11579=CARTESIAN_POINT('Ctrl Pts',(-0.105946424023768,-7.72317823831756,
-0.119899664639066));
#11580=CARTESIAN_POINT('Ctrl Pts',(-0.328001971961939,-7.48991362080854,
-0.135599677374291));
#11581=CARTESIAN_POINT('Ctrl Pts',(-0.255935273437745,-7.17602012349283,
-0.151299690109517));
#11582=CARTESIAN_POINT('Ctrl Pts',(0.0456311732230033,-7.06297275643139,
-0.166999702844742));
#11583=CARTESIAN_POINT('Ctrl Pts',(0.306279643097191,-7.25214034406058,
-0.182699715579967));
#11584=CARTESIAN_POINT('Ctrl Pts',(0.292284251408242,-7.57389540504817,
-0.198399728315193));
#11585=CARTESIAN_POINT('Ctrl Pts',(0.0161947512141955,-7.7397166386425,
-0.214099741050418));
#11586=CARTESIAN_POINT('Ctrl Pts',(-0.274416729718245,-7.60091077734321,
-0.229799753785643));
#11587=CARTESIAN_POINT('Ctrl Pts',(-0.31895610046371,-7.28194625782827,
-0.245499766520869));
#11588=CARTESIAN_POINT('Ctrl Pts',(-0.0774844740208837,-7.06884167967991,
-0.261199779256094));
#11589=CARTESIAN_POINT('Ctrl Pts',(0.233468222649161,-7.15268993532641,
-0.27689979199132));
#11590=CARTESIAN_POINT('Ctrl Pts',(0.335067724762625,-7.45830350302544,
-0.292599804726544));
#11591=CARTESIAN_POINT('Ctrl Pts',(0.13620878334661,-7.71163575800473,-0.308299817461771));
#11592=CARTESIAN_POINT('Ctrl Pts',(-0.184789880705154,-7.68552124018313,
-0.323999830196995));
#11593=CARTESIAN_POINT('Ctrl Pts',(-0.340085685993297,-7.40337708657666,
-0.339699842932221));
#11594=CARTESIAN_POINT('Ctrl Pts',(-0.19042339398888,-7.11820466731038,
-0.355399855667446));
#11595=CARTESIAN_POINT('Ctrl Pts',(0.129993382232775,-7.08572082615184,
-0.371099868402671));
#11596=CARTESIAN_POINT('Ctrl Pts',(0.333843845508162,-7.33505413531342,
-0.386799881137897));
#11597=CARTESIAN_POINT('Ctrl Pts',(0.238333329770683,-7.64262502435649,
-0.402499893873123));
#11598=CARTESIAN_POINT('Ctrl Pts',(-0.070892969258429,-7.73263172646143,
-0.418199906608347));
#11599=CARTESIAN_POINT('Ctrl Pts',(-0.316548862594466,-7.52436436826539,
-0.433899919343574));
#11600=CARTESIAN_POINT('Ctrl Pts',(-0.278352354097216,-7.20457828805423,
-0.449599932078798));
#11601=CARTESIAN_POINT('Ctrl Pts',(0.00944538088763332,-7.06002873152775,
-0.465299944814024));
#11602=CARTESIAN_POINT('Ctrl Pts',(0.288773351858187,-7.22033467339375,
-0.480999957549248));
#11603=CARTESIAN_POINT('Ctrl Pts',(0.309155488572638,-7.54174823641955,
-0.496699970284475));
#11604=CARTESIAN_POINT('Ctrl Pts',(0.052314931325667,-7.73605479766878,
-0.512399983019699));
#11605=CARTESIAN_POINT('Ctrl Pts',(-0.251436923793061,-7.62901779447239,
-0.528099995754926));
#11606=CARTESIAN_POINT('Ctrl Pts',(-0.329722883089562,-7.31661834475815,
-0.54380000849015));
#11607=CARTESIAN_POINT('Ctrl Pts',(-0.112343157960958,-7.0789880113434,
-0.559500021225376));
#11608=CARTESIAN_POINT('Ctrl Pts',(0.205775730597156,-7.12921223581066,
-0.575200033960601));
#11609=CARTESIAN_POINT('Ctrl Pts',(0.339373595989117,-7.4222543897593,-0.590900046695826));
#11610=CARTESIAN_POINT('Ctrl Pts',(0.168651804056731,-7.69534093285333,
-0.606600059431053));
#11611=CARTESIAN_POINT('Ctrl Pts',(-0.15330148087219,-7.70359219825212,
-0.622300072166277));
#11612=CARTESIAN_POINT('Ctrl Pts',(-0.337788255924836,-7.43960989054611,
-0.638000084901503));
#11613=CARTESIAN_POINT('Ctrl Pts',(-0.219376257012592,-7.14010807885398,
-0.653700097636727));
#11614=CARTESIAN_POINT('Ctrl Pts',(0.0957509138319004,-7.07365573241465,
-0.669400110371954));
#11615=CARTESIAN_POINT('Ctrl Pts',(0.325020594078889,-7.29983561669969,
-0.685100123107178));
#11616=CARTESIAN_POINT('Ctrl Pts',(0.262834588646226,-7.6158415391922,-0.700800135842404));
#11617=CARTESIAN_POINT('Ctrl Pts',(-0.0350243992439388,-7.73828480188633,
-0.716500148577629));
#11618=CARTESIAN_POINT('Ctrl Pts',(-0.301503529702136,-7.55741606455238,
-0.732200161312854));
#11619=CARTESIAN_POINT('Ctrl Pts',(-0.297567376756904,-7.23532783720007,
-0.74790017404808));
#11620=CARTESIAN_POINT('Ctrl Pts',(-0.0269090023883596,-7.06102986635047,
-0.763600186783306));
#11621=CARTESIAN_POINT('Ctrl Pts',(0.268099680933479,-7.19043187069426,
-0.77930019951853));
#11622=CARTESIAN_POINT('Ctrl Pts',(0.32225063958776,-7.50828921687363,-0.795000212253757));
#11623=CARTESIAN_POINT('Ctrl Pts',(0.166339987378195,-7.65448997065358,
-0.805466887410573));
#11624=CARTESIAN_POINT('Ctrl Pts',(0.074593285434692,-7.67901775698422,
-0.810700224988981));
#11625=CARTESIAN_POINT('Ctrl Pts',(0.233606265769614,-7.20026984430693,
0.0321006749669432));
#11626=CARTESIAN_POINT('Ctrl Pts',(0.299281595044582,-7.27708432618563,
0.0268673373885347));
#11627=CARTESIAN_POINT('Ctrl Pts',(0.34788446529264,-7.49928149911123,0.0164006622317179));
#11628=CARTESIAN_POINT('Ctrl Pts',(0.108793687021496,-7.74539580169946,
0.000700649496492485));
#11629=CARTESIAN_POINT('Ctrl Pts',(-0.227926582539088,-7.68105106815663,
-0.0149993632387328));
#11630=CARTESIAN_POINT('Ctrl Pts',(-0.360224702622273,-7.36504429314182,
-0.0306993759739582));
#11631=CARTESIAN_POINT('Ctrl Pts',(-0.169525086729888,-7.08020524373302,
-0.0463993887091836));
#11632=CARTESIAN_POINT('Ctrl Pts',(0.1731988395346,-7.0822171223069,-0.0620994014444089));
#11633=CARTESIAN_POINT('Ctrl Pts',(0.360608974721706,-7.3691443808669,-0.0777994141796343));
#11634=CARTESIAN_POINT('Ctrl Pts',(0.224659927796838,-7.6837617716103,-0.0934994269148595));
#11635=CARTESIAN_POINT('Ctrl Pts',(-0.112744994253697,-7.74391654987674,
-0.109199439650085));
#11636=CARTESIAN_POINT('Ctrl Pts',(-0.349049821971846,-7.49568336784179,
-0.12489945238531));
#11637=CARTESIAN_POINT('Ctrl Pts',(-0.272358611429711,-7.16164735976291,
-0.140599465120536));
#11638=CARTESIAN_POINT('Ctrl Pts',(0.0485593205265976,-7.04134575574766,
-0.156299477855761));
#11639=CARTESIAN_POINT('Ctrl Pts',(0.32593357368315,-7.24265220640667,-0.171999490590986));
#11640=CARTESIAN_POINT('Ctrl Pts',(0.311040099268243,-7.58505425382268,
-0.187699503326212));
#11641=CARTESIAN_POINT('Ctrl Pts',(0.017233966595936,-7.7615162175086,-0.203399516061437));
#11642=CARTESIAN_POINT('Ctrl Pts',(-0.292026020701376,-7.61380319954907,
-0.219099528796662));
#11643=CARTESIAN_POINT('Ctrl Pts',(-0.339423477907051,-7.27437076234124,
-0.234799541531888));
#11644=CARTESIAN_POINT('Ctrl Pts',(-0.0824566440890477,-7.04759128714739,
-0.250499554267113));
#11645=CARTESIAN_POINT('Ctrl Pts',(0.248449852494269,-7.13682007602022,
-0.266199567002339));
#11646=CARTESIAN_POINT('Ctrl Pts',(0.356568983342811,-7.46204483232109,
-0.281899579737564));
#11647=CARTESIAN_POINT('Ctrl Pts',(0.144949285803845,-7.73163338988777,
-0.297599592472789));
#11648=CARTESIAN_POINT('Ctrl Pts',(-0.196647826769216,-7.70384310636604,
-0.313299605208015));
#11649=CARTESIAN_POINT('Ctrl Pts',(-0.361908946586785,-7.40359379384616,
-0.32899961794324));
#11650=CARTESIAN_POINT('Ctrl Pts',(-0.202642841972932,-7.10012189219636,
-0.344699630678465));
#11651=CARTESIAN_POINT('Ctrl Pts',(0.13833504309277,-7.06555356656853,-0.36039964341369));
#11652=CARTESIAN_POINT('Ctrl Pts',(0.355266567892898,-7.33088656640977,
-0.376099656148916));
#11653=CARTESIAN_POINT('Ctrl Pts',(0.253627152997932,-7.65819424514732,
-0.391799668884141));
#11654=CARTESIAN_POINT('Ctrl Pts',(-0.0754421632001089,-7.75397666730194,
-0.407499681619367));
#11655=CARTESIAN_POINT('Ctrl Pts',(-0.336861767851841,-7.53234481592602,
-0.423199694354592));
#11656=CARTESIAN_POINT('Ctrl Pts',(-0.29621419365842,-7.19203809856356,
-0.438899707089817));
#11657=CARTESIAN_POINT('Ctrl Pts',(0.010051489927223,-7.03821281309385,
-0.454599719825043));
#11658=CARTESIAN_POINT('Ctrl Pts',(0.307303905685085,-7.20880556939548,
-0.470299732560268));
#11659=CARTESIAN_POINT('Ctrl Pts',(0.328993961842462,-7.55084420496352,
-0.485999745295494));
#11660=CARTESIAN_POINT('Ctrl Pts',(0.0556719746423119,-7.75761939660742,
-0.501699758030718));
#11661=CARTESIAN_POINT('Ctrl Pts',(-0.267571603189326,-7.64371384083705,
-0.517399770765944));
#11662=CARTESIAN_POINT('Ctrl Pts',(-0.350881163774864,-7.31126775322783,
-0.533099783501169));
#11663=CARTESIAN_POINT('Ctrl Pts',(-0.119552205895206,-7.05838870778368,
-0.548799796236395));
#11664=CARTESIAN_POINT('Ctrl Pts',(0.21898033631151,-7.11183581514136,-0.56449980897162));
#11665=CARTESIAN_POINT('Ctrl Pts',(0.361151161846345,-7.42368245147158,
-0.580199821706845));
#11666=CARTESIAN_POINT('Ctrl Pts',(0.179474171539626,-7.71429292762124,
-0.595899834442071));
#11667=CARTESIAN_POINT('Ctrl Pts',(-0.16313881982596,-7.72307367580168,
-0.611599847177296));
#11668=CARTESIAN_POINT('Ctrl Pts',(-0.359464090686704,-7.44215165281094,
-0.627299859912522));
#11669=CARTESIAN_POINT('Ctrl Pts',(-0.23345360699228,-7.12343084321925,
-0.642999872647746));
#11670=CARTESIAN_POINT('Ctrl Pts',(0.101895239308332,-7.05271425710996,
-0.658699885382973));
#11671=CARTESIAN_POINT('Ctrl Pts',(0.345877129402089,-7.29340807937902,
-0.674399898118197));
#11672=CARTESIAN_POINT('Ctrl Pts',(0.279700654926715,-7.62969206672302,
-0.690099910853423));
#11673=CARTESIAN_POINT('Ctrl Pts',(-0.0372719110426151,-7.75999249994725,
-0.705799923588648));
#11674=CARTESIAN_POINT('Ctrl Pts',(-0.320850977623468,-7.56751743588265,
-0.721499936323874));
#11675=CARTESIAN_POINT('Ctrl Pts',(-0.316662242182126,-7.2247608428534,
-0.7371999490591));
#11676=CARTESIAN_POINT('Ctrl Pts',(-0.0286357500746574,-7.03927819062664,
-0.752899961794323));
#11677=CARTESIAN_POINT('Ctrl Pts',(0.285303607599647,-7.17698390717715,
-0.76859997452955));
#11678=CARTESIAN_POINT('Ctrl Pts',(0.342929427239765,-7.51523812385981,
-0.784299987264775));
#11679=CARTESIAN_POINT('Ctrl Pts',(0.177014005842305,-7.67082056372685,
-0.794766662421592));
#11680=CARTESIAN_POINT('Ctrl Pts',(0.0793799282532836,-7.69692229537457,
-0.8));
#11681=CARTESIAN_POINT('Ctrl Pts',(0.0793799282532837,-7.69692229537457,
-0.8));
#11682=CARTESIAN_POINT('Ctrl Pts',(0.0961911535774395,-7.69077267405574,
-0.8));
#11683=CARTESIAN_POINT('Ctrl Pts',(0.112330843922834,-7.68307124108963,
-0.800000000000001));
#11684=CARTESIAN_POINT('Ctrl Pts',(0.127669392025775,-7.67400023114597,
-0.800000000000001));
#11685=CARTESIAN_POINT('Ctrl Pts',(0.137645102295363,-7.66810073098187,
-0.8));
#11686=CARTESIAN_POINT('Ctrl Pts',(0.147281499905208,-7.66162083360303,
-0.8));
#11687=CARTESIAN_POINT('Ctrl Pts',(0.156535308745364,-7.65460204840892,
-0.8));
#11688=CARTESIAN_POINT('Ctrl Pts',(0.16394907438502,-7.6489788904852,-0.8));
#11689=CARTESIAN_POINT('Ctrl Pts',(0.171117175854576,-7.64300969246698,
-0.8));
#11690=CARTESIAN_POINT('Ctrl Pts',(0.178013695811224,-7.63671383667496,
-0.8));
#11691=CARTESIAN_POINT('Ctrl Pts',(0.181540623741549,-7.63349409254636,
-0.8));
#11692=CARTESIAN_POINT('Ctrl Pts',(0.18499019303302,-7.63019453557326,-0.8));
#11693=CARTESIAN_POINT('Ctrl Pts',(0.188356686614326,-7.62682145400554,
-0.8));
#11694=CARTESIAN_POINT('Ctrl Pts',(0.200715909300271,-7.61443804520746,
-0.8));
#11695=CARTESIAN_POINT('Ctrl Pts',(0.2119727366568,-7.60105296662967,-0.8));
#11696=CARTESIAN_POINT('Ctrl Pts',(0.221976954632972,-7.58681403533943,
-0.8));
#11697=CARTESIAN_POINT('Ctrl Pts',(0.228265905107983,-7.57786301748729,
-0.8));
#11698=CARTESIAN_POINT('Ctrl Pts',(0.234059046958926,-7.56857397550235,
-0.800000000000001));
#11699=CARTESIAN_POINT('Ctrl Pts',(0.239308880691954,-7.55898034246681,
-0.800000000000001));
#11700=CARTESIAN_POINT('Ctrl Pts',(0.241553642901407,-7.55487822685998,
-0.800000000000001));
#11701=CARTESIAN_POINT('Ctrl Pts',(0.243698962884783,-7.55072040648099,
-0.8));
#11702=CARTESIAN_POINT('Ctrl Pts',(0.245740613533059,-7.54650946019889,
-0.8));
#11703=CARTESIAN_POINT('Ctrl Pts',(0.247686929038575,-7.54249514460152,
-0.8));
#11704=CARTESIAN_POINT('Ctrl Pts',(0.249535114515858,-7.53844054532369,
-0.8));
#11705=CARTESIAN_POINT('Ctrl Pts',(0.251281773031569,-7.53435014256214,
-0.8));
#11706=CARTESIAN_POINT('Ctrl Pts',(0.25753761623788,-7.51969993011548,-0.8));
#11707=CARTESIAN_POINT('Ctrl Pts',(0.262498419038268,-7.50458280996037,
-0.800000000000001));
#11708=CARTESIAN_POINT('Ctrl Pts',(0.266024763128534,-7.48910875296159,
-0.800000000000001));
#11709=CARTESIAN_POINT('Ctrl Pts',(0.268541680001999,-7.47806419401775,
-0.8));
#11710=CARTESIAN_POINT('Ctrl Pts',(0.270326758003547,-7.46683739589159,
-0.8));
#11711=CARTESIAN_POINT('Ctrl Pts',(0.271391872668289,-7.45549714829965,
-0.800000000000001));
#11712=CARTESIAN_POINT('Ctrl Pts',(0.27180519341859,-7.45109653323119,-0.800000000000001));
#11713=CARTESIAN_POINT('Ctrl Pts',(0.272109991496476,-7.44667886409003,
-0.8));
#11714=CARTESIAN_POINT('Ctrl Pts',(0.272306569544964,-7.4422483195902,-0.8));
#11715=CARTESIAN_POINT('Ctrl Pts',(0.272509069569706,-7.43768430352772,
-0.8));
#11716=CARTESIAN_POINT('Ctrl Pts',(0.272596269292494,-7.43311641885229,
-0.8));
#11717=CARTESIAN_POINT('Ctrl Pts',(0.272569843180126,-7.42855121408732,
-0.8));
#11718=CARTESIAN_POINT('Ctrl Pts',(0.272471763334016,-7.41160757233752,
-0.8));
#11719=CARTESIAN_POINT('Ctrl Pts',(0.270813105492815,-7.3946899321374,-0.8));
#11720=CARTESIAN_POINT('Ctrl Pts',(0.267648469785739,-7.37802931988141,
-0.8));
#11721=CARTESIAN_POINT('Ctrl Pts',(0.265994340517827,-7.36932095376763,
-0.8));
#11722=CARTESIAN_POINT('Ctrl Pts',(0.263927860253695,-7.36068304066339,
-0.8));
#11723=CARTESIAN_POINT('Ctrl Pts',(0.261451436850857,-7.35215158032667,
-0.8));
#11724=CARTESIAN_POINT('Ctrl Pts',(0.26000111795531,-7.34715512531064,-0.8));
#11725=CARTESIAN_POINT('Ctrl Pts',(0.258409538895798,-7.34219357239197,
-0.8));
#11726=CARTESIAN_POINT('Ctrl Pts',(0.256678528275944,-7.33727990943004,
-0.8));
#11727=CARTESIAN_POINT('Ctrl Pts',(0.251357982528078,-7.32217695842633,
-0.8));
#11728=CARTESIAN_POINT('Ctrl Pts',(0.244748768101333,-7.30759386618852,
-0.8));
#11729=CARTESIAN_POINT('Ctrl Pts',(0.236874461322484,-7.2937452086627,-0.8));
#11730=CARTESIAN_POINT('Ctrl Pts',(0.232807858999536,-7.28659321618312,
-0.8));
#11731=CARTESIAN_POINT('Ctrl Pts',(0.228399170212801,-7.27963280000633,
-0.8));
#11732=CARTESIAN_POINT('Ctrl Pts',(0.223669087593591,-7.27292514292032,
-0.8));
#11733=CARTESIAN_POINT('Ctrl Pts',(0.21642296268428,-7.26264952513373,-0.8));
#11734=CARTESIAN_POINT('Ctrl Pts',(0.208418195009514,-7.25295420792725,
-0.8));
#11735=CARTESIAN_POINT('Ctrl Pts',(0.199658648264246,-7.24395737393901,
-0.8));
#11736=CARTESIAN_POINT('Ctrl Pts',(0.197072110678764,-7.24130076967196,
-0.8));
#11737=CARTESIAN_POINT('Ctrl Pts',(0.194419670008508,-7.23870520686924,
-0.8));
#11738=CARTESIAN_POINT('Ctrl Pts',(0.191704041017359,-7.23617187252307,
-0.8));
#11739=CARTESIAN_POINT('Ctrl Pts',(0.191346599666505,-7.2364012796625,0.));
#11740=CARTESIAN_POINT('Ctrl Pts',(0.202509817473759,-7.24689196324677,
-4.25187765113737E-19));
#11741=CARTESIAN_POINT('Ctrl Pts',(0.212570029866005,-7.25841325449013,
1.70283439359328E-17));
#11742=CARTESIAN_POINT('Ctrl Pts',(0.221522302700304,-7.27074765126196,
1.73472347597681E-17));
#11743=CARTESIAN_POINT('Ctrl Pts',(0.229528851253605,-7.28177903384573,
1.76324377368777E-17));
#11744=CARTESIAN_POINT('Ctrl Pts',(0.236649204955062,-7.29346212976217,
-1.68985376951836E-17));
#11745=CARTESIAN_POINT('Ctrl Pts',(0.242860412371513,-7.30566884695974,
1.73472347597681E-18));
#11746=CARTESIAN_POINT('Ctrl Pts',(0.244940798159157,-7.30975737263099,
7.97575989914875E-18));
#11747=CARTESIAN_POINT('Ctrl Pts',(0.246919671013813,-7.31390628918125,
1.8683266199719E-17));
#11748=CARTESIAN_POINT('Ctrl Pts',(0.248793544918815,-7.31810659182485,
2.08166817117217E-17));
#11749=CARTESIAN_POINT('Ctrl Pts',(0.255493762728008,-7.33312518112348,
2.84449156978875E-17));
#11750=CARTESIAN_POINT('Ctrl Pts',(0.260811093553058,-7.34869786677283,
7.65141509275329E-17));
#11751=CARTESIAN_POINT('Ctrl Pts',(0.264722827386125,-7.36459856759787,
5.89805981832114E-17));
#11752=CARTESIAN_POINT('Ctrl Pts',(0.267427565046703,-7.37559298239867,
4.68571607370262E-17));
#11753=CARTESIAN_POINT('Ctrl Pts',(0.269459624700383,-7.38674528662227,
4.0452509126737E-17));
#11754=CARTESIAN_POINT('Ctrl Pts',(0.270799674072059,-7.39798906439888,
4.16333634234434E-17));
#11755=CARTESIAN_POINT('Ctrl Pts',(0.271554626847406,-7.40432354834945,
4.22986293811185E-17));
#11756=CARTESIAN_POINT('Ctrl Pts',(0.27208975223859,-7.41068715911504,6.88910133647342E-17));
#11757=CARTESIAN_POINT('Ctrl Pts',(0.272399999297887,-7.41706844790294,
6.59194920871187E-17));
#11758=CARTESIAN_POINT('Ctrl Pts',(0.272610263460686,-7.4213932474598,6.39055989172972E-17));
#11759=CARTESIAN_POINT('Ctrl Pts',(0.272716738029981,-7.42571709930175,
-1.06875105497055E-17));
#11760=CARTESIAN_POINT('Ctrl Pts',(0.272718929390231,-7.43003454190223,
-8.67361737988404E-18));
#11761=CARTESIAN_POINT('Ctrl Pts',(0.272726931468211,-7.44580032589523,
-1.31958684872211E-18));
#11762=CARTESIAN_POINT('Ctrl Pts',(0.27134758489836,-7.46148679133341,5.78590717144025E-17));
#11763=CARTESIAN_POINT('Ctrl Pts',(0.268538129113132,-7.47691813343808,
5.20417042793042E-17));
#11764=CARTESIAN_POINT('Ctrl Pts',(0.266219645760504,-7.4896527384696,4.04832294204731E-17));
#11765=CARTESIAN_POINT('Ctrl Pts',(0.262926744086474,-7.50221429697178,
3.27839278289332E-17));
#11766=CARTESIAN_POINT('Ctrl Pts',(0.258732626744963,-7.51453551399731,
4.5102810375397E-17));
#11767=CARTESIAN_POINT('Ctrl Pts',(0.256787792726102,-7.52024892639706,
5.08151402650737E-17));
#11768=CARTESIAN_POINT('Ctrl Pts',(0.254646875440068,-7.52591460238169,
4.71189268070476E-17));
#11769=CARTESIAN_POINT('Ctrl Pts',(0.252327893343031,-7.5314990454491,4.5102810375397E-17));
#11770=CARTESIAN_POINT('Ctrl Pts',(0.245813460854531,-7.54718673764602,
3.94391813203355E-17));
#11771=CARTESIAN_POINT('Ctrl Pts',(0.237886907768047,-7.56227236975653,
3.73105788674031E-17));
#11772=CARTESIAN_POINT('Ctrl Pts',(0.228725878996942,-7.5766134557043,1.04083408558608E-17));
#11773=CARTESIAN_POINT('Ctrl Pts',(0.223374521430301,-7.58499071121981,
-5.30643294735275E-18));
#11774=CARTESIAN_POINT('Ctrl Pts',(0.217600893833204,-7.59311391451407,
3.69689762542118E-17));
#11775=CARTESIAN_POINT('Ctrl Pts',(0.211432791129273,-7.60095290540197,
3.46944695195361E-17));
#11776=CARTESIAN_POINT('Ctrl Pts',(0.207420148579369,-7.60605253974577,
3.32147953082452E-17));
#11777=CARTESIAN_POINT('Ctrl Pts',(0.20324045059128,-7.61103185738154,2.54856801722722E-17));
#11778=CARTESIAN_POINT('Ctrl Pts',(0.198900278349408,-7.61588193104767,
3.12250225675825E-17));
#11779=CARTESIAN_POINT('Ctrl Pts',(0.195670728628085,-7.61949090165619,
3.54957036835372E-17));
#11780=CARTESIAN_POINT('Ctrl Pts',(0.19235503384787,-7.62302506290143,1.08425633614596E-17));
#11781=CARTESIAN_POINT('Ctrl Pts',(0.188962047141393,-7.62647538090844,
6.93889390390723E-18));
#11782=CARTESIAN_POINT('Ctrl Pts',(0.179751979430083,-7.63584107114516,
-3.65739283013793E-18));
#11783=CARTESIAN_POINT('Ctrl Pts',(0.169961756459919,-7.64460258732274,
1.58981699072491E-17));
#11784=CARTESIAN_POINT('Ctrl Pts',(0.15965473466309,-7.65269275268246,1.73472347597681E-17));
#11785=CARTESIAN_POINT('Ctrl Pts',(0.154922700033441,-7.6564070111168,1.80125118104906E-17));
#11786=CARTESIAN_POINT('Ctrl Pts',(0.150081554712747,-7.65997966275367,
2.66878873465253E-17));
#11787=CARTESIAN_POINT('Ctrl Pts',(0.145136600582228,-7.66340356863892,
3.81639164714898E-17));
#11788=CARTESIAN_POINT('Ctrl Pts',(0.139976052344163,-7.66697675274073,
5.01402867911481E-17));
#11789=CARTESIAN_POINT('Ctrl Pts',(0.134708897983985,-7.67038332088609,
-3.16234153219695E-17));
#11790=CARTESIAN_POINT('Ctrl Pts',(0.129346789376753,-7.67361307290272,
-1.73472347597681E-17));
#11791=CARTESIAN_POINT('Ctrl Pts',(0.117404965946791,-7.68080597612983,
1.44469044522131E-17));
#11792=CARTESIAN_POINT('Ctrl Pts',(0.10498570886698,-7.68712791357992,2.06413296011656E-17));
#11793=CARTESIAN_POINT('Ctrl Pts',(0.0921567849037076,-7.69249315206613,
-2.08166817117217E-17));
#11794=CARTESIAN_POINT('Ctrl Pts',(0.0880066762640415,-7.69422878653238,
-3.42281924062706E-17));
#11795=CARTESIAN_POINT('Ctrl Pts',(0.0838136017590666,-7.69586419192416,
-4.59422420206302E-18));
#11796=CARTESIAN_POINT('Ctrl Pts',(0.0795809081573363,-7.69740028961993,
-6.93889390390723E-18));
#11797=CARTESIAN_POINT('Ctrl Pts',(-0.2516645197469,-7.40021351101923,-0.161258330249198));
#11798=CARTESIAN_POINT('Ctrl Pts',(-0.251853760397228,-7.42268031128274,
-0.15983892928355));
#11799=CARTESIAN_POINT('Ctrl Pts',(-0.249087077319634,-7.445101303405,-0.158419528317902));
#11800=CARTESIAN_POINT('Ctrl Pts',(-0.243177161464371,-7.46666062885335,
-0.157000127352254));
#11801=CARTESIAN_POINT('Ctrl Pts',(-0.221387275816053,-7.54614995622776,
-0.151766789773845));
#11802=CARTESIAN_POINT('Ctrl Pts',(-0.156868279689982,-7.61392578571347,
-0.146533452195437));
#11803=CARTESIAN_POINT('Ctrl Pts',(-0.0785474567930319,-7.63960158320207,
-0.141300114617028));
#11804=CARTESIAN_POINT('Ctrl Pts',(-0.000226633896081616,-7.66527738069067,
-0.13606677703862));
#11805=CARTESIAN_POINT('Ctrl Pts',(0.0918960157717476,-7.64885314618216,
-0.130833439460211));
#11806=CARTESIAN_POINT('Ctrl Pts',(0.156516622945739,-7.59769057715216,
-0.125600101881803));
#11807=CARTESIAN_POINT('Ctrl Pts',(0.22113723011973,-7.54652800812215,-0.120366764303394));
#11808=CARTESIAN_POINT('Ctrl Pts',(0.258255794799884,-7.46062710457066,
-0.115133426724986));
#11809=CARTESIAN_POINT('Ctrl Pts',(0.251230509311017,-7.37850635978343,
-0.109900089146578));
#11810=CARTESIAN_POINT('Ctrl Pts',(0.244205223822151,-7.2963856149962,-0.104666751568169));
#11811=CARTESIAN_POINT('Ctrl Pts',(0.193036088164265,-7.21804502897323,
-0.0994334139897607));
#11812=CARTESIAN_POINT('Ctrl Pts',(0.120664063886602,-7.17860008142513,
-0.0942000764113522));
#11813=CARTESIAN_POINT('Ctrl Pts',(0.048292039608938,-7.13915513387703,
-0.0889667388329437));
#11814=CARTESIAN_POINT('Ctrl Pts',(-0.0452828732885026,-7.13860582480379,
-0.0837334012545353));
#11815=CARTESIAN_POINT('Ctrl Pts',(-0.118103965820357,-7.177216388362,-0.0785000636761268));
#11816=CARTESIAN_POINT('Ctrl Pts',(-0.190925058352211,-7.21582695192021,
-0.0732667260977184));
#11817=CARTESIAN_POINT('Ctrl Pts',(-0.242992330518479,-7.29359738810986,
-0.06803338851931));
#11818=CARTESIAN_POINT('Ctrl Pts',(-0.250965095861989,-7.37562273179982,
-0.0628000509409015));
#11819=CARTESIAN_POINT('Ctrl Pts',(-0.251748010978523,-7.3836775131394,
-0.062286144043667));
#11820=CARTESIAN_POINT('Ctrl Pts',(-0.252105723523339,-7.3917733244789,
-0.0617722371464325));
#11821=CARTESIAN_POINT('Ctrl Pts',(-0.25205356191611,-7.39987360404796,
-0.0612583302491979));
#11822=CARTESIAN_POINT('Ctrl Pts',(-0.0793799282532839,-7.69692229537457,
2.77555756156289E-17));
#11823=CARTESIAN_POINT('Ctrl Pts',(-0.177014005842305,-7.67082056372685,
-0.00523333757840842));
#11824=CARTESIAN_POINT('Ctrl Pts',(-0.342929400138797,-7.51523794788106,
-0.0157000127352253));
#11825=CARTESIAN_POINT('Ctrl Pts',(-0.285303631037492,-7.17698397189122,
-0.0314000254704507));
#11826=CARTESIAN_POINT('Ctrl Pts',(0.0286357521188298,-7.03927813304723,
-0.047100038205676));
#11827=CARTESIAN_POINT('Ctrl Pts',(0.31666225793602,-7.22476085896309,-0.0628000509409014));
#11828=CARTESIAN_POINT('Ctrl Pts',(0.320850989126134,-7.56751742991046,
-0.0785000636761266));
#11829=CARTESIAN_POINT('Ctrl Pts',(0.0372719144191142,-7.75999252270946,
-0.0942000764113521));
#11830=CARTESIAN_POINT('Ctrl Pts',(-0.27970066815779,-7.62969207265103,
-0.109900089146577));
#11831=CARTESIAN_POINT('Ctrl Pts',(-0.345877143550449,-7.29340807693237,
-0.125600101881803));
#11832=CARTESIAN_POINT('Ctrl Pts',(-0.101895244140074,-7.05271424100694,
-0.141300114617028));
#11833=CARTESIAN_POINT('Ctrl Pts',(0.233453617301762,-7.1234308319262,-0.157000127352253));
#11834=CARTESIAN_POINT('Ctrl Pts',(0.359464106016436,-7.44215165429935,
-0.172700140087479));
#11835=CARTESIAN_POINT('Ctrl Pts',(0.163138826931865,-7.72307368988404,
-0.188400152822704));
#11836=CARTESIAN_POINT('Ctrl Pts',(-0.179474179312067,-7.714292941062,-0.204100165557929));
#11837=CARTESIAN_POINT('Ctrl Pts',(-0.36115117737076,-7.42368245253896,
-0.219800178293155));
#11838=CARTESIAN_POINT('Ctrl Pts',(-0.218980345752975,-7.11183580270963,
-0.23550019102838));
#11839=CARTESIAN_POINT('Ctrl Pts',(0.119552211049655,-7.05838869308885,
-0.251200203763606));
#11840=CARTESIAN_POINT('Ctrl Pts',(0.350881178877997,-7.31126774940073,
-0.266900216498831));
#11841=CARTESIAN_POINT('Ctrl Pts',(0.267571614711511,-7.64371385133353,
-0.282600229234056));
#11842=CARTESIAN_POINT('Ctrl Pts',(-0.0556719770403169,-7.75761941200269,
-0.298300241969282));
#11843=CARTESIAN_POINT('Ctrl Pts',(-0.328993976006532,-7.55084421145899,
-0.314000254704507));
#11844=CARTESIAN_POINT('Ctrl Pts',(-0.307303918916174,-7.20880556116322,
-0.329700267439732));
#11845=CARTESIAN_POINT('Ctrl Pts',(-0.0100514903598289,-7.03821279751757,
-0.345400280174958));
#11846=CARTESIAN_POINT('Ctrl Pts',(0.296214206411665,-7.19203808960976,
-0.361100292910183));
#11847=CARTESIAN_POINT('Ctrl Pts',(0.336861782355269,-7.53234482162411,
-0.376800305645408));
#11848=CARTESIAN_POINT('Ctrl Pts',(0.0754421664482044,-7.75397668254217,
-0.392500318380634));
#11849=CARTESIAN_POINT('Ctrl Pts',(-0.253627163917688,-7.65819425626374,
-0.408200331115859));
#11850=CARTESIAN_POINT('Ctrl Pts',(-0.355266583188697,-7.3308865634341,
-0.423900343851084));
#11851=CARTESIAN_POINT('Ctrl Pts',(-0.138335049048699,-7.06555355216919,
-0.43960035658631));
#11852=CARTESIAN_POINT('Ctrl Pts',(0.202642850697595,-7.1001218792852,-0.455300369321535));
#11853=CARTESIAN_POINT('Ctrl Pts',(0.361908962168568,-7.40359379400104,
-0.47100038205676));
#11854=CARTESIAN_POINT('Ctrl Pts',(0.196647835235759,-7.70384311944753,
-0.486700394791986));
#11855=CARTESIAN_POINT('Ctrl Pts',(-0.144949292044521,-7.73163340416662,
-0.502400407527211));
#11856=CARTESIAN_POINT('Ctrl Pts',(-0.356568998694743,-7.46204483499129,
-0.518100420262437));
#11857=CARTESIAN_POINT('Ctrl Pts',(-0.24844986319099,-7.13682006469127,
-0.533800432997662));
#11858=CARTESIAN_POINT('Ctrl Pts',(0.0824566476388583,-7.04759127197059,
-0.549500445732887));
#11859=CARTESIAN_POINT('Ctrl Pts',(0.3394234925214,-7.27437075694011,-0.565200458468112));
#11860=CARTESIAN_POINT('Ctrl Pts',(0.292026033272937,-7.61380320873943,
-0.580900471203338));
#11861=CARTESIAN_POINT('Ctrl Pts',(-0.0172339673348224,-7.76151623310164,
-0.596600483938563));
#11862=CARTESIAN_POINT('Ctrl Pts',(-0.311040112666544,-7.58505426173674,
-0.612300496673788));
#11863=CARTESIAN_POINT('Ctrl Pts',(-0.325933587701845,-7.24265219973275,
-0.628000509409014));
#11864=CARTESIAN_POINT('Ctrl Pts',(-0.0485593226474429,-7.04134574011728,
-0.643700522144239));
#11865=CARTESIAN_POINT('Ctrl Pts',(0.272358623219876,-7.16164734985291,
-0.659400534879465));
#11866=CARTESIAN_POINT('Ctrl Pts',(0.349049836864763,-7.49568337130869,
-0.675100547614689));
#11867=CARTESIAN_POINT('Ctrl Pts',(0.11274499939327,-7.74391656588417,-0.690800560349915));
#11868=CARTESIAN_POINT('Ctrl Pts',(-0.224659938070643,-7.68376178164081,
-0.706500573085141));
#11869=CARTESIAN_POINT('Ctrl Pts',(-0.360608988983327,-7.36914438347625,
-0.722200585820365));
#11870=CARTESIAN_POINT('Ctrl Pts',(-0.173198849645488,-7.08221710163593,
-0.737900598555592));
#11871=CARTESIAN_POINT('Ctrl Pts',(0.169525099592154,-7.08020524213913,
-0.753600611290816));
#11872=CARTESIAN_POINT('Ctrl Pts',(0.360224706479889,-7.36504427094214,
-0.769300624026043));
#11873=CARTESIAN_POINT('Ctrl Pts',(0.227926616839064,-7.68105111445003,
-0.785000636761266));
#11874=CARTESIAN_POINT('Ctrl Pts',(-0.108793742993405,-7.74539576164464,
-0.800700649496493));
#11875=CARTESIAN_POINT('Ctrl Pts',(-0.347884343277012,-7.49928162878455,
-0.816400662231718));
#11876=CARTESIAN_POINT('Ctrl Pts',(-0.299281595044583,-7.27708432618564,
-0.826867337388535));
#11877=CARTESIAN_POINT('Ctrl Pts',(-0.233606265769615,-7.20026984430694,
-0.832100674966943));
#11878=CARTESIAN_POINT('Ctrl Pts',(-0.074593285434692,-7.67901775698422,
0.0107002249889811));
#11879=CARTESIAN_POINT('Ctrl Pts',(-0.166339987378195,-7.65448997065358,
0.00546688741057264));
#11880=CARTESIAN_POINT('Ctrl Pts',(-0.322250614120992,-7.50828905150648,
-0.00499978774624427));
#11881=CARTESIAN_POINT('Ctrl Pts',(-0.268099702958013,-7.19043193150604,
-0.0206998004814696));
#11882=CARTESIAN_POINT('Ctrl Pts',(0.0269090043092675,-7.06102981224313,
-0.036399813216695));
#11883=CARTESIAN_POINT('Ctrl Pts',(0.297567391560831,-7.23532785233835,
-0.0520998259519202));
#11884=CARTESIAN_POINT('Ctrl Pts',(0.301503540511186,-7.55741605894031,
-0.0677998386871457));
#11885=CARTESIAN_POINT('Ctrl Pts',(0.0350244024168338,-7.73828482327598,
-0.0834998514223709));
#11886=CARTESIAN_POINT('Ctrl Pts',(-0.262834601079461,-7.61584154476274,
-0.0991998641575964));
#11887=CARTESIAN_POINT('Ctrl Pts',(-0.325020607374097,-7.29983561440058,
-0.114899876892822));
#11888=CARTESIAN_POINT('Ctrl Pts',(-0.0957509183722879,-7.07365571728264,
-0.130599889628047));
#11889=CARTESIAN_POINT('Ctrl Pts',(0.219376266700408,-7.14010806824191,
-0.146299902363272));
#11890=CARTESIAN_POINT('Ctrl Pts',(0.337788270330178,-7.43960989194476,
-0.161999915098498));
#11891=CARTESIAN_POINT('Ctrl Pts',(0.153301487549606,-7.70359221148531,
-0.177699927833723));
#11892=CARTESIAN_POINT('Ctrl Pts',(-0.168651811360491,-7.69534094548361,
-0.193399940568948));
#11893=CARTESIAN_POINT('Ctrl Pts',(-0.339373610577404,-7.42225439076231,
-0.209099953304174));
#11894=CARTESIAN_POINT('Ctrl Pts',(-0.205775739469297,-7.12921222412858,
-0.224799966039399));
#11895=CARTESIAN_POINT('Ctrl Pts',(0.112343162804592,-7.07898799753467,
-0.240499978774624));
#11896=CARTESIAN_POINT('Ctrl Pts',(0.329722897281971,-7.31661834116182,
-0.25619999150985));
#11897=CARTESIAN_POINT('Ctrl Pts',(0.251436934620453,-7.62901780433593,
-0.271900004245075));
#11898=CARTESIAN_POINT('Ctrl Pts',(-0.0523149335790711,-7.73605481213571,
-0.287600016980301));
#11899=CARTESIAN_POINT('Ctrl Pts',(-0.309155501882608,-7.54174824252333,
-0.303300029715526));
#11900=CARTESIAN_POINT('Ctrl Pts',(-0.288773364291437,-7.22033466565791,
-0.319000042450751));
#11901=CARTESIAN_POINT('Ctrl Pts',(-0.00944538129415302,-7.06002871689073,
-0.334700055185977));
#11902=CARTESIAN_POINT('Ctrl Pts',(0.278352366081435,-7.20457827964033,
-0.350400067921202));
#11903=CARTESIAN_POINT('Ctrl Pts',(0.316548876223331,-7.52436437361988,
-0.366100080656427));
#11904=CARTESIAN_POINT('Ctrl Pts',(0.0708929723106632,-7.73263174078266,
-0.381800093391653));
#11905=CARTESIAN_POINT('Ctrl Pts',(-0.238333340031973,-7.64262503480259,
-0.397500106126878));
#11906=CARTESIAN_POINT('Ctrl Pts',(-0.333843859881619,-7.33505413251718,
-0.413200118862103));
#11907=CARTESIAN_POINT('Ctrl Pts',(-0.12999338782956,-7.08572081262079,
-0.428900131597328));
#11908=CARTESIAN_POINT('Ctrl Pts',(0.190423402187442,-7.11820465517776,
-0.444600144332554));
#11909=CARTESIAN_POINT('Ctrl Pts',(0.340085700635493,-7.4033770867222,-0.460300157067779));
#11910=CARTESIAN_POINT('Ctrl Pts',(0.184789888661161,-7.6855212524758,-0.476000169803005));
#11911=CARTESIAN_POINT('Ctrl Pts',(-0.13620878921097,-7.71163577142256,
-0.491700182538229));
#11912=CARTESIAN_POINT('Ctrl Pts',(-0.33506773918883,-7.45830350553463,
-0.507400195273456));
#11913=CARTESIAN_POINT('Ctrl Pts',(-0.233468232700866,-7.15268992468061,
-0.52310020800868));
#11914=CARTESIAN_POINT('Ctrl Pts',(0.0774844773566386,-7.06884166541827,
-0.538800220743906));
#11915=CARTESIAN_POINT('Ctrl Pts',(0.318956114196808,-7.28194625275284,
-0.554500233479131));
#11916=CARTESIAN_POINT('Ctrl Pts',(0.274416741531735,-7.60091078597937,
-0.570200246214357));
#11917=CARTESIAN_POINT('Ctrl Pts',(-0.0161947519085262,-7.73971665329528,
-0.585900258949582));
#11918=CARTESIAN_POINT('Ctrl Pts',(-0.292284263998619,-7.57389541248501,
-0.601600271684807));
#11919=CARTESIAN_POINT('Ctrl Pts',(-0.306279656270553,-7.2521403377891,
-0.617300284420032));
#11920=CARTESIAN_POINT('Ctrl Pts',(-0.0456311752159611,-7.06297274174353,
-0.633000297155258));
#11921=CARTESIAN_POINT('Ctrl Pts',(0.255935284516958,-7.17602011418042,
-0.648700309890483));
#11922=CARTESIAN_POINT('Ctrl Pts',(0.328001985956807,-7.48991362406639,
-0.664400322625709));
#11923=CARTESIAN_POINT('Ctrl Pts',(0.105946428853423,-7.72317825335973,
-0.680100335360934));
#11924=CARTESIAN_POINT('Ctrl Pts',(-0.211112849998708,-7.66665082772375,
-0.695800348096159));
#11925=CARTESIAN_POINT('Ctrl Pts',(-0.338864116376122,-7.37100499003633,
-0.711500360831385));
#11926=CARTESIAN_POINT('Ctrl Pts',(-0.162754886693057,-7.10137954309684,
-0.72720037356661));
#11927=CARTESIAN_POINT('Ctrl Pts',(0.159302665301906,-7.09948899956776,
-0.742900386301835));
#11928=CARTESIAN_POINT('Ctrl Pts',(0.338503006268098,-7.36715211600001,
-0.758600399037061));
#11929=CARTESIAN_POINT('Ctrl Pts',(0.214182546673399,-7.66410361489641,
-0.774300411772286));
#11930=CARTESIAN_POINT('Ctrl Pts',(-0.102233434864309,-7.7245682529982,
-0.790000424507512));
#11931=CARTESIAN_POINT('Ctrl Pts',(-0.326906772119047,-7.49329490511401,
-0.805700437242737));
#11932=CARTESIAN_POINT('Ctrl Pts',(-0.281234789899006,-7.28449619263982,
-0.816167112399554));
#11933=CARTESIAN_POINT('Ctrl Pts',(-0.219519710401912,-7.21231365609213,
-0.821400449977962));
#11934=CARTESIAN_POINT('Ctrl Pts',(-0.0698066426161,-7.66111321859386,0.0214004499779622));
#11935=CARTESIAN_POINT('Ctrl Pts',(-0.155665968914086,-7.6381593775803,
0.0161671123995537));
#11936=CARTESIAN_POINT('Ctrl Pts',(-0.301571828103187,-7.50134015513189,
0.00570043724273681));
#11937=CARTESIAN_POINT('Ctrl Pts',(-0.250895774878533,-7.20387989112088,
-0.00999957549248853));
#11938=CARTESIAN_POINT('Ctrl Pts',(0.0251822564997051,-7.08278149143901,
-0.0256995882277139));
#11939=CARTESIAN_POINT('Ctrl Pts',(0.278472525185642,-7.2458948457136,-0.0413996009629392));
#11940=CARTESIAN_POINT('Ctrl Pts',(0.282156091896237,-7.54731468797016,
-0.0570996136981646));
#11941=CARTESIAN_POINT('Ctrl Pts',(0.0327768904145534,-7.7165771238425,
-0.0727996264333898));
#11942=CARTESIAN_POINT('Ctrl Pts',(-0.245968534001132,-7.60199101687444,
-0.0884996391686154));
#11943=CARTESIAN_POINT('Ctrl Pts',(-0.304164071197746,-7.30626315186879,
-0.10419965190384));
#11944=CARTESIAN_POINT('Ctrl Pts',(-0.0896065926045006,-7.09459719355835,
-0.119899664639066));
#11945=CARTESIAN_POINT('Ctrl Pts',(0.205298916099055,-7.15678530455762,
-0.135599677374291));
#11946=CARTESIAN_POINT('Ctrl Pts',(0.316112434643921,-7.43706812959018,
-0.151299690109517));
#11947=CARTESIAN_POINT('Ctrl Pts',(0.143464148167348,-7.68411073308658,
-0.166999702844742));
#11948=CARTESIAN_POINT('Ctrl Pts',(-0.157829443408914,-7.67638894990523,
-0.182699715579967));
#11949=CARTESIAN_POINT('Ctrl Pts',(-0.317596043784047,-7.42082632898565,
-0.198399728315193));
#11950=CARTESIAN_POINT('Ctrl Pts',(-0.192571133185619,-7.14658864554754,
-0.214099741050418));
#11951=CARTESIAN_POINT('Ctrl Pts',(0.105134114559528,-7.09958730198047,
-0.229799753785643));
#11952=CARTESIAN_POINT('Ctrl Pts',(0.308564615685943,-7.32196893292292,
-0.245499766520869));
#11953=CARTESIAN_POINT('Ctrl Pts',(0.235302254529395,-7.61432175733832,
-0.261199779256094));
#11954=CARTESIAN_POINT('Ctrl Pts',(-0.0489578901178251,-7.71449021226873,
-0.276899791991319));
#11955=CARTESIAN_POINT('Ctrl Pts',(-0.289317027758686,-7.53265227358768,
-0.292599804726545));
#11956=CARTESIAN_POINT('Ctrl Pts',(-0.270242809666699,-7.2318637701526,
-0.30829981746177));
#11957=CARTESIAN_POINT('Ctrl Pts',(-0.00883927222847752,-7.08184463626389,
-0.323999830196995));
#11958=CARTESIAN_POINT('Ctrl Pts',(0.260490525751205,-7.21711846967092,
-0.339699842932221));
#11959=CARTESIAN_POINT('Ctrl Pts',(0.296235970091394,-7.51638392561565,
-0.355399855667446));
#11960=CARTESIAN_POINT('Ctrl Pts',(0.0663437781731218,-7.71128679902317,
-0.371099868402672));
#11961=CARTESIAN_POINT('Ctrl Pts',(-0.223039516146258,-7.62705581334143,
-0.386799881137897));
#11962=CARTESIAN_POINT('Ctrl Pts',(-0.312421136574541,-7.33922170160028,
-0.402499893873123));
#11963=CARTESIAN_POINT('Ctrl Pts',(-0.12165172661042,-7.10588807307238,
-0.418199906608347));
#11964=CARTESIAN_POINT('Ctrl Pts',(0.17820395367729,-7.13628743107034,-0.433899919343573));
#11965=CARTESIAN_POINT('Ctrl Pts',(0.318262439102417,-7.40316037944335,
-0.449599932078798));
#11966=CARTESIAN_POINT('Ctrl Pts',(0.172931942086563,-7.66719938550407,
-0.465299944814024));
#11967=CARTESIAN_POINT('Ctrl Pts',(-0.127468286377419,-7.69163813867849,
-0.480999957549249));
#11968=CARTESIAN_POINT('Ctrl Pts',(-0.313566479682916,-7.45456217607797,
-0.496699970284474));
#11969=CARTESIAN_POINT('Ctrl Pts',(-0.218486602210741,-7.16855978466994,
-0.512399983019699));
#11970=CARTESIAN_POINT('Ctrl Pts',(0.0725123070744189,-7.09009205886595,
-0.528099995754925));
#11971=CARTESIAN_POINT('Ctrl Pts',(0.298488735872217,-7.28952174856557,
-0.54380000849015));
#11972=CARTESIAN_POINT('Ctrl Pts',(0.256807449790533,-7.58801836321932,
-0.559500021225376));
#11973=CARTESIAN_POINT('Ctrl Pts',(-0.0151555364822303,-7.71791707348892,
-0.5752000339606));
#11974=CARTESIAN_POINT('Ctrl Pts',(-0.273528415330694,-7.56273656323327,
-0.590900046695827));
#11975=CARTESIAN_POINT('Ctrl Pts',(-0.286625724839261,-7.26162847584545,
-0.606600059431051));
#11976=CARTESIAN_POINT('Ctrl Pts',(-0.0427030277844796,-7.08459974336978,
-0.622300072166277));
#11977=CARTESIAN_POINT('Ctrl Pts',(0.239511945814041,-7.19039287850791,
-0.638000084901502));
#11978=CARTESIAN_POINT('Ctrl Pts',(0.306954135048851,-7.4841438768241,-0.653700097636728));
#11979=CARTESIAN_POINT('Ctrl Pts',(0.0991478583135767,-7.70243994083529,
-0.669400110371953));
#11980=CARTESIAN_POINT('Ctrl Pts',(-0.197565761926773,-7.64953987380668,
-0.685100123107178));
#11981=CARTESIAN_POINT('Ctrl Pts',(-0.317119243768918,-7.37286559659641,
-0.700800135842404));
#11982=CARTESIAN_POINT('Ctrl Pts',(-0.152310923740626,-7.12054198455776,
-0.716500148577628));
#11983=CARTESIAN_POINT('Ctrl Pts',(0.149080231011657,-7.11877275699639,
-0.732200161312855));
#11984=CARTESIAN_POINT('Ctrl Pts',(0.316781306056307,-7.36925996105789,
-0.747900174048079));
#11985=CARTESIAN_POINT('Ctrl Pts',(0.200438476507733,-7.64715611534278,
-0.763600186783305));
#11986=CARTESIAN_POINT('Ctrl Pts',(-0.0956731267352124,-7.70374074435177,
-0.779300199518531));
#11987=CARTESIAN_POINT('Ctrl Pts',(-0.305929200961081,-7.48730818144347,
-0.795000212253756));
#11988=CARTESIAN_POINT('Ctrl Pts',(-0.26318798475343,-7.291908059094,-0.805466887410573));
#11989=CARTESIAN_POINT('Ctrl Pts',(-0.205433155034209,-7.22435746787732,
-0.810700224988981));
#11990=CARTESIAN_POINT('Ctrl Pts',(-0.0650199997975081,-7.64320868020351,
0.0321006749669432));
#11991=CARTESIAN_POINT('Ctrl Pts',(-0.144991950449976,-7.62182878450703,
0.0268673373885348));
#11992=CARTESIAN_POINT('Ctrl Pts',(-0.280893042085382,-7.4943912587573,
0.0164006622317179));
#11993=CARTESIAN_POINT('Ctrl Pts',(-0.233691846799053,-7.2173278507357,
0.000700649496492526));
#11994=CARTESIAN_POINT('Ctrl Pts',(0.0234555086901425,-7.10453317063491,
-0.0149993632387329));
#11995=CARTESIAN_POINT('Ctrl Pts',(0.259377658810454,-7.25646183908885,
-0.0306993759739581));
#11996=CARTESIAN_POINT('Ctrl Pts',(0.262808643281289,-7.53721331700002,
-0.0463993887091836));
#11997=CARTESIAN_POINT('Ctrl Pts',(0.030529378412273,-7.694869424409,-0.0620994014444088));
#11998=CARTESIAN_POINT('Ctrl Pts',(-0.229102466922803,-7.58814048898617,
-0.0777994141796343));
#11999=CARTESIAN_POINT('Ctrl Pts',(-0.283307535021394,-7.31269068933698,
-0.0934994269148594));
#12000=CARTESIAN_POINT('Ctrl Pts',(-0.0834622668367136,-7.11553866983406,
-0.109199439650085));
#12001=CARTESIAN_POINT('Ctrl Pts',(0.191221565497701,-7.17346254087333,
-0.12489945238531));
#12002=CARTESIAN_POINT('Ctrl Pts',(0.294436598957663,-7.4345263672356,-0.140599465120536));
#12003=CARTESIAN_POINT('Ctrl Pts',(0.133626808785089,-7.66462925468784,
-0.156299477855761));
#12004=CARTESIAN_POINT('Ctrl Pts',(-0.147007075457338,-7.65743695432686,
-0.171999490590986));
#12005=CARTESIAN_POINT('Ctrl Pts',(-0.295818476990691,-7.41939826720899,
-0.187699503326212));
#12006=CARTESIAN_POINT('Ctrl Pts',(-0.179366526901941,-7.16396506696649,
-0.203399516061437));
#12007=CARTESIAN_POINT('Ctrl Pts',(0.0979250663144644,-7.12018660642628,
-0.219099528796662));
#12008=CARTESIAN_POINT('Ctrl Pts',(0.287406334089916,-7.32731952468401,
-0.234799541531888));
#12009=CARTESIAN_POINT('Ctrl Pts',(0.219167574438337,-7.59962571034071,
-0.250499554267113));
#12010=CARTESIAN_POINT('Ctrl Pts',(-0.0456008466565794,-7.69292561240175,
-0.266199567002338));
#12011=CARTESIAN_POINT('Ctrl Pts',(-0.269478553634763,-7.52355630465202,
-0.281899579737564));
#12012=CARTESIAN_POINT('Ctrl Pts',(-0.251712255041962,-7.24339287464728,
-0.297599592472789));
#12013=CARTESIAN_POINT('Ctrl Pts',(-0.00823316316280154,-7.10366055563705,
-0.313299605208015));
#12014=CARTESIAN_POINT('Ctrl Pts',(0.242628685420975,-7.2296586597015,-0.32899961794324));
#12015=CARTESIAN_POINT('Ctrl Pts',(0.275923063959457,-7.50840347761142,
-0.344699630678465));
#12016=CARTESIAN_POINT('Ctrl Pts',(0.0617945840355804,-7.68994185726368,
-0.36039964341369));
#12017=CARTESIAN_POINT('Ctrl Pts',(-0.207745692260543,-7.61148659188026,
-0.376099656148916));
#12018=CARTESIAN_POINT('Ctrl Pts',(-0.290998413267463,-7.34338927068337,
-0.391799668884141));
#12019=CARTESIAN_POINT('Ctrl Pts',(-0.113310065391281,-7.12605533352397,
-0.407499681619367));
#12020=CARTESIAN_POINT('Ctrl Pts',(0.165984505167137,-7.1543702069629,-0.423199694354592));
#12021=CARTESIAN_POINT('Ctrl Pts',(0.296439177569342,-7.40294367216451,
-0.438899707089817));
#12022=CARTESIAN_POINT('Ctrl Pts',(0.161073995511965,-7.64887751853234,
-0.454599719825043));
#12023=CARTESIAN_POINT('Ctrl Pts',(-0.118727783543868,-7.67164050593443,
-0.470299732560267));
#12024=CARTESIAN_POINT('Ctrl Pts',(-0.292065220177002,-7.4508208466213,
-0.485999745295493));
#12025=CARTESIAN_POINT('Ctrl Pts',(-0.203504971720617,-7.18442964465928,
-0.501699758030718));
#12026=CARTESIAN_POINT('Ctrl Pts',(0.0675401367921992,-7.11134245231363,
-0.517399770765944));
#12027=CARTESIAN_POINT('Ctrl Pts',(0.278021357547625,-7.29709724437831,
-0.533099783501169));
#12028=CARTESIAN_POINT('Ctrl Pts',(0.239198158049331,-7.57512594045925,
-0.548799796236395));
#12029=CARTESIAN_POINT('Ctrl Pts',(-0.0141163210559342,-7.69611749368257,
-0.56449980897162));
#12030=CARTESIAN_POINT('Ctrl Pts',(-0.25477256666277,-7.55157771398154,
-0.580199821706845));
#12031=CARTESIAN_POINT('Ctrl Pts',(-0.26697179340797,-7.2711166139018,-0.595899834442071));
#12032=CARTESIAN_POINT('Ctrl Pts',(-0.0397748803529979,-7.10622674499603,
-0.611599847177296));
#12033=CARTESIAN_POINT('Ctrl Pts',(0.223088607111123,-7.20476564283543,
-0.627299859912521));
#12034=CARTESIAN_POINT('Ctrl Pts',(0.285906284140895,-7.47837412958179,
-0.642999872647747));
#12035=CARTESIAN_POINT('Ctrl Pts',(0.0923492877737298,-7.68170162831085,
-0.658699885382972));
#12036=CARTESIAN_POINT('Ctrl Pts',(-0.184018673854838,-7.63242891988962,
-0.674399898118197));
#12037=CARTESIAN_POINT('Ctrl Pts',(-0.295374371161713,-7.37472620315649,
-0.690099910853423));
#12038=CARTESIAN_POINT('Ctrl Pts',(-0.141866960788195,-7.13970442601869,
-0.705799923588648));
#12039=CARTESIAN_POINT('Ctrl Pts',(0.138857796721408,-7.13805651442501,
-0.721499936323874));
#12040=CARTESIAN_POINT('Ctrl Pts',(0.295059605844517,-7.37136780611577,
-0.737199949059099));
#12041=CARTESIAN_POINT('Ctrl Pts',(0.186694406342068,-7.63020861578915,
-0.752899961794324));
#12042=CARTESIAN_POINT('Ctrl Pts',(-0.0891128186061158,-7.68291323570534,
-0.76859997452955));
#12043=CARTESIAN_POINT('Ctrl Pts',(-0.284951629803116,-7.48132145777293,
-0.784299987264774));
#12044=CARTESIAN_POINT('Ctrl Pts',(-0.245141179607853,-7.29931992554818,
-0.794766662421592));
#12045=CARTESIAN_POINT('Ctrl Pts',(-0.191346599666506,-7.23640127966251,
-0.8));
#12046=CARTESIAN_POINT('Ctrl Pts',(-0.191346599666506,-7.23640127966251,
-0.8));
#12047=CARTESIAN_POINT('Ctrl Pts',(-0.202509812150815,-7.24689195824451,
-0.8));
#12048=CARTESIAN_POINT('Ctrl Pts',(-0.21257001858597,-7.25841324529628,
-0.8));
#12049=CARTESIAN_POINT('Ctrl Pts',(-0.2215222854557,-7.27074763835105,-0.8));
#12050=CARTESIAN_POINT('Ctrl Pts',(-0.229528851949894,-7.28177904967911,
-0.8));
#12051=CARTESIAN_POINT('Ctrl Pts',(-0.236649218441325,-7.29346217849914,
-0.8));
#12052=CARTESIAN_POINT('Ctrl Pts',(-0.242860433713407,-7.30566893142592,
-0.8));
#12053=CARTESIAN_POINT('Ctrl Pts',(-0.244940810611317,-7.30975744642258,
-0.8));
#12054=CARTESIAN_POINT('Ctrl Pts',(-0.246919675168011,-7.31390635200313,
-0.8));
#12055=CARTESIAN_POINT('Ctrl Pts',(-0.248793541339973,-7.31810664328013,
-0.8));
#12056=CARTESIAN_POINT('Ctrl Pts',(-0.255493751071069,-7.33312523580754,
-0.8));
#12057=CARTESIAN_POINT('Ctrl Pts',(-0.260811073903805,-7.34869792479653,
-0.8));
#12058=CARTESIAN_POINT('Ctrl Pts',(-0.264722800485284,-7.36459862853377,
-0.8));
#12059=CARTESIAN_POINT('Ctrl Pts',(-0.267427531006873,-7.37559303671058,
-0.8));
#12060=CARTESIAN_POINT('Ctrl Pts',(-0.269459584929932,-7.38674533385887,
-0.8));
#12061=CARTESIAN_POINT('Ctrl Pts',(-0.270799630246209,-7.39798910408356,
-0.8));
#12062=CARTESIAN_POINT('Ctrl Pts',(-0.271554584183732,-7.40432361270102,
-0.8));
#12063=CARTESIAN_POINT('Ctrl Pts',(-0.272089709263086,-7.41068724824774,
-0.8));
#12064=CARTESIAN_POINT('Ctrl Pts',(-0.272399954519056,-7.41706856176779,
-0.8));
#12065=CARTESIAN_POINT('Ctrl Pts',(-0.272610215830843,-7.42139334458343,
-0.8));
#12066=CARTESIAN_POINT('Ctrl Pts',(-0.272716688467774,-7.42571717942635,
-0.8));
#12067=CARTESIAN_POINT('Ctrl Pts',(-0.272718878845034,-7.43003460508684,
-0.8));
#12068=CARTESIAN_POINT('Ctrl Pts',(-0.272726877365373,-7.44580039008993,
-0.8));
#12069=CARTESIAN_POINT('Ctrl Pts',(-0.271347528745165,-7.46148685548989,
-0.8));
#12070=CARTESIAN_POINT('Ctrl Pts',(-0.268538072982214,-7.47691819603078,
-0.8));
#12071=CARTESIAN_POINT('Ctrl Pts',(-0.266219589118033,-7.48965280268256,
-0.8));
#12072=CARTESIAN_POINT('Ctrl Pts',(-0.26292668789853,-7.5022143616876,-0.8));
#12073=CARTESIAN_POINT('Ctrl Pts',(-0.258732571736959,-7.51453557833684,
-0.8));
#12074=CARTESIAN_POINT('Ctrl Pts',(-0.256787738588096,-7.52024898961365,
-0.8));
#12075=CARTESIAN_POINT('Ctrl Pts',(-0.254646822394779,-7.52591466429966,
-0.8));
#12076=CARTESIAN_POINT('Ctrl Pts',(-0.252327841578967,-7.53149910592954,
-0.8));
#12077=CARTESIAN_POINT('Ctrl Pts',(-0.245813410497626,-7.54718679936692,
-0.8));
#12078=CARTESIAN_POINT('Ctrl Pts',(-0.237886859352545,-7.56227243122225,
-0.8));
#12079=CARTESIAN_POINT('Ctrl Pts',(-0.228725832616534,-7.57661351587103,
-0.8));
#12080=CARTESIAN_POINT('Ctrl Pts',(-0.223374474548107,-7.58499077327424,
-0.8));
#12081=CARTESIAN_POINT('Ctrl Pts',(-0.217600846214963,-7.59311397793835,
-0.8));
#12082=CARTESIAN_POINT('Ctrl Pts',(-0.21143274247831,-7.60095296973045,
-0.8));
#12083=CARTESIAN_POINT('Ctrl Pts',(-0.20742008137373,-7.60605262738963,
-0.8));
#12084=CARTESIAN_POINT('Ctrl Pts',(-0.203240363216825,-7.61103196707157,
-0.8));
#12085=CARTESIAN_POINT('Ctrl Pts',(-0.19890016925924,-7.6158820614063,-0.8));
#12086=CARTESIAN_POINT('Ctrl Pts',(-0.195670588103427,-7.61949106446479,
-0.8));
#12087=CARTESIAN_POINT('Ctrl Pts',(-0.192354860452395,-7.62302525643464,
-0.8));
#12088=CARTESIAN_POINT('Ctrl Pts',(-0.188961839362612,-7.62647560355552,
-0.8));
#12089=CARTESIAN_POINT('Ctrl Pts',(-0.179751748624594,-7.63584130132751,
-0.8));
#12090=CARTESIAN_POINT('Ctrl Pts',(-0.169961500633801,-7.64460282207988,
-0.8));
#12091=CARTESIAN_POINT('Ctrl Pts',(-0.159654451890089,-7.65269298880017,
-0.8));
#12092=CARTESIAN_POINT('Ctrl Pts',(-0.154923544879998,-7.656406353062,-0.8));
#12093=CARTESIAN_POINT('Ctrl Pts',(-0.150083579318515,-7.65997817804833,
-0.8));
#12094=CARTESIAN_POINT('Ctrl Pts',(-0.145139853312966,-7.66340132998996,
-0.8));
#12095=CARTESIAN_POINT('Ctrl Pts',(-0.13997839750837,-7.66697524315572,
-0.8));
#12096=CARTESIAN_POINT('Ctrl Pts',(-0.134710287969361,-7.67038248469088,
-0.8));
#12097=CARTESIAN_POINT('Ctrl Pts',(-0.129347191444159,-7.67361284285922,
-0.8));
#12098=CARTESIAN_POINT('Ctrl Pts',(-0.117405249048123,-7.68080584246004,
-0.8));
#12099=CARTESIAN_POINT('Ctrl Pts',(-0.104985860997357,-7.68712785830345,
-0.8));
#12100=CARTESIAN_POINT('Ctrl Pts',(-0.0921567961212457,-7.69249315468034,
-0.8));
#12101=CARTESIAN_POINT('Ctrl Pts',(-0.0880066881472035,-7.69422878853143,
-0.8));
#12102=CARTESIAN_POINT('Ctrl Pts',(-0.0838136142204832,-7.69586419339144,
-0.8));
#12103=CARTESIAN_POINT('Ctrl Pts',(-0.0795809211152283,-7.69740029063291,
-0.8));
#12104=CARTESIAN_POINT('Ctrl Pts',(-0.251593604700942,-7.39979879766985,
-0.0887416697508022));
#12105=CARTESIAN_POINT('Ctrl Pts',(-0.251789073617808,-7.37467806093596,
-0.090327588805488));
#12106=CARTESIAN_POINT('Ctrl Pts',(-0.248321652469561,-7.3496099888614,
-0.0919135078601738));
#12107=CARTESIAN_POINT('Ctrl Pts',(-0.240965812307516,-7.32574031936136,
-0.0934994269148596));
#12108=CARTESIAN_POINT('Ctrl Pts',(-0.216692445626501,-7.24697334950268,
-0.0987327644932681));
#12109=CARTESIAN_POINT('Ctrl Pts',(-0.150077356231607,-7.18125600966837,
-0.103966102071677));
#12110=CARTESIAN_POINT('Ctrl Pts',(-0.0709891728117581,-7.15805131825776,
-0.109199439650085));
#12111=CARTESIAN_POINT('Ctrl Pts',(0.00809901060809128,-7.13484662684715,
-0.114432777228494));
#12112=CARTESIAN_POINT('Ctrl Pts',(0.0996602880528962,-7.15415458386024,
-0.119666114806902));
#12113=CARTESIAN_POINT('Ctrl Pts',(0.162643432351959,-7.20731920009383,
-0.12489945238531));
#12114=CARTESIAN_POINT('Ctrl Pts',(0.225626576651022,-7.26048381632742,
-0.130132789963719));
#12115=CARTESIAN_POINT('Ctrl Pts',(0.260031587804342,-7.34750509178151,
-0.135366127542127));
#12116=CARTESIAN_POINT('Ctrl Pts',(0.250432461685574,-7.4293662107506,-0.140599465120536));
#12117=CARTESIAN_POINT('Ctrl Pts',(0.240833335566805,-7.51122732971968,
-0.145832802698944));
#12118=CARTESIAN_POINT('Ctrl Pts',(0.187230072175947,-7.58792829220376,
-0.151066140277353));
#12119=CARTESIAN_POINT('Ctrl Pts',(0.113656126440114,-7.62508005671897,
-0.156299477855761));
#12120=CARTESIAN_POINT('Ctrl Pts',(0.0400821807042802,-7.66223182123418,
-0.161532815434169));
#12121=CARTESIAN_POINT('Ctrl Pts',(-0.0534624473765288,-7.65983438778052,
-0.166766153012578));
#12122=CARTESIAN_POINT('Ctrl Pts',(-0.125036661672492,-7.61896255653404,
-0.171999490590986));
#12123=CARTESIAN_POINT('Ctrl Pts',(-0.196610875968456,-7.57809072528757,
-0.177232828169395));
#12124=CARTESIAN_POINT('Ctrl Pts',(-0.246214676479574,-7.49874449624828,
-0.182466165747803));
#12125=CARTESIAN_POINT('Ctrl Pts',(-0.251607918387007,-7.41649918168822,
-0.187699503326212));
#12126=CARTESIAN_POINT('Ctrl Pts',(-0.251965921640279,-7.41103973991196,
-0.188046892134409));
#12127=CARTESIAN_POINT('Ctrl Pts',(-0.252129119871954,-7.40556752389274,
-0.188394280942605));
#12128=CARTESIAN_POINT('Ctrl Pts',(-0.252102603566075,-7.4000936994049,
-0.188741669750802));
#12129=CARTESIAN_POINT('Ctrl Pts',(-0.0793799282532839,-7.69692229537457,
2.77555756156289E-17));
#12130=CARTESIAN_POINT('Ctrl Pts',(-0.0961911494322625,-7.69077267557206,
2.35324001622483E-17));
#12131=CARTESIAN_POINT('Ctrl Pts',(-0.112330835541762,-7.68307124215404,
-2.1766246802835E-17));
#12132=CARTESIAN_POINT('Ctrl Pts',(-0.127669379580378,-7.67400023063824,
-1.34441069388203E-17));
#12133=CARTESIAN_POINT('Ctrl Pts',(-0.13764508202298,-7.66810073251721,
-8.03165118290813E-18));
#12134=CARTESIAN_POINT('Ctrl Pts',(-0.147281472230525,-7.66162083730929,
2.61489825013166E-18));
#12135=CARTESIAN_POINT('Ctrl Pts',(-0.156535274241645,-7.65460205458247,
8.67361737988404E-18));
#12136=CARTESIAN_POINT('Ctrl Pts',(-0.163949010525728,-7.64897891675118,
1.35275947821813E-17));
#12137=CARTESIAN_POINT('Ctrl Pts',(-0.171117084588845,-7.64300974124484,
7.79481809193044E-17));
#12138=CARTESIAN_POINT('Ctrl Pts',(-0.178013579433405,-7.63671391029203,
9.36750677027476E-17));
#12139=CARTESIAN_POINT('Ctrl Pts',(-0.181540539144798,-7.63349413812939,
1.01718007967481E-16));
#12140=CARTESIAN_POINT('Ctrl Pts',(-0.184990139201544,-7.63019455138719,
-3.81961123697981E-17));
#12141=CARTESIAN_POINT('Ctrl Pts',(-0.188356661978096,-7.6268214388693,
-3.38271077815477E-17));
#12142=CARTESIAN_POINT('Ctrl Pts',(-0.200715886255777,-7.61443802224343,
-1.77875586204687E-17));
#12143=CARTESIAN_POINT('Ctrl Pts',(-0.211972714988144,-7.60105293520862,
2.70635579723243E-17));
#12144=CARTESIAN_POINT('Ctrl Pts',(-0.221976934246241,-7.58681399582591,
-1.73472347597681E-18));
#12145=CARTESIAN_POINT('Ctrl Pts',(-0.228265887851312,-7.57786296957857,
-1.98381907493045E-17));
#12146=CARTESIAN_POINT('Ctrl Pts',(-0.234059032429037,-7.56857391909213,
2.8705858906042E-18));
#12147=CARTESIAN_POINT('Ctrl Pts',(-0.239308868459768,-7.55898027773993,
-3.46944695195361E-18));
#12148=CARTESIAN_POINT('Ctrl Pts',(-0.241553631081729,-7.55487815961855,
-6.18036376224402E-18));
#12149=CARTESIAN_POINT('Ctrl Pts',(-0.243698951449468,-7.55072033678723,
4.51101226057749E-17));
#12150=CARTESIAN_POINT('Ctrl Pts',(-0.245740602454379,-7.54650938813658,
4.85722573273506E-17));
#12151=CARTESIAN_POINT('Ctrl Pts',(-0.247686917822847,-7.54249507126515,
5.1872726408548E-17));
#12152=CARTESIAN_POINT('Ctrl Pts',(-0.249535103186422,-7.53844047081111,
8.10072286248015E-17));
#12153=CARTESIAN_POINT('Ctrl Pts',(-0.251281761611404,-7.53435006699437,
7.45931094670027E-17));
#12154=CARTESIAN_POINT('Ctrl Pts',(-0.2575376047831,-7.51969985008849,5.16202585868036E-17));
#12155=CARTESIAN_POINT('Ctrl Pts',(-0.262498407735628,-7.5045827269486,
3.19807068830928E-17));
#12156=CARTESIAN_POINT('Ctrl Pts',(-0.266024752279042,-7.4891086692212,
5.55111512312578E-17));
#12157=CARTESIAN_POINT('Ctrl Pts',(-0.268541669693304,-7.47806410880349,
6.90752738671573E-17));
#12158=CARTESIAN_POINT('Ctrl Pts',(-0.270326748263048,-7.46683731032382,
1.98990298923518E-18));
#12159=CARTESIAN_POINT('Ctrl Pts',(-0.271391863481061,-7.4554970632839,
0.));
#12160=CARTESIAN_POINT('Ctrl Pts',(-0.271805184633354,-7.45109644643555,
-7.72187818324019E-19));
#12161=CARTESIAN_POINT('Ctrl Pts',(-0.272109983012601,-7.44667877563548,
3.18736603349747E-17));
#12162=CARTESIAN_POINT('Ctrl Pts',(-0.272306561259532,-7.44224822959102,
3.12250225675825E-17));
#12163=CARTESIAN_POINT('Ctrl Pts',(-0.272509061253092,-7.43768421724747,
3.05568451584854E-17));
#12164=CARTESIAN_POINT('Ctrl Pts',(-0.27259626110233,-7.43311633646646,
7.03447662139463E-17));
#12165=CARTESIAN_POINT('Ctrl Pts',(-0.272569835270061,-7.42855113569005,
7.28583859910259E-17));
#12166=CARTESIAN_POINT('Ctrl Pts',(-0.272471756407933,-7.41160749913858,
8.21876273579062E-17));
#12167=CARTESIAN_POINT('Ctrl Pts',(-0.270813099881604,-7.39468986571343,
2.72914138058113E-17));
#12168=CARTESIAN_POINT('Ctrl Pts',(-0.267648465653111,-7.37802926095779,
-1.73472347597681E-17));
#12169=CARTESIAN_POINT('Ctrl Pts',(-0.265994330828014,-7.36932086543916,
-4.06795815039127E-17));
#12170=CARTESIAN_POINT('Ctrl Pts',(-0.263927841897732,-7.36068292366611,
3.71040643002486E-17));
#12171=CARTESIAN_POINT('Ctrl Pts',(-0.261451406717338,-7.35215143569316,
5.20417042793042E-17));
#12172=CARTESIAN_POINT('Ctrl Pts',(-0.260001090669275,-7.34715499806419,
6.07898835788593E-17));
#12173=CARTESIAN_POINT('Ctrl Pts',(-0.25840951525882,-7.34219346234189,
1.85022084656224E-17));
#12174=CARTESIAN_POINT('Ctrl Pts',(-0.256678509151567,-7.33727981648105,
2.42861286636753E-17));
#12175=CARTESIAN_POINT('Ctrl Pts',(-0.251357961519984,-7.32217687332112,
4.20640110073944E-17));
#12176=CARTESIAN_POINT('Ctrl Pts',(-0.244748745096942,-7.30759378918613,
6.42002344202532E-17));
#12177=CARTESIAN_POINT('Ctrl Pts',(-0.236874436022921,-7.29374513935771,
2.77555756156289E-17));
#12178=CARTESIAN_POINT('Ctrl Pts',(-0.23280784441881,-7.28659317178936,
8.9341727323557E-18));
#12179=CARTESIAN_POINT('Ctrl Pts',(-0.228399168283279,-7.27963277931266,
6.23483830602166E-17));
#12180=CARTESIAN_POINT('Ctrl Pts',(-0.223669100108808,-7.27292514415603,
4.16333634234434E-17));
#12181=CARTESIAN_POINT('Ctrl Pts',(-0.216422974570852,-7.2626495276924,
9.89943755332752E-18));
#12182=CARTESIAN_POINT('Ctrl Pts',(-0.208418205701992,-7.25295421133118,
-3.20573011646789E-17));
#12183=CARTESIAN_POINT('Ctrl Pts',(-0.199658657126578,-7.24395737740928,
-3.46944695195361E-17));
#12184=CARTESIAN_POINT('Ctrl Pts',(-0.197072119679919,-7.24130077385944,
-2.85083271403733E-17));
#12185=CARTESIAN_POINT('Ctrl Pts',(-0.194419679127491,-7.23870521167385,
-2.14915623890787E-17));
#12186=CARTESIAN_POINT('Ctrl Pts',(-0.1917040502342,-7.23617187785139,-2.08166817117217E-17));
#12187=CARTESIAN_POINT('Origin',(0.,0.,-0.8));
#12188=CARTESIAN_POINT('',(-8.2,-1.00421037530083E-15,-0.8));
#12189=CARTESIAN_POINT('Origin',(0.,0.,-0.8));
#12190=CARTESIAN_POINT('',(-3.5,-4.28626379701574E-16,-0.8));
#12191=CARTESIAN_POINT('Origin',(0.,0.,-0.8));
#12192=CARTESIAN_POINT('Ctrl Pts',(-0.191346599666504,7.5635987203375,-0.8));
#12193=CARTESIAN_POINT('Ctrl Pts',(-0.20250980500676,7.55310804846915,-0.8));
#12194=CARTESIAN_POINT('Ctrl Pts',(-0.212570003446807,7.5415867670429,-0.8));
#12195=CARTESIAN_POINT('Ctrl Pts',(-0.221522262311368,7.52925237897662,
-0.8));
#12196=CARTESIAN_POINT('Ctrl Pts',(-0.229528852882395,7.51822092907276,
-0.8));
#12197=CARTESIAN_POINT('Ctrl Pts',(-0.236649236537895,7.50653775609482,
-0.8));
#12198=CARTESIAN_POINT('Ctrl Pts',(-0.242860462351933,7.49433095521787,
-0.8));
#12199=CARTESIAN_POINT('Ctrl Pts',(-0.244940827324234,7.49024245453724,
-0.8));
#12200=CARTESIAN_POINT('Ctrl Pts',(-0.24691968074903,7.48609356366845,-0.8));
#12201=CARTESIAN_POINT('Ctrl Pts',(-0.248793536546706,7.48189328763567,
-0.8));
#12202=CARTESIAN_POINT('Ctrl Pts',(-0.255493735434215,7.46687469077406,
-0.8));
#12203=CARTESIAN_POINT('Ctrl Pts',(-0.260811047538467,7.45130199730205,
-0.8));
#12204=CARTESIAN_POINT('Ctrl Pts',(-0.264722764385489,7.43540128965534,
-0.8));
#12205=CARTESIAN_POINT('Ctrl Pts',(-0.267427485323018,7.42440689037352,
-0.8));
#12206=CARTESIAN_POINT('Ctrl Pts',(-0.269459531552823,7.41325460272601,
-0.8));
#12207=CARTESIAN_POINT('Ctrl Pts',(-0.270799571424799,7.40201084264177,
-0.8));
#12208=CARTESIAN_POINT('Ctrl Pts',(-0.271554526921096,7.39567630092241,
-0.8));
#12209=CARTESIAN_POINT('Ctrl Pts',(-0.272089651581207,7.38931263212047,
-0.8));
#12210=CARTESIAN_POINT('Ctrl Pts',(-0.272399894416452,7.38293128541091,
-0.8));
#12211=CARTESIAN_POINT('Ctrl Pts',(-0.272610151901875,7.37860652506082,
-0.8));
#12212=CARTESIAN_POINT('Ctrl Pts',(-0.272716621945222,7.37428271302943,
-0.8));
#12213=CARTESIAN_POINT('Ctrl Pts',(-0.27271881100291,7.36996531010121,-0.8));
#12214=CARTESIAN_POINT('Ctrl Pts',(-0.272726804747392,7.35419952374042,
-0.8));
#12215=CARTESIAN_POINT('Ctrl Pts',(-0.271347453373968,7.33851305838944,
-0.8));
#12216=CARTESIAN_POINT('Ctrl Pts',(-0.268537997639155,7.32308171994473,
-0.8));
#12217=CARTESIAN_POINT('Ctrl Pts',(-0.266219513087219,7.31034711111768,
-0.8));
#12218=CARTESIAN_POINT('Ctrl Pts',(-0.262926612476523,7.29778555143682,
-0.8));
#12219=CARTESIAN_POINT('Ctrl Pts',(-0.258732497897385,7.28546433529152,
-0.8));
#12220=CARTESIAN_POINT('Ctrl Pts',(-0.256787665913683,7.27975092551567,
-0.8));
#12221=CARTESIAN_POINT('Ctrl Pts',(-0.254646751184067,7.27408525256649,
-0.8));
#12222=CARTESIAN_POINT('Ctrl Pts',(-0.252327772084624,7.26850081285998,
-0.8));
#12223=CARTESIAN_POINT('Ctrl Pts',(-0.24581334288864,7.25281311775483,-0.8));
#12224=CARTESIAN_POINT('Ctrl Pts',(-0.237886794345816,7.23772748623907,
-0.8));
#12225=CARTESIAN_POINT('Ctrl Pts',(-0.228725770337881,7.22338640333096,
-0.8));
#12226=CARTESIAN_POINT('Ctrl Pts',(-0.223374411591948,7.21500914338927,
-0.8));
#12227=CARTESIAN_POINT('Ctrl Pts',(-0.217600782266579,7.20688593688198,
-0.8));
#12228=CARTESIAN_POINT('Ctrl Pts',(-0.211432677139281,7.19904694387202,
-0.8));
#12229=CARTESIAN_POINT('Ctrl Pts',(-0.207419991121397,7.1939472549082,-0.8));
#12230=CARTESIAN_POINT('Ctrl Pts',(-0.203240245884041,7.18896788562565,
-0.8));
#12231=CARTESIAN_POINT('Ctrl Pts',(-0.198900022769198,7.1841177635399,-0.8));
#12232=CARTESIAN_POINT('Ctrl Pts',(-0.195670399400898,7.18050871690502,
-0.8));
#12233=CARTESIAN_POINT('Ctrl Pts',(-0.192354627608631,7.17697448367564,
-0.8));
#12234=CARTESIAN_POINT('Ctrl Pts',(-0.188961560346599,7.17352409745826,
-0.8));
#12235=CARTESIAN_POINT('Ctrl Pts',(-0.179751438686603,7.16415838956568,
-0.8));
#12236=CARTESIAN_POINT('Ctrl Pts',(-0.169961157096887,7.15539686266801,
-0.8));
#12237=CARTESIAN_POINT('Ctrl Pts',(-0.159654072168358,7.14730669411858,
-0.8));
#12238=CARTESIAN_POINT('Ctrl Pts',(-0.154924675023346,7.14359452716685,
-0.8));
#12239=CARTESIAN_POINT('Ctrl Pts',(-0.150086289122297,7.14002380910476,
-0.8));
#12240=CARTESIAN_POINT('Ctrl Pts',(-0.145144207522002,7.13660166676285,
-0.8));
#12241=CARTESIAN_POINT('Ctrl Pts',(-0.139981536349868,7.13302677726397,
-0.8));
#12242=CARTESIAN_POINT('Ctrl Pts',(-0.13471214767354,7.1296186339709,-0.8));
#12243=CARTESIAN_POINT('Ctrl Pts',(-0.129347728154467,7.12638746410443,
-0.8));
#12244=CARTESIAN_POINT('Ctrl Pts',(-0.11740562697242,7.11919433587414,-0.8));
#12245=CARTESIAN_POINT('Ctrl Pts',(-0.104986064106116,7.11287221540064,
-0.8));
#12246=CARTESIAN_POINT('Ctrl Pts',(-0.0921568111370747,7.10750684175833,
-0.8));
#12247=CARTESIAN_POINT('Ctrl Pts',(-0.088006704056484,7.10577120873303,
-0.8));
#12248=CARTESIAN_POINT('Ctrl Pts',(-0.0838136309060128,7.10413580458697,
-0.8));
#12249=CARTESIAN_POINT('Ctrl Pts',(-0.0795809384672947,7.10259970795555,
-0.8));
#12250=CARTESIAN_POINT('Ctrl Pts',(0.0793799282532802,7.10307770462543,
-0.8));
#12251=CARTESIAN_POINT('Ctrl Pts',(0.0961911602327611,7.10922732837881,
-0.8));
#12252=CARTESIAN_POINT('Ctrl Pts',(0.112330857379334,7.11692876061935,-0.8));
#12253=CARTESIAN_POINT('Ctrl Pts',(0.127669412008062,7.12599976803891,-0.8));
#12254=CARTESIAN_POINT('Ctrl Pts',(0.137645134844041,7.13189927148307,-0.8));
#12255=CARTESIAN_POINT('Ctrl Pts',(0.14728154433848,7.13837917234721,-0.8));
#12256=CARTESIAN_POINT('Ctrl Pts',(0.156535364142904,7.14539796150249,-0.8));
#12257=CARTESIAN_POINT('Ctrl Pts',(0.163949176913172,7.1510211516846,-0.8));
#12258=CARTESIAN_POINT('Ctrl Pts',(0.171117322384025,7.15699038584565,-0.8));
#12259=CARTESIAN_POINT('Ctrl Pts',(0.178013882658357,7.16328628151714,-0.8));
#12260=CARTESIAN_POINT('Ctrl Pts',(0.181540759565318,7.16650598063802,-0.8));
#12261=CARTESIAN_POINT('Ctrl Pts',(0.184990279464215,7.16980548981786,-0.8));
#12262=CARTESIAN_POINT('Ctrl Pts',(0.188356726173562,7.17317852169621,-0.8));
#12263=CARTESIAN_POINT('Ctrl Pts',(0.200715946303584,7.18556191792655,-0.8));
#12264=CARTESIAN_POINT('Ctrl Pts',(0.211972771450931,7.19894698292655,-0.8));
#12265=CARTESIAN_POINT('Ctrl Pts',(0.221976987368764,7.21318590122467,-0.8));
#12266=CARTESIAN_POINT('Ctrl Pts',(0.228265932818091,7.22213690559821,-0.8));
#12267=CARTESIAN_POINT('Ctrl Pts',(0.234059070290878,7.231425933934,-0.8));
#12268=CARTESIAN_POINT('Ctrl Pts',(0.239308900334691,7.24101955361731,-0.8));
#12269=CARTESIAN_POINT('Ctrl Pts',(0.241553661905442,7.24512166523041,-0.8));
#12270=CARTESIAN_POINT('Ctrl Pts',(0.243698981293207,7.24927948171673,-0.8));
#12271=CARTESIAN_POINT('Ctrl Pts',(0.245740631388171,7.25349042424184,-0.8));
#12272=CARTESIAN_POINT('Ctrl Pts',(0.247686947093964,7.25750473775864,-0.8));
#12273=CARTESIAN_POINT('Ctrl Pts',(0.249535132735624,7.26155933511193,-0.8));
#12274=CARTESIAN_POINT('Ctrl Pts',(0.251281791380746,7.26564973614279,-0.8));
#12275=CARTESIAN_POINT('Ctrl Pts',(0.257537634638496,7.2802999414258,-0.8));
#12276=CARTESIAN_POINT('Ctrl Pts',(0.262498437191553,7.29541705678458,-0.8));
#12277=CARTESIAN_POINT('Ctrl Pts',(0.266024780552404,7.31089111260971,-0.8));
#12278=CARTESIAN_POINT('Ctrl Pts',(0.268541696557213,7.32193566918861,-0.8));
#12279=CARTESIAN_POINT('Ctrl Pts',(0.270326773646181,7.33316246674896,-0.8));
#12280=CARTESIAN_POINT('Ctrl Pts',(0.271391887422382,7.34450271522912,-0.8));
#12281=CARTESIAN_POINT('Ctrl Pts',(0.271805207529464,7.348903327465,-0.8));
#12282=CARTESIAN_POINT('Ctrl Pts',(0.272110005124503,7.353320993968,-0.8));
#12283=CARTESIAN_POINT('Ctrl Pts',(0.272306582854207,7.35775153601331,-0.8));
#12284=CARTESIAN_POINT('Ctrl Pts',(0.272509082926936,7.36231555803023,-0.8));
#12285=CARTESIAN_POINT('Ctrl Pts',(0.272596282445522,7.3668834489416,-0.8));
#12286=CARTESIAN_POINT('Ctrl Pts',(0.272569855883151,7.37144866009378,-0.8));
#12287=CARTESIAN_POINT('Ctrl Pts',(0.27247177445576,7.3883923101935,-0.8));
#12288=CARTESIAN_POINT('Ctrl Pts',(0.27081311450216,7.40530996127497,-0.8));
#12289=CARTESIAN_POINT('Ctrl Pts',(0.267648476420034,7.42197058557661,-0.8));
#12290=CARTESIAN_POINT('Ctrl Pts',(0.265994356074714,7.43067890447688,-0.8));
#12291=CARTESIAN_POINT('Ctrl Pts',(0.263927889725214,7.43931677154928,-0.8));
#12292=CARTESIAN_POINT('Ctrl Pts',(0.261451485232966,7.447848187512,-0.8));
#12293=CARTESIAN_POINT('Ctrl Pts',(0.260001161760158,7.45284467046369,-0.8));
#12294=CARTESIAN_POINT('Ctrl Pts',(0.258409576835351,7.45780625101157,-0.8));
#12295=CARTESIAN_POINT('Ctrl Pts',(0.256678558962749,7.46271994144919,-0.8));
#12296=CARTESIAN_POINT('Ctrl Pts',(0.251358016236622,7.47782290504656,-0.8));
#12297=CARTESIAN_POINT('Ctrl Pts',(0.244748805012871,7.49240601029322,-0.8));
#12298=CARTESIAN_POINT('Ctrl Pts',(0.23687450191739,7.50625468017588,-0.8));
#12299=CARTESIAN_POINT('Ctrl Pts',(0.232807882388933,7.51340671264214,-0.8));
#12300=CARTESIAN_POINT('Ctrl Pts',(0.228399173295155,7.5203671668612,-0.8));
#12301=CARTESIAN_POINT('Ctrl Pts',(0.223669067490228,7.5270748591468,-0.8));
#12302=CARTESIAN_POINT('Ctrl Pts',(0.216422943591704,7.53735047905449,-0.8));
#12303=CARTESIAN_POINT('Ctrl Pts',(0.208418177836147,7.5470457976146,-0.8));
#12304=CARTESIAN_POINT('Ctrl Pts',(0.199658634031892,7.55604263170521,-0.8));
#12305=CARTESIAN_POINT('Ctrl Pts',(0.197072096223501,7.55869923712339,-0.8));
#12306=CARTESIAN_POINT('Ctrl Pts',(0.19441965536406,7.56129480091647,-0.8));
#12307=CARTESIAN_POINT('Ctrl Pts',(0.191704026215795,7.56382813610289,-0.8));
#12308=CARTESIAN_POINT('Ctrl Pts',(7.2086534003335,0.163598720337496,-0.8));
#12309=CARTESIAN_POINT('Ctrl Pts',(7.19749017953724,0.153108033944298,-0.8));
#12310=CARTESIAN_POINT('Ctrl Pts',(7.18742996379988,0.141586740347201,-0.8));
#12311=CARTESIAN_POINT('Ctrl Pts',(7.17847768761626,0.129252341488054,-0.8));
#12312=CARTESIAN_POINT('Ctrl Pts',(7.1704711491364,0.118220975043782,-0.8));
#12313=CARTESIAN_POINT('Ctrl Pts',(7.1633508026162,0.106537897602213,-0.8));
#12314=CARTESIAN_POINT('Ctrl Pts',(7.15713959961044,0.0943312004660431,
-0.8));
#12315=CARTESIAN_POINT('Ctrl Pts',(7.15505920883279,0.0902426688041016,
-0.8));
#12316=CARTESIAN_POINT('Ctrl Pts',(7.15308033132025,0.0860937460975511,
-0.8));
#12317=CARTESIAN_POINT('Ctrl Pts',(7.1512064530744,0.0818934370748483,-0.8));
#12318=CARTESIAN_POINT('Ctrl Pts',(7.14450623072875,0.0668748495893196,
-0.8));
#12319=CARTESIAN_POINT('Ctrl Pts',(7.13918889541544,0.0513021658152235,
-0.8));
#12320=CARTESIAN_POINT('Ctrl Pts',(7.13527715751009,0.0354014666253399,
-0.8));
#12321=CARTESIAN_POINT('Ctrl Pts',(7.13257241583995,0.024407048102453,-0.8));
#12322=CARTESIAN_POINT('Ctrl Pts',(7.13054035296786,0.0132547399032318,
-0.8));
#12323=CARTESIAN_POINT('Ctrl Pts',(7.1292003013188,0.00201095788328195,
-0.8));
#12324=CARTESIAN_POINT('Ctrl Pts',(7.1284453491983,-0.00432351219812528,
-0.8));
#12325=CARTESIAN_POINT('Ctrl Pts',(7.12791022363301,-0.010687109030267,
-0.8));
#12326=CARTESIAN_POINT('Ctrl Pts',(7.1275999755608,-0.017068383912153,-0.8));
#12327=CARTESIAN_POINT('Ctrl Pts',(7.12738970979551,-0.0213931928851633,
-0.8));
#12328=CARTESIAN_POINT('Ctrl Pts',(7.12728323414032,-0.0257170542882299,
-0.8));
#12329=CARTESIAN_POINT('Ctrl Pts',(7.12728104222802,-0.0300345064165335,
-0.8));
#12330=CARTESIAN_POINT('Ctrl Pts',(7.12727303815211,-0.0458002898456707,
-0.8));
#12331=CARTESIAN_POINT('Ctrl Pts',(7.12865238357099,-0.0614867553087103,
-0.8));
#12332=CARTESIAN_POINT('Ctrl Pts',(7.1314618393697,-0.0769180982948808,
-0.8));
#12333=CARTESIAN_POINT('Ctrl Pts',(7.13378032243542,-0.0896527024168026,
-0.8));
#12334=CARTESIAN_POINT('Ctrl Pts',(7.13707322436504,-0.102214260636911,
-0.8));
#12335=CARTESIAN_POINT('Ctrl Pts',(7.14126734236948,-0.11453547787408,-0.8));
#12336=CARTESIAN_POINT('Ctrl Pts',(7.14321217687778,-0.120248890906726,
-0.8));
#12337=CARTESIAN_POINT('Ctrl Pts',(7.14535309477846,-0.125914567622866,
-0.8));
#12338=CARTESIAN_POINT('Ctrl Pts',(7.14767207759612,-0.131499011499717,
-0.8));
#12339=CARTESIAN_POINT('Ctrl Pts',(7.15418651087584,-0.147186703000945,
-0.8));
#12340=CARTESIAN_POINT('Ctrl Pts',(7.1621130650536,-0.162272335255616,-0.8));
#12341=CARTESIAN_POINT('Ctrl Pts',(7.17127409496857,-0.176613421933616,
-0.8));
#12342=CARTESIAN_POINT('Ctrl Pts',(7.17662545225571,-0.184990676392116,
-0.8));
#12343=CARTESIAN_POINT('Ctrl Pts',(7.18239907944199,-0.193113878919975,
-0.8));
#12344=CARTESIAN_POINT('Ctrl Pts',(7.18856718156875,-0.200952869302734,
-0.8));
#12345=CARTESIAN_POINT('Ctrl Pts',(7.19257981371173,-0.206052490569052,
-0.8));
#12346=CARTESIAN_POINT('Ctrl Pts',(7.19675950038746,-0.211031795839324,
-0.8));
#12347=CARTESIAN_POINT('Ctrl Pts',(7.20109966044925,-0.215881857912704,
-0.8));
#12348=CARTESIAN_POINT('Ctrl Pts',(7.2043291925446,-0.219490810326305,-0.8));
#12349=CARTESIAN_POINT('Ctrl Pts',(7.20764486889344,-0.22302495434415,-0.8));
#12350=CARTESIAN_POINT('Ctrl Pts',(7.21103783632041,-0.226475256026996,
-0.8));
#12351=CARTESIAN_POINT('Ctrl Pts',(7.22024789111854,-0.235840942038731,
-0.8));
#12352=CARTESIAN_POINT('Ctrl Pts',(7.23003810005691,-0.244602455651909,
-0.8));
#12353=CARTESIAN_POINT('Ctrl Pts',(7.24034510674114,-0.252692620249968,
-0.8));
#12354=CARTESIAN_POINT('Ctrl Pts',(7.24507777505305,-0.256407381169837,
-0.8));
#12355=CARTESIAN_POINT('Ctrl Pts',(7.24991958336186,-0.2599804973403,-0.8));
#12356=CARTESIAN_POINT('Ctrl Pts',(7.25486522766478,-0.263404826892334,
-0.8));
#12357=CARTESIAN_POINT('Ctrl Pts',(7.26002526592285,-0.266977601320589,
-0.8));
#12358=CARTESIAN_POINT('Ctrl Pts',(7.26529188355138,-0.270383791071441,
-0.8));
#12359=CARTESIAN_POINT('Ctrl Pts',(7.27065343703401,-0.27361320247099,-0.8));
#12360=CARTESIAN_POINT('Ctrl Pts',(7.28259519346882,-0.280806051425342,
-0.8));
#12361=CARTESIAN_POINT('Ctrl Pts',(7.29501437679438,-0.287127944728029,
-0.8));
#12362=CARTESIAN_POINT('Ctrl Pts',(7.30784322140636,-0.292493150612868,
-0.8));
#12363=CARTESIAN_POINT('Ctrl Pts',(7.31199333041977,-0.294228785424493,
-0.8));
#12364=CARTESIAN_POINT('Ctrl Pts',(7.3161864052494,-0.295864191114811,-0.8));
#12365=CARTESIAN_POINT('Ctrl Pts',(7.32041909912987,-0.297400289065613,
-0.8));
#12366=CARTESIAN_POINT('Ctrl Pts',(7.47937992825329,-0.29692229537457,-0.8));
#12367=CARTESIAN_POINT('Ctrl Pts',(7.49619115357747,-0.290772674055728,
-0.8));
#12368=CARTESIAN_POINT('Ctrl Pts',(7.5123308439229,-0.283071241089594,-0.8));
#12369=CARTESIAN_POINT('Ctrl Pts',(7.52766939202587,-0.27400023114592,-0.8));
#12370=CARTESIAN_POINT('Ctrl Pts',(7.53764510229467,-0.268100730982278,
-0.8));
#12371=CARTESIAN_POINT('Ctrl Pts',(7.54728149990377,-0.261620833603991,
-0.8));
#12372=CARTESIAN_POINT('Ctrl Pts',(7.55653530874326,-0.254602048410521,
-0.8));
#12373=CARTESIAN_POINT('Ctrl Pts',(7.56394907438075,-0.248978890488539,
-0.8));
#12374=CARTESIAN_POINT('Ctrl Pts',(7.57111717584829,-0.24300969247227,-0.8));
#12375=CARTESIAN_POINT('Ctrl Pts',(7.57801369580309,-0.236713836682386,
-0.8));
#12376=CARTESIAN_POINT('Ctrl Pts',(7.58154062373583,-0.233494092551808,
-0.8));
#12377=CARTESIAN_POINT('Ctrl Pts',(7.58499019302965,-0.230194535576604,
-0.8));
#12378=CARTESIAN_POINT('Ctrl Pts',(7.58835668661318,-0.226821454006683,
-0.8));
#12379=CARTESIAN_POINT('Ctrl Pts',(7.60071590929916,-0.214438045208707,
-0.8));
#12380=CARTESIAN_POINT('Ctrl Pts',(7.61197273665574,-0.201052966631013,
-0.8));
#12381=CARTESIAN_POINT('Ctrl Pts',(7.62197695463197,-0.186814035340863,
-0.8));
#12382=CARTESIAN_POINT('Ctrl Pts',(7.62826590510742,-0.177863017488208,
-0.8));
#12383=CARTESIAN_POINT('Ctrl Pts',(7.63405904695874,-0.16857397550271,-0.8));
#12384=CARTESIAN_POINT('Ctrl Pts',(7.63930888069208,-0.158980342466583,
-0.8));
#12385=CARTESIAN_POINT('Ctrl Pts',(7.64155364292289,-0.154878226820711,
-0.8));
#12386=CARTESIAN_POINT('Ctrl Pts',(7.64369896292573,-0.150720406401628,
-0.8));
#12387=CARTESIAN_POINT('Ctrl Pts',(7.64574061359146,-0.146509460078439,
-0.8));
#12388=CARTESIAN_POINT('Ctrl Pts',(7.64768692907881,-0.142495144513688,
-0.8));
#12389=CARTESIAN_POINT('Ctrl Pts',(7.64953511453937,-0.138440545269517,
-0.8));
#12390=CARTESIAN_POINT('Ctrl Pts',(7.65128177304014,-0.134350142542067,
-0.8));
#12391=CARTESIAN_POINT('Ctrl Pts',(7.65753761624241,-0.119699930101675,
-0.8));
#12392=CARTESIAN_POINT('Ctrl Pts',(7.66249841903988,-0.104582809953302,
-0.8));
#12393=CARTESIAN_POINT('Ctrl Pts',(7.66602476312854,-0.0891087529615867,
-0.8));
#12394=CARTESIAN_POINT('Ctrl Pts',(7.668541680002,-0.0780641940177735,-0.8));
#12395=CARTESIAN_POINT('Ctrl Pts',(7.67032675800354,-0.0668373958916314,
-0.8));
#12396=CARTESIAN_POINT('Ctrl Pts',(7.67139187266829,-0.0554971482997141,
-0.8));
#12397=CARTESIAN_POINT('Ctrl Pts',(7.67180519341954,-0.051096533221107,
-0.8));
#12398=CARTESIAN_POINT('Ctrl Pts',(7.67210999149788,-0.046678864069736,
-0.8));
#12399=CARTESIAN_POINT('Ctrl Pts',(7.67230656954632,-0.0422483195596408,
-0.8));
#12400=CARTESIAN_POINT('Ctrl Pts',(7.67250906957021,-0.0376843035048666,
-0.8));
#12401=CARTESIAN_POINT('Ctrl Pts',(7.67259626929253,-0.0331164188372603,
-0.8));
#12402=CARTESIAN_POINT('Ctrl Pts',(7.67256984318009,-0.0285512140800657,
-0.8));
#12403=CARTESIAN_POINT('Ctrl Pts',(7.67247176333353,-0.0116075723308694,
-0.8));
#12404=CARTESIAN_POINT('Ctrl Pts',(7.67081310549201,0.00531006786860519,
-0.8));
#12405=CARTESIAN_POINT('Ctrl Pts',(7.66764846978472,0.0219706801239459,
-0.8));
#12406=CARTESIAN_POINT('Ctrl Pts',(7.66599434051542,0.030679046244134,-0.8));
#12407=CARTESIAN_POINT('Ctrl Pts',(7.66392786024929,0.0393169593546687,
-0.8));
#12408=CARTESIAN_POINT('Ctrl Pts',(7.66145143684384,0.0478484196974881,
-0.8));
#12409=CARTESIAN_POINT('Ctrl Pts',(7.66000111794769,0.0528448747139515,
-0.8));
#12410=CARTESIAN_POINT('Ctrl Pts',(7.65840953888752,0.0578064276330517,
-0.8));
#12411=CARTESIAN_POINT('Ctrl Pts',(7.65667852826701,0.0627200905953307,
-0.8));
#12412=CARTESIAN_POINT('Ctrl Pts',(7.65135798251779,0.0778230415981986,
-0.8));
#12413=CARTESIAN_POINT('Ctrl Pts',(7.64474876808975,0.0924061338350732,
-0.8));
#12414=CARTESIAN_POINT('Ctrl Pts',(7.63687446130966,0.106254791359862,-0.8));
#12415=CARTESIAN_POINT('Ctrl Pts',(7.63280785898707,0.113406783837146,-0.8));
#12416=CARTESIAN_POINT('Ctrl Pts',(7.62839917020088,0.120367200011687,-0.8));
#12417=CARTESIAN_POINT('Ctrl Pts',(7.62366908758241,0.127074857095534,-0.8));
#12418=CARTESIAN_POINT('Ctrl Pts',(7.61642296267604,0.137350474876241,-0.8));
#12419=CARTESIAN_POINT('Ctrl Pts',(7.60841819500501,0.147045792077381,-0.8));
#12420=CARTESIAN_POINT('Ctrl Pts',(7.59965864826425,0.156042626060984,-0.8));
#12421=CARTESIAN_POINT('Ctrl Pts',(7.59707211067876,0.158699230328034,-0.8));
#12422=CARTESIAN_POINT('Ctrl Pts',(7.59441967000851,0.161294793130762,-0.8));
#12423=CARTESIAN_POINT('Ctrl Pts',(7.59170404101736,0.163828127476924,-0.8));
#12424=CARTESIAN_POINT('Ctrl Pts',(-7.59134659966651,0.163598720337494,
-0.8));
#12425=CARTESIAN_POINT('Ctrl Pts',(-7.60250980500677,0.153108048469134,
-0.8));
#12426=CARTESIAN_POINT('Ctrl Pts',(-7.61257000344682,0.141586767042882,
-0.8));
#12427=CARTESIAN_POINT('Ctrl Pts',(-7.62152226231139,0.129252378976592,
-0.8));
#12428=CARTESIAN_POINT('Ctrl Pts',(-7.62952885288343,0.118220929071331,
-0.8));
#12429=CARTESIAN_POINT('Ctrl Pts',(-7.63664923653971,0.106537756091835,
-0.8));
#12430=CARTESIAN_POINT('Ctrl Pts',(-7.6428604623543,0.0943309552132166,
-0.8));
#12431=CARTESIAN_POINT('Ctrl Pts',(-7.6449408273248,0.0902424545359381,
-0.8));
#12432=CARTESIAN_POINT('Ctrl Pts',(-7.64691968074795,0.0860935636706147,
-0.8));
#12433=CARTESIAN_POINT('Ctrl Pts',(-7.64879353654417,0.0818932876413604,
-0.8));
#12434=CARTESIAN_POINT('Ctrl Pts',(-7.65549373543205,0.0668746907798337,
-0.799999999999999));
#12435=CARTESIAN_POINT('Ctrl Pts',(-7.66081104753667,0.0513019973078679,
-0.8));
#12436=CARTESIAN_POINT('Ctrl Pts',(-7.66472276438405,0.0354012896611767,
-0.8));
#12437=CARTESIAN_POINT('Ctrl Pts',(-7.6674274853223,0.0244068903774662,
-0.8));
#12438=CARTESIAN_POINT('Ctrl Pts',(-7.66945953155259,0.0132546027280042,
-0.8));
#12439=CARTESIAN_POINT('Ctrl Pts',(-7.6707995714248,0.00201084264178555,
-0.8));
#12440=CARTESIAN_POINT('Ctrl Pts',(-7.67155452692688,-0.00432369912609444,
-0.8));
#12441=CARTESIAN_POINT('Ctrl Pts',(-7.67208965158941,-0.0106873679770006,
-0.799999999999999));
#12442=CARTESIAN_POINT('Ctrl Pts',(-7.67239989442358,-0.0170687147357037,
-0.799999999999999));
#12443=CARTESIAN_POINT('Ctrl Pts',(-7.67261015190465,-0.0213934750445532,
-0.799999999999999));
#12444=CARTESIAN_POINT('Ctrl Pts',(-7.67271662194561,-0.0257172870342268,
-0.8));
#12445=CARTESIAN_POINT('Ctrl Pts',(-7.67271881100292,-0.030034689921079,
-0.8));
#12446=CARTESIAN_POINT('Ctrl Pts',(-7.67272680474609,-0.0458004762743684,
-0.8));
#12447=CARTESIAN_POINT('Ctrl Pts',(-7.67134745337264,-0.0614869416178373,
-0.8));
#12448=CARTESIAN_POINT('Ctrl Pts',(-7.66853799763916,-0.0769182800552743,
-0.8));
#12449=CARTESIAN_POINT('Ctrl Pts',(-7.66621951308713,-0.0896528888827926,
-0.8));
#12450=CARTESIAN_POINT('Ctrl Pts',(-7.66292661247628,-0.102214448564117,
-0.8));
#12451=CARTESIAN_POINT('Ctrl Pts',(-7.65873249789692,-0.114535664709849,
-0.8));
#12452=CARTESIAN_POINT('Ctrl Pts',(-7.65678766591361,-0.120249074484433,
-0.8));
#12453=CARTESIAN_POINT('Ctrl Pts',(-7.65464675118448,-0.125914747432373,
-0.8));
#12454=CARTESIAN_POINT('Ctrl Pts',(-7.6523277720856,-0.131499187137676,
-0.8));
#12455=CARTESIAN_POINT('Ctrl Pts',(-7.64581334288988,-0.147186882242587,
-0.8));
#12456=CARTESIAN_POINT('Ctrl Pts',(-7.63788679434737,-0.162272513758134,
-0.8));
#12457=CARTESIAN_POINT('Ctrl Pts',(-7.62872577033978,-0.176613596666072,
-0.8));
#12458=CARTESIAN_POINT('Ctrl Pts',(-7.62337441159445,-0.184990856607026,
-0.8));
#12459=CARTESIAN_POINT('Ctrl Pts',(-7.61760078226976,-0.193114063113643,
-0.8));
#12460=CARTESIAN_POINT('Ctrl Pts',(-7.61143267714321,-0.200953056122988,
-0.8));
#12461=CARTESIAN_POINT('Ctrl Pts',(-7.60741999113199,-0.206052745078555,
-0.8));
#12462=CARTESIAN_POINT('Ctrl Pts',(-7.60324024590185,-0.21103211435324,
-0.8));
#12463=CARTESIAN_POINT('Ctrl Pts',(-7.59890002279473,-0.215882236431572,
-0.8));
#12464=CARTESIAN_POINT('Ctrl Pts',(-7.59567039942596,-0.21949128306788,
-0.8));
#12465=CARTESIAN_POINT('Ctrl Pts',(-7.5923546276331,-0.223025516298712,
-0.8));
#12466=CARTESIAN_POINT('Ctrl Pts',(-7.58896156037046,-0.226475902517482,
-0.8));
#12467=CARTESIAN_POINT('Ctrl Pts',(-7.57975143871387,-0.235841610408655,
-0.8));
#12468=CARTESIAN_POINT('Ctrl Pts',(-7.5699611571278,-0.244603137305301,
-0.8));
#12469=CARTESIAN_POINT('Ctrl Pts',(-7.55965407220312,-0.252693305854133,
-0.8));
#12470=CARTESIAN_POINT('Ctrl Pts',(-7.55492467495832,-0.256405472885301,
-0.8));
#12471=CARTESIAN_POINT('Ctrl Pts',(-7.55008628895285,-0.25997619102085,
-0.8));
#12472=CARTESIAN_POINT('Ctrl Pts',(-7.54514420724383,-0.263398333429773,
-0.8));
#12473=CARTESIAN_POINT('Ctrl Pts',(-7.53998153614902,-0.266973222866464,
-0.8));
#12474=CARTESIAN_POINT('Ctrl Pts',(-7.53471214755407,-0.27038136610209,
-0.8));
#12475=CARTESIAN_POINT('Ctrl Pts',(-7.52934772811915,-0.273612535916845,
-0.8));
#12476=CARTESIAN_POINT('Ctrl Pts',(-7.51740562694793,-0.280805664138331,
-0.8));
#12477=CARTESIAN_POINT('Ctrl Pts',(-7.50498606409347,-0.287127784604654,
-0.8));
#12478=CARTESIAN_POINT('Ctrl Pts',(-7.49215681113707,-0.292493158241675,
-0.8));
#12479=CARTESIAN_POINT('Ctrl Pts',(-7.48800670405648,-0.294228791266972,
-0.8));
#12480=CARTESIAN_POINT('Ctrl Pts',(-7.48381363090601,-0.295864195413031,
-0.8));
#12481=CARTESIAN_POINT('Ctrl Pts',(-7.47958093846729,-0.297400292044454,
-0.8));
#12482=CARTESIAN_POINT('Ctrl Pts',(-7.32062007174671,-0.29692229537457,
-0.8));
#12483=CARTESIAN_POINT('Ctrl Pts',(-7.30380883220412,-0.290772668854571,
-0.8));
#12484=CARTESIAN_POINT('Ctrl Pts',(-7.28766912732842,-0.283071237438702,
-0.8));
#12485=CARTESIAN_POINT('Ctrl Pts',(-7.27233056528333,-0.274000232887525,
-0.8));
#12486=CARTESIAN_POINT('Ctrl Pts',(-7.26235482816667,-0.268100725715958,
-0.8));
#12487=CARTESIAN_POINT('Ctrl Pts',(-7.25271840516627,-0.261620820891142,
-0.8));
#12488=CARTESIAN_POINT('Ctrl Pts',(-7.24346457290171,-0.254602027234289,
-0.8));
#12489=CARTESIAN_POINT('Ctrl Pts',(-7.23605070657022,-0.248978800392428,
-0.8));
#12490=CARTESIAN_POINT('Ctrl Pts',(-7.22888251109443,-0.243009525157091,
-0.8));
#12491=CARTESIAN_POINT('Ctrl Pts',(-7.22198590500135,-0.236713584164732,
-0.8));
#12492=CARTESIAN_POINT('Ctrl Pts',(-7.21845908607672,-0.233493936189985,
-0.8));
#12493=CARTESIAN_POINT('Ctrl Pts',(-7.21500962230698,-0.2301944813217,-0.8));
#12494=CARTESIAN_POINT('Ctrl Pts',(-7.21164322886242,-0.226821505909535,
-0.8));
#12495=CARTESIAN_POINT('Ctrl Pts',(-7.19928401163746,-0.214438123960911,
-0.8));
#12496=CARTESIAN_POINT('Ctrl Pts',(-7.188027189001,-0.201053074390168,-0.8));
#12497=CARTESIAN_POINT('Ctrl Pts',(-7.17802297542257,-0.186814170855175,
-0.8));
#12498=CARTESIAN_POINT('Ctrl Pts',(-7.171734035686,-0.177863181799981,-0.8));
#12499=CARTESIAN_POINT('Ctrl Pts',(-7.16594090318987,-0.168574168976251,
-0.8));
#12500=CARTESIAN_POINT('Ctrl Pts',(-7.16069107733955,-0.15898056446742,
-0.8));
#12501=CARTESIAN_POINT('Ctrl Pts',(-7.15844631652005,-0.154878457438895,
-0.8));
#12502=CARTESIAN_POINT('Ctrl Pts',(-7.15630099783232,-0.15072064542349,
-0.8));
#12503=CARTESIAN_POINT('Ctrl Pts',(-7.15425934838691,-0.146509707216243,
-0.8));
#12504=CARTESIAN_POINT('Ctrl Pts',(-7.15231303243113,-0.142495396022921,
-0.8));
#12505=CARTESIAN_POINT('Ctrl Pts',(-7.15046484658208,-0.138440800814485,
-0.8));
#12506=CARTESIAN_POINT('Ctrl Pts',(-7.14871818777149,-0.134350401707579,
-0.8));
#12507=CARTESIAN_POINT('Ctrl Pts',(-7.1424623444498,-0.119700204553552,
-0.8));
#12508=CARTESIAN_POINT('Ctrl Pts',(-7.13750154217398,-0.104583094632127,
-0.8));
#12509=CARTESIAN_POINT('Ctrl Pts',(-7.13397519964019,-0.0891090401260764,
-0.8));
#12510=CARTESIAN_POINT('Ctrl Pts',(-7.13145828462303,-0.0780644862322087,
-0.8));
#12511=CARTESIAN_POINT('Ctrl Pts',(-7.12967320857157,-0.0668376893119182,
-0.8));
#12512=CARTESIAN_POINT('Ctrl Pts',(-7.12860809580548,-0.0554974398191664,
-0.8));
#12513=CARTESIAN_POINT('Ctrl Pts',(-7.12819477643118,-0.0510968308188738,
-0.8));
#12514=CARTESIAN_POINT('Ctrl Pts',(-7.12788997938578,-0.0466791673306104,
-0.8));
#12515=CARTESIAN_POINT('Ctrl Pts',(-7.12769340201838,-0.0422486280913985,
-0.8));
#12516=CARTESIAN_POINT('Ctrl Pts',(-7.12749090188967,-0.0376845992915606,
-0.8));
#12517=CARTESIAN_POINT('Ctrl Pts',(-7.12740370260243,-0.0331167012771051,
-0.8));
#12518=CARTESIAN_POINT('Ctrl Pts',(-7.12743012967622,-0.0285514828500066,
-0.8));
#12519=CARTESIAN_POINT('Ctrl Pts',(-7.12752821290038,-0.0116078232524714,
-0.8));
#12520=CARTESIAN_POINT('Ctrl Pts',(-7.12918687525478,0.00530984020385254,
-0.8));
#12521=CARTESIAN_POINT('Ctrl Pts',(-7.13235151603647,0.021970478203028,
-0.8));
#12522=CARTESIAN_POINT('Ctrl Pts',(-7.13400562623726,0.0306787434271353,
-0.8));
#12523=CARTESIAN_POINT('Ctrl Pts',(-7.13607207676681,0.0393165581665612,
-0.8));
#12524=CARTESIAN_POINT('Ctrl Pts',(-7.13854845975925,0.0478479236807756,
-0.8));
#12525=CARTESIAN_POINT('Ctrl Pts',(-7.13999878843953,0.0528444384061105,
-0.8));
#12526=CARTESIAN_POINT('Ctrl Pts',(-7.14159038003695,0.0578060503789822,
-0.8));
#12527=CARTESIAN_POINT('Ctrl Pts',(-7.14332140616028,0.0627197720666046,
-0.8));
#12528=CARTESIAN_POINT('Ctrl Pts',(-7.1486419454519,0.0778227499793214,
-0.8));
#12529=CARTESIAN_POINT('Ctrl Pts',(-7.15525115303475,0.092405870012346,
-0.8));
#12530=CARTESIAN_POINT('Ctrl Pts',(-7.16312545194293,0.106254553939122,
-0.8));
#12531=CARTESIAN_POINT('Ctrl Pts',(-7.16719209102926,0.113406631858387,
-0.8));
#12532=CARTESIAN_POINT('Ctrl Pts',(-7.17160082320644,0.120367129319865,
-0.799999999999999));
#12533=CARTESIAN_POINT('Ctrl Pts',(-7.17633095536696,0.127074861616176,
-0.799999999999999));
#12534=CARTESIAN_POINT('Ctrl Pts',(-7.18357707811536,0.137350483931364,
-0.799999999999999));
#12535=CARTESIAN_POINT('Ctrl Pts',(-7.19158184168782,0.147045804025915,
-0.799999999999999));
#12536=CARTESIAN_POINT('Ctrl Pts',(-7.2003413821471,0.156042638227876,-0.799999999999999));
#12537=CARTESIAN_POINT('Ctrl Pts',(-7.20292792020884,0.158699244953618,
-0.799999999999999));
#12538=CARTESIAN_POINT('Ctrl Pts',(-7.20558036128329,0.161294809871419,
-0.799999999999999));
#12539=CARTESIAN_POINT('Ctrl Pts',(-7.2082959906101,0.163828146011838,-0.799999999999999));
#12540=CARTESIAN_POINT('Origin',(-7.4,0.,0.220842344717745));
#12541=CARTESIAN_POINT('Ctrl Pts',(-7.70772056490863,0.000154295167761212,
-0.0291576552822542));
#12542=CARTESIAN_POINT('Ctrl Pts',(-7.70778424817136,0.0100435505178975,
-0.0296715621794889));
#12543=CARTESIAN_POINT('Ctrl Pts',(-7.70290029244162,0.120578394498565,
-0.035418806655132));
#12544=CARTESIAN_POINT('Ctrl Pts',(-7.56952504259133,0.319794750950713,
-0.0463993887091835));
#12545=CARTESIAN_POINT('Ctrl Pts',(-7.2268011951414,0.317782806798611,-0.0620994014444089));
#12546=CARTESIAN_POINT('Ctrl Pts',(-7.03939107410859,0.0308556281233394,
-0.0777994141796342));
#12547=CARTESIAN_POINT('Ctrl Pts',(-7.17534010740672,-0.283761737281935,
-0.0934994269148595));
#12548=CARTESIAN_POINT('Ctrl Pts',(-7.51274497664259,-0.343916495026914,
-0.109199439650085));
#12549=CARTESIAN_POINT('Ctrl Pts',(-7.69164526295008,-0.155985565502471,
-0.12108551577255));
#12550=CARTESIAN_POINT('Ctrl Pts',(-7.70747663110457,-0.0276893459128193,
-0.127738254316606));
#12551=CARTESIAN_POINT('Ctrl Pts',(-7.70724559592217,-0.000260666439420156,
-0.129157655282254));
#12552=CARTESIAN_POINT('Ctrl Pts',(-7.70701976654778,-0.000306170806070059,
-0.0208423447177452));
#12553=CARTESIAN_POINT('Ctrl Pts',(-7.70655486683947,0.0677880488673211,
-0.0243615716353137));
#12554=CARTESIAN_POINT('Ctrl Pts',(-7.65102809142816,0.238050536013955,
-0.0331141361312906));
#12555=CARTESIAN_POINT('Ctrl Pts',(-7.37136424514298,0.36072194419717,-0.0471000382056761));
#12556=CARTESIAN_POINT('Ctrl Pts',(-7.0833377209053,0.175239119455976,-0.0628000509409012));
#12557=CARTESIAN_POINT('Ctrl Pts',(-7.07914899542098,-0.167517421922754,
-0.0785000636761269));
#12558=CARTESIAN_POINT('Ctrl Pts',(-7.3627280810489,-0.359992553262469,
-0.0942000764113519));
#12559=CARTESIAN_POINT('Ctrl Pts',(-7.64768205623712,-0.242854235705339,
-0.108314170091892));
#12560=CARTESIAN_POINT('Ctrl Pts',(-7.70661024184805,-0.0702887181447709,
-0.117194926194023));
#12561=CARTESIAN_POINT('Ctrl Pts',(-7.70715908192673,0.000245638898741782,
-0.120842344717745));
#12562=CARTESIAN_POINT('Ctrl Pts',(-7.20865340033349,0.163598720337495,
0.));
#12563=CARTESIAN_POINT('Ctrl Pts',(-7.15485882039215,0.100680074451818,
-0.00523333757840845));
#12564=CARTESIAN_POINT('Ctrl Pts',(-7.11504792740546,-0.081320987239729,
-0.0157000127352253));
#12565=CARTESIAN_POINT('Ctrl Pts',(-7.31088738477093,-0.282913381389853,
-0.0314000254704507));
#12566=CARTESIAN_POINT('Ctrl Pts',(-7.58669428177702,-0.230208447695885,
-0.047100038205676));
#12567=CARTESIAN_POINT('Ctrl Pts',(-7.69505959198511,0.0286321132263963,
-0.0628000509409014));
#12568=CARTESIAN_POINT('Ctrl Pts',(-7.53885775003211,0.261943479914891,
-0.0785000636761267));
#12569=CARTESIAN_POINT('Ctrl Pts',(-7.25813307589668,0.260295498980154,
-0.0942000764113521));
#12570=CARTESIAN_POINT('Ctrl Pts',(-7.10462568051681,0.0252738063447232,
-0.109900089146577));
#12571=CARTESIAN_POINT('Ctrl Pts',(-7.21598136339561,-0.232428883555319,
-0.125600101881803));
#12572=CARTESIAN_POINT('Ctrl Pts',(-7.49234926913868,-0.281701570271761,
-0.141300114617028));
#12573=CARTESIAN_POINT('Ctrl Pts',(-7.68590623015859,-0.0783741170228757,
-0.157000127352253));
#12574=CARTESIAN_POINT('Ctrl Pts',(-7.62308856437211,0.195234321246773,
-0.172700140087479));
#12575=CARTESIAN_POINT('Ctrl Pts',(-7.36022512733543,0.293773198343426,
-0.188400152822704));
#12576=CARTESIAN_POINT('Ctrl Pts',(-7.13302825740755,0.12888336190753,-0.204100165557929));
#12577=CARTESIAN_POINT('Ctrl Pts',(-7.1452274819044,-0.15157768529494,-0.219800178293155));
#12578=CARTESIAN_POINT('Ctrl Pts',(-7.38588368162235,-0.296117437159506,
-0.23550019102838));
#12579=CARTESIAN_POINT('Ctrl Pts',(-7.63919811247918,-0.175125907145724,
-0.251200203763605));
#12580=CARTESIAN_POINT('Ctrl Pts',(-7.67802130457259,0.102902736043491,
-0.266900216498831));
#12581=CARTESIAN_POINT('Ctrl Pts',(-7.46754012392463,0.288657492672429,
-0.282600229234056));
#12582=CARTESIAN_POINT('Ctrl Pts',(-7.19649506705352,0.215570314274908,
-0.298300241969282));
#12583=CARTESIAN_POINT('Ctrl Pts',(-7.10793483547166,-0.050820836942206,
-0.314000254704507));
#12584=CARTESIAN_POINT('Ctrl Pts',(-7.28127223907772,-0.271640454175529,
-0.329700267439732));
#12585=CARTESIAN_POINT('Ctrl Pts',(-7.56107396482191,-0.24887747111374,
-0.345400280174958));
#12586=CARTESIAN_POINT('Ctrl Pts',(-7.6964391210875,-0.00294367160307863,
-0.361100292910183));
#12587=CARTESIAN_POINT('Ctrl Pts',(-7.56598447354143,0.245629746235912,
-0.376800305645408));
#12588=CARTESIAN_POINT('Ctrl Pts',(-7.28668995619815,0.273944614280356,
-0.392500318380634));
#12589=CARTESIAN_POINT('Ctrl Pts',(-7.10900164217772,0.0566107185302396,
-0.408200331115859));
#12590=CARTESIAN_POINT('Ctrl Pts',(-7.19225434732208,-0.211486551584725,
-0.423900343851084));
#12591=CARTESIAN_POINT('Ctrl Pts',(-7.46179457226168,-0.289941802019968,
-0.43960035658631));
#12592=CARTESIAN_POINT('Ctrl Pts',(-7.67592301138651,-0.108403456956597,
-0.455300369321535));
#12593=CARTESIAN_POINT('Ctrl Pts',(-7.64262863919221,0.170341307842165,
-0.47100038205676));
#12594=CARTESIAN_POINT('Ctrl Pts',(-7.39176683840533,0.296339387901059,
-0.486700394791986));
#12595=CARTESIAN_POINT('Ctrl Pts',(-7.14828779291894,0.156607095511924,
-0.502400407527211));
#12596=CARTESIAN_POINT('Ctrl Pts',(-7.13052149770804,-0.12355628110687,
-0.518100420262436));
#12597=CARTESIAN_POINT('Ctrl Pts',(-7.35439916203589,-0.292925556596044,
-0.533800432997662));
#12598=CARTESIAN_POINT('Ctrl Pts',(-7.61916753267196,-0.199625672292344,
-0.549500445732886));
#12599=CARTESIAN_POINT('Ctrl Pts',(-7.68740627934318,0.0726804614431528,
-0.565200458468113));
#12600=CARTESIAN_POINT('Ctrl Pts',(-7.49792504763019,0.279813340307149,
-0.580900471203337));
#12601=CARTESIAN_POINT('Ctrl Pts',(-7.22063350732225,0.236034887969839,
-0.596600483938563));
#12602=CARTESIAN_POINT('Ctrl Pts',(-7.10418157928289,-0.0193982633392013,
-0.612300496673788));
#12603=CARTESIAN_POINT('Ctrl Pts',(-7.25299295271724,-0.257436905607251,
-0.628000509409014));
#12604=CARTESIAN_POINT('Ctrl Pts',(-7.53362678302623,-0.26462920363873,
-0.643700522144238));
#12605=CARTESIAN_POINT('Ctrl Pts',(-7.69443654339104,-0.0345263618448277,
-0.659400534879465));
#12606=CARTESIAN_POINT('Ctrl Pts',(-7.59122152812465,0.226537418199014,
-0.675100547614689));
#12607=CARTESIAN_POINT('Ctrl Pts',(-7.31653775068187,0.284461271780152,
-0.690800560349915));
#12608=CARTESIAN_POINT('Ctrl Pts',(-7.11669251625801,0.0873093018200402,
-0.70650057308514));
#12609=CARTESIAN_POINT('Ctrl Pts',(-7.17089758104745,-0.188140467543259,
-0.722200585820366));
#12610=CARTESIAN_POINT('Ctrl Pts',(-7.43052936616057,-0.294869341820571,
-0.73790059855559));
#12611=CARTESIAN_POINT('Ctrl Pts',(-7.66280860159844,-0.137213338782277,
-0.753600611290817));
#12612=CARTESIAN_POINT('Ctrl Pts',(-7.65937760170093,0.143538219530879,
-0.76930062402604));
#12613=CARTESIAN_POINT('Ctrl Pts',(-7.42345550125086,0.295466620280292,
-0.785000636761269));
#12614=CARTESIAN_POINT('Ctrl Pts',(-7.16630823828261,0.182672384524398,
-0.80070064949649));
#12615=CARTESIAN_POINT('Ctrl Pts',(-7.11910685953888,-0.0943918973400733,
-0.816400662231719));
#12616=CARTESIAN_POINT('Ctrl Pts',(-7.25500804955002,-0.221828784507026,
-0.826867337388535));
#12617=CARTESIAN_POINT('Ctrl Pts',(-7.33498000020249,-0.243208680203507,
-0.832100674966943));
#12618=CARTESIAN_POINT('Ctrl Pts',(-7.19456684496579,0.175642532122685,
0.0107002249889811));
#12619=CARTESIAN_POINT('Ctrl Pts',(-7.13681201524657,0.108091940906,0.00546688741057261));
#12620=CARTESIAN_POINT('Ctrl Pts',(-7.09407032365007,-0.0873076762705518,
-0.00499978774624428));
#12621=CARTESIAN_POINT('Ctrl Pts',(-7.30432709161405,-0.303740900761287,
-0.0206998004814696));
#12622=CARTESIAN_POINT('Ctrl Pts',(-7.60043834277246,-0.247155934874821,
-0.0363998132166949));
#12623=CARTESIAN_POINT('Ctrl Pts',(-7.71678129117659,0.0307399523464065,
-0.0520998259519203));
#12624=CARTESIAN_POINT('Ctrl Pts',(-7.54908018088519,0.281227236926832,
-0.0677998386871455));
#12625=CARTESIAN_POINT('Ctrl Pts',(-7.24768911564492,0.27945793491964,-0.0834998514223711));
#12626=CARTESIAN_POINT('Ctrl Pts',(-7.08288081171408,0.027134413604262,
-0.0991998641575962));
#12627=CARTESIAN_POINT('Ctrl Pts',(-7.20243427806597,-0.249539834797524,
-0.114899876892822));
#12628=CARTESIAN_POINT('Ctrl Pts',(-7.49914783830665,-0.302439878523479,
-0.130599889628047));
#12629=CARTESIAN_POINT('Ctrl Pts',(-7.70695407709247,-0.084143863340614,
-0.146299902363272));
#12630=CARTESIAN_POINT('Ctrl Pts',(-7.63951189992867,0.209607082930084,
-0.161999915098497));
#12631=CARTESIAN_POINT('Ctrl Pts',(-7.35729698046994,0.315400195798434,
-0.177699927833723));
#12632=CARTESIAN_POINT('Ctrl Pts',(-7.1133743297172,0.138371498183013,-0.193399940568948));
#12633=CARTESIAN_POINT('Ctrl Pts',(-7.1264716368119,-0.162736532434825,
-0.209099953304173));
#12634=CARTESIAN_POINT('Ctrl Pts',(-7.38484446639323,-0.317917012804747,
-0.224799966039399));
#12635=CARTESIAN_POINT('Ctrl Pts',(-7.6568074008656,-0.188018327453308,
-0.240499978774624));
#12636=CARTESIAN_POINT('Ctrl Pts',(-7.69848867899726,0.110478230414916,
-0.25619999150985));
#12637=CARTESIAN_POINT('Ctrl Pts',(-7.47251229325957,0.309907882070095,
-0.271900004245075));
#12638=CARTESIAN_POINT('Ctrl Pts',(-7.18151343941786,0.231440171241058,
-0.287600016980301));
#12639=CARTESIAN_POINT('Ctrl Pts',(-7.0864335800625,-0.0545621656863128,
-0.303300029715526));
#12640=CARTESIAN_POINT('Ctrl Pts',(-7.27253173790952,-0.291638083109205,
-0.319000042450751));
#12641=CARTESIAN_POINT('Ctrl Pts',(-7.57293190913717,-0.267199334594605,
-0.334700055185977));
#12642=CARTESIAN_POINT('Ctrl Pts',(-7.7182623784625,-0.00316037884059091,
-0.350400067921202));
#12643=CARTESIAN_POINT('Ctrl Pts',(-7.57820391972335,0.263712518683071,
-0.366100080656427));
#12644=CARTESIAN_POINT('Ctrl Pts',(-7.27834829656839,0.294111870889409,
-0.381800093391653));
#12645=CARTESIAN_POINT('Ctrl Pts',(-7.0875789229524,0.0607782868192583,
-0.397500106126878));
#12646=CARTESIAN_POINT('Ctrl Pts',(-7.17696052635036,-0.227055770079409,
-0.413200118862103));
#12647=CARTESIAN_POINT('Ctrl Pts',(-7.46634376553245,-0.311286739712534,
-0.428900131597328));
#12648=CARTESIAN_POINT('Ctrl Pts',(-7.69623591364813,-0.116383903440261,
-0.444600144332554));
#12649=CARTESIAN_POINT('Ctrl Pts',(-7.66049047611917,0.182881495483375,
-0.460300157067779));
#12650=CARTESIAN_POINT('Ctrl Pts',(-7.39116072945509,0.318155303117609,
-0.476000169803005));
#12651=CARTESIAN_POINT('Ctrl Pts',(-7.12975724182498,0.16813619780979,-0.49170018253823));
#12652=CARTESIAN_POINT('Ctrl Pts',(-7.11068302736388,-0.132652248309177,
-0.507400195273455));
#12653=CARTESIAN_POINT('Ctrl Pts',(-7.35104211921456,-0.31449015235472,
-0.523100208008681));
#12654=CARTESIAN_POINT('Ctrl Pts',(-7.63530220968826,-0.214321716488908,
-0.538800220743905));
#12655=CARTESIAN_POINT('Ctrl Pts',(-7.70856455690886,0.0780310521829601,
-0.554500233479132));
#12656=CARTESIAN_POINT('Ctrl Pts',(-7.50513409449975,0.300412640831581,
-0.570200246214356));
#12657=CARTESIAN_POINT('Ctrl Pts',(-7.20742890355809,0.253411306071293,
-0.585900258949583));
#12658=CARTESIAN_POINT('Ctrl Pts',(-7.08240401663227,-0.0208263248309716,
-0.601600271684806));
#12659=CARTESIAN_POINT('Ctrl Pts',(-7.24217058683982,-0.276388897598994,
-0.617300284420033));
#12660=CARTESIAN_POINT('Ctrl Pts',(-7.54346412051216,-0.28411067827933,
-0.633000297155257));
#12661=CARTESIAN_POINT('Ctrl Pts',(-7.71611237498659,-0.0370681238025536,
-0.648700309890484));
#12662=CARTESIAN_POINT('Ctrl Pts',(-7.60529887597468,0.243214651501716,
-0.664400322625709));
#12663=CARTESIAN_POINT('Ctrl Pts',(-7.31039342620376,0.305402743757612,
-0.680100335360934));
#12664=CARTESIAN_POINT('Ctrl Pts',(-7.09583598385675,0.0937368386372456,
-0.695800348096159));
#12665=CARTESIAN_POINT('Ctrl Pts',(-7.1540315175006,-0.201990993852965,
-0.711500360831385));
#12666=CARTESIAN_POINT('Ctrl Pts',(-7.43277687726091,-0.316577035174062,
-0.72720037356661));
#12667=CARTESIAN_POINT('Ctrl Pts',(-7.68215604714478,-0.147314711355987,
-0.742900386301836));
#12668=CARTESIAN_POINT('Ctrl Pts',(-7.67847246387183,0.1541052172216,-0.75860039903706));
#12669=CARTESIAN_POINT('Ctrl Pts',(-7.42518224851276,0.31721828408378,-0.774300411772287));
#12670=CARTESIAN_POINT('Ctrl Pts',(-7.14910431646667,0.1961203614586,-0.790000424507511));
#12671=CARTESIAN_POINT('Ctrl Pts',(-7.09842806627886,-0.10134084072585,
-0.805700437242737));
#12672=CARTESIAN_POINT('Ctrl Pts',(-7.24433403108591,-0.2381593775803,-0.816167112399554));
#12673=CARTESIAN_POINT('Ctrl Pts',(-7.3301933573839,-0.261113218593862,
-0.821400449977962));
#12674=CARTESIAN_POINT('Ctrl Pts',(-7.18048028959809,0.187686343907875,
0.0214004499779621));
#12675=CARTESIAN_POINT('Ctrl Pts',(-7.11876521010099,0.115503807360182,
0.0161671123995537));
#12676=CARTESIAN_POINT('Ctrl Pts',(-7.07309271989468,-0.0932943653013744,
0.00570043724273679));
#12677=CARTESIAN_POINT('Ctrl Pts',(-7.29776679845717,-0.324568420132722,
-0.00999957549248856));
#12678=CARTESIAN_POINT('Ctrl Pts',(-7.61418240376789,-0.264103422053756,
-0.0256995882277139));
#12679=CARTESIAN_POINT('Ctrl Pts',(-7.73850299036808,0.0328477914664162,
-0.0413996009629393));
#12680=CARTESIAN_POINT('Ctrl Pts',(-7.55930261173826,0.300510993938772,
-0.0570996136981645));
#12681=CARTESIAN_POINT('Ctrl Pts',(-7.23724515539316,0.298620370859126,
-0.0727996264333899));
#12682=CARTESIAN_POINT('Ctrl Pts',(-7.06113594291133,0.0289950208638007,
-0.0884996391686152));
#12683=CARTESIAN_POINT('Ctrl Pts',(-7.18888719273634,-0.26665078603973,
-0.104199651903841));
#12684=CARTESIAN_POINT('Ctrl Pts',(-7.50594640747463,-0.323178186775197,
-0.119899664639066));
#12685=CARTESIAN_POINT('Ctrl Pts',(-7.72800192402634,-0.0899136096583525,
-0.135599677374291));
#12686=CARTESIAN_POINT('Ctrl Pts',(-7.65593523548524,0.223979844613395,
-0.151299690109517));
#12687=CARTESIAN_POINT('Ctrl Pts',(-7.35436883360446,0.337027193253441,
-0.166999702844742));
#12688=CARTESIAN_POINT('Ctrl Pts',(-7.09372040202686,0.147859634458496,
-0.182699715579967));
#12689=CARTESIAN_POINT('Ctrl Pts',(-7.10771579171938,-0.173895379574711,
-0.198399728315193));
#12690=CARTESIAN_POINT('Ctrl Pts',(-7.3838052511641,-0.339716588449989,
-0.214099741050418));
#12691=CARTESIAN_POINT('Ctrl Pts',(-7.67441668925201,-0.200910747760891,
-0.229799753785643));
#12692=CARTESIAN_POINT('Ctrl Pts',(-7.71895605342194,0.11805372478634,-0.245499766520869));
#12693=CARTESIAN_POINT('Ctrl Pts',(-7.47748446259449,0.331158271467761,
-0.261199779256094));
#12694=CARTESIAN_POINT('Ctrl Pts',(-7.16653181178222,0.247310028207208,
-0.276899791991319));
#12695=CARTESIAN_POINT('Ctrl Pts',(-7.06493232465333,-0.0583034944304196,
-0.292599804726545));
#12696=CARTESIAN_POINT('Ctrl Pts',(-7.26379123674133,-0.311635712042882,
-0.30829981746177));
#12697=CARTESIAN_POINT('Ctrl Pts',(-7.58478985345242,-0.285521198075471,
-0.323999830196996));
#12698=CARTESIAN_POINT('Ctrl Pts',(-7.7400856358375,-0.00337708607810321,
-0.339699842932221));
#12699=CARTESIAN_POINT('Ctrl Pts',(-7.59042336590528,0.28179529113023,-0.355399855667446));
#12700=CARTESIAN_POINT('Ctrl Pts',(-7.27000663693862,0.314279127498463,
-0.371099868402672));
#12701=CARTESIAN_POINT('Ctrl Pts',(-7.06615620372709,0.0649458551082769,
-0.386799881137897));
#12702=CARTESIAN_POINT('Ctrl Pts',(-7.16166670537864,-0.242624988574094,
-0.402499893873122));
#12703=CARTESIAN_POINT('Ctrl Pts',(-7.47089295880322,-0.332631677405099,
-0.418199906608348));
#12704=CARTESIAN_POINT('Ctrl Pts',(-7.71654881590975,-0.124364349923924,
-0.433899919343572));
#12705=CARTESIAN_POINT('Ctrl Pts',(-7.67835231304613,0.195421683124586,
-0.449599932078799));
#12706=CARTESIAN_POINT('Ctrl Pts',(-7.39055462050486,0.339971218334158,
-0.465299944814023));
#12707=CARTESIAN_POINT('Ctrl Pts',(-7.11122669073103,0.179665300107655,
-0.48099995754925));
#12708=CARTESIAN_POINT('Ctrl Pts',(-7.09084455701971,-0.141748215511483,
-0.496699970284474));
#12709=CARTESIAN_POINT('Ctrl Pts',(-7.34768507639324,-0.336054748113396,
-0.512399983019701));
#12710=CARTESIAN_POINT('Ctrl Pts',(-7.65143688670457,-0.229017760685471,
-0.528099995754924));
#12711=CARTESIAN_POINT('Ctrl Pts',(-7.72972283447454,0.083381642922767,
-0.543800008490151));
#12712=CARTESIAN_POINT('Ctrl Pts',(-7.51234314136931,0.321011941356013,
-0.559500021225375));
#12713=CARTESIAN_POINT('Ctrl Pts',(-7.19422429979393,0.270787724172747,
-0.575200033960601));
#12714=CARTESIAN_POINT('Ctrl Pts',(-7.06062645398167,-0.0222543863227421,
-0.590900046695826));
#12715=CARTESIAN_POINT('Ctrl Pts',(-7.23134822096239,-0.295340889590735,
-0.606600059431052));
#12716=CARTESIAN_POINT('Ctrl Pts',(-7.55330145799812,-0.303592152919931,
-0.622300072166277));
#12717=CARTESIAN_POINT('Ctrl Pts',(-7.73778820658214,-0.0396098857602792,
-0.638000084901502));
#12718=CARTESIAN_POINT('Ctrl Pts',(-7.6193762238247,0.259891884804417,-0.653700097636727));
#12719=CARTESIAN_POINT('Ctrl Pts',(-7.30424910172566,0.326344215735072,
-0.669400110371953));
#12720=CARTESIAN_POINT('Ctrl Pts',(-7.07497945145549,0.100164375454451,
-0.685100123107178));
#12721=CARTESIAN_POINT('Ctrl Pts',(-7.13716545395374,-0.215841520162671,
-0.700800135842404));
#12722=CARTESIAN_POINT('Ctrl Pts',(-7.43502438836124,-0.338284728527552,
-0.716500148577629));
#12723=CARTESIAN_POINT('Ctrl Pts',(-7.70150349269112,-0.157416083929697,
-0.732200161312854));
#12724=CARTESIAN_POINT('Ctrl Pts',(-7.69756732604273,0.164672214912321,
-0.74790017404808));
#12725=CARTESIAN_POINT('Ctrl Pts',(-7.42690899577466,0.338969947887268,
-0.763600186783304));
#12726=CARTESIAN_POINT('Ctrl Pts',(-7.13190039465073,0.209568338392803,
-0.779300199518531));
#12727=CARTESIAN_POINT('Ctrl Pts',(-7.07774927301882,-0.108289784111627,
-0.795000212253755));
#12728=CARTESIAN_POINT('Ctrl Pts',(-7.2336600126218,-0.254489970653575,
-0.805466887410573));
#12729=CARTESIAN_POINT('Ctrl Pts',(-7.32540671456531,-0.279017756984216,
-0.810700224988981));
#12730=CARTESIAN_POINT('Ctrl Pts',(-7.16639373423038,0.199730155693065,
0.0321006749669432));
#12731=CARTESIAN_POINT('Ctrl Pts',(-7.10071840495542,0.122915673814364,
0.0268673373885347));
#12732=CARTESIAN_POINT('Ctrl Pts',(-7.05211511613929,-0.0992810543321975,
0.0164006622317178));
#12733=CARTESIAN_POINT('Ctrl Pts',(-7.29120650530028,-0.345395939504156,
0.000700649496492501));
#12734=CARTESIAN_POINT('Ctrl Pts',(-7.62792646476333,-0.281050909232692,
-0.0149993632387328));
#12735=CARTESIAN_POINT('Ctrl Pts',(-7.76022468955957,0.0349556305864266,
-0.0306993759739582));
#12736=CARTESIAN_POINT('Ctrl Pts',(-7.56952504259133,0.319794750950713,
-0.0463993887091835));
#12737=CARTESIAN_POINT('Ctrl Pts',(-7.2268011951414,0.317782806798611,-0.0620994014444089));
#12738=CARTESIAN_POINT('Ctrl Pts',(-7.03939107410859,0.0308556281233394,
-0.0777994141796342));
#12739=CARTESIAN_POINT('Ctrl Pts',(-7.17534010740672,-0.283761737281935,
-0.0934994269148595));
#12740=CARTESIAN_POINT('Ctrl Pts',(-7.51274497664259,-0.343916495026914,
-0.109199439650085));
#12741=CARTESIAN_POINT('Ctrl Pts',(-7.74904977096025,-0.0956833559760907,
-0.12489945238531));
#12742=CARTESIAN_POINT('Ctrl Pts',(-7.67235857104177,0.238352606296705,
-0.140599465120536));
#12743=CARTESIAN_POINT('Ctrl Pts',(-7.351440686739,0.358654190708449,-0.156299477855761));
#12744=CARTESIAN_POINT('Ctrl Pts',(-7.07406647433649,0.15734777073398,-0.171999490590986));
#12745=CARTESIAN_POINT('Ctrl Pts',(-7.08895994662689,-0.185054226714597,
-0.187699503326211));
#12746=CARTESIAN_POINT('Ctrl Pts',(-7.38276603593497,-0.36151616409523,
-0.203399516061437));
#12747=CARTESIAN_POINT('Ctrl Pts',(-7.69202597763844,-0.213803168068474,
-0.219099528796662));
#12748=CARTESIAN_POINT('Ctrl Pts',(-7.73942342784661,0.125629219157764,
-0.234799541531888));
#12749=CARTESIAN_POINT('Ctrl Pts',(-7.48245663192943,0.352408660865427,
-0.250499554267113));
#12750=CARTESIAN_POINT('Ctrl Pts',(-7.15155018414657,0.263179885173358,
-0.266199567002338));
#12751=CARTESIAN_POINT('Ctrl Pts',(-7.04343106924415,-0.0620448231745263,
-0.281899579737564));
#12752=CARTESIAN_POINT('Ctrl Pts',(-7.25505073557315,-0.331633340976559,
-0.297599592472789));
#12753=CARTESIAN_POINT('Ctrl Pts',(-7.59664779776768,-0.303843061556337,
-0.313299605208015));
#12754=CARTESIAN_POINT('Ctrl Pts',(-7.76190889321249,-0.00359379331561558,
-0.328999617943239));
#12755=CARTESIAN_POINT('Ctrl Pts',(-7.60264281208722,0.299878063577389,
-0.344699630678465));
#12756=CARTESIAN_POINT('Ctrl Pts',(-7.26166497730884,0.334446384107517,
-0.36039964341369));
#12757=CARTESIAN_POINT('Ctrl Pts',(-7.04473348450178,0.0691134233972956,
-0.376099656148916));
#12758=CARTESIAN_POINT('Ctrl Pts',(-7.14637288440692,-0.258194207068779,
-0.391799668884141));
#12759=CARTESIAN_POINT('Ctrl Pts',(-7.47544215207399,-0.353976615097665,
-0.407499681619366));
#12760=CARTESIAN_POINT('Ctrl Pts',(-7.73686171817138,-0.132344796407588,
-0.423199694354592));
#12761=CARTESIAN_POINT('Ctrl Pts',(-7.69621414997308,0.207961870765797,
-0.438899707089817));
#12762=CARTESIAN_POINT('Ctrl Pts',(-7.38994851155463,0.361787133550707,
-0.454599719825042));
#12763=CARTESIAN_POINT('Ctrl Pts',(-7.09269613963708,0.191194402405521,
-0.470299732560268));
#12764=CARTESIAN_POINT('Ctrl Pts',(-7.07100608667554,-0.15084418271379,
-0.485999745295493));
#12765=CARTESIAN_POINT('Ctrl Pts',(-7.34432803357192,-0.357619343872072,
-0.501699758030719));
#12766=CARTESIAN_POINT('Ctrl Pts',(-7.66757156372086,-0.243713804882034,
-0.517399770765943));
#12767=CARTESIAN_POINT('Ctrl Pts',(-7.75088111204022,0.0887322336625739,
-0.53309978350117));
#12768=CARTESIAN_POINT('Ctrl Pts',(-7.51955218823887,0.341611241880446,
-0.548799796236394));
#12769=CARTESIAN_POINT('Ctrl Pts',(-7.18101969602976,0.288164142274201,
-0.56449980897162));
#12770=CARTESIAN_POINT('Ctrl Pts',(-7.03884889133106,-0.0236824478145123,
-0.580199821706845));
#12771=CARTESIAN_POINT('Ctrl Pts',(-7.22052585508497,-0.314292881582478,
-0.595899834442071));
#12772=CARTESIAN_POINT('Ctrl Pts',(-7.56313879548406,-0.323073627560531,
-0.611599847177296));
#12773=CARTESIAN_POINT('Ctrl Pts',(-7.75946403817769,-0.0421516477180053,
-0.627299859912521));
#12774=CARTESIAN_POINT('Ctrl Pts',(-7.63345357167473,0.276569118107119,
-0.642999872647746));
#12775=CARTESIAN_POINT('Ctrl Pts',(-7.29810477724755,0.347285687712531,
-0.658699885382972));
#12776=CARTESIAN_POINT('Ctrl Pts',(-7.05412291905423,0.106591912271656,
-0.674399898118197));
#12777=CARTESIAN_POINT('Ctrl Pts',(-7.12029939040689,-0.229692046472377,
-0.690099910853423));
#12778=CARTESIAN_POINT('Ctrl Pts',(-7.43727189946158,-0.359992421881043,
-0.705799923588648));
#12779=CARTESIAN_POINT('Ctrl Pts',(-7.72085093823746,-0.167517456503407,
-0.721499936323873));
#12780=CARTESIAN_POINT('Ctrl Pts',(-7.71666218821363,0.175239212603042,
-0.737199949059098));
#12781=CARTESIAN_POINT('Ctrl Pts',(-7.42863574303655,0.360721611690756,
-0.752899961794324));
#12782=CARTESIAN_POINT('Ctrl Pts',(-7.1146964728348,0.223016315327006,-0.768599974529548));
#12783=CARTESIAN_POINT('Ctrl Pts',(-7.05707047975879,-0.115238727497404,
-0.784299987264776));
#12784=CARTESIAN_POINT('Ctrl Pts',(-7.22298599415769,-0.270820563726849,
-0.794766662421592));
#12785=CARTESIAN_POINT('Ctrl Pts',(-7.32062007174671,-0.29692229537457,
-0.8));
#12786=CARTESIAN_POINT('Ctrl Pts',(-7.20865340033349,0.163598720337495,
0.));
#12787=CARTESIAN_POINT('Ctrl Pts',(-7.19749016426694,0.153108019593971,
-2.76372499376297E-18));
#12788=CARTESIAN_POINT('Ctrl Pts',(-7.18742993143982,0.141586713971671,
-8.45132788489384E-17));
#12789=CARTESIAN_POINT('Ctrl Pts',(-7.1784776381451,0.129252304447995,-5.46437894932694E-17));
#12790=CARTESIAN_POINT('Ctrl Pts',(-7.17047115113201,0.118221020461395,
-2.79299999936894E-17));
#12791=CARTESIAN_POINT('Ctrl Pts',(-7.16335084130231,0.106538037408676,
2.44997822749073E-17));
#12792=CARTESIAN_POINT('Ctrl Pts',(-7.15713966083231,0.0943314427665496,
2.60208521396521E-17));
#12793=CARTESIAN_POINT('Ctrl Pts',(-7.15505924455693,0.0902428804903266,
2.65303299302091E-17));
#12794=CARTESIAN_POINT('Ctrl Pts',(-7.15308034324392,0.0860939263230946,
-2.27985261165535E-17));
#12795=CARTESIAN_POINT('Ctrl Pts',(-7.15120644281776,0.0818935847012138,
-2.16840434497101E-17));
#12796=CARTESIAN_POINT('Ctrl Pts',(-7.14450619729809,0.0668750064778017,
-1.76991425494042E-17));
#12797=CARTESIAN_POINT('Ctrl Pts',(-7.13918883905698,0.0513023322829503,
3.17673853203519E-17));
#12798=CARTESIAN_POINT('Ctrl Pts',(-7.13527708034929,0.0354016414449469,
2.94902990916057E-17));
#12799=CARTESIAN_POINT('Ctrl Pts',(-7.13257231819721,0.0244072039082036,
2.79158214438866E-17));
#12800=CARTESIAN_POINT('Ctrl Pts',(-7.13054023888487,0.0132548753996132,
-1.66159572056239E-18));
#12801=CARTESIAN_POINT('Ctrl Pts',(-7.12920017560294,0.00201107170221857,
-5.20417042793042E-18));
#12802=CARTESIAN_POINT('Ctrl Pts',(-7.12844522682347,-0.00432332757017003,
-7.1999436780392E-18));
#12803=CARTESIAN_POINT('Ctrl Pts',(-7.1279101003675,-0.0106868532653293,
2.05898758024937E-17));
#12804=CARTESIAN_POINT('Ctrl Pts',(-7.12759984712261,-0.0170680571507328,
1.90819582357449E-17));
#12805=CARTESIAN_POINT('Ctrl Pts',(-7.12738957317498,-0.021392914194958,
1.80599680239007E-17));
#12806=CARTESIAN_POINT('Ctrl Pts',(-7.12728309197496,-0.0257168244094562,
-4.90358507150565E-18));
#12807=CARTESIAN_POINT('Ctrl Pts',(-7.12728089724359,-0.0300343251795264,
-5.20417042793042E-18));
#12808=CARTESIAN_POINT('Ctrl Pts',(-7.12727288296517,-0.0458001057272751,
-6.30178754895358E-18));
#12809=CARTESIAN_POINT('Ctrl Pts',(-7.12865222250825,-0.0614865713174629,
6.0937287207194E-17));
#12810=CARTESIAN_POINT('Ctrl Pts',(-7.13146167838013,-0.0769179188083685,
6.93889390390723E-17));
#12811=CARTESIAN_POINT('Ctrl Pts',(-7.13378015998439,-0.0896525182889436,
7.27129920200424E-17));
#12812=CARTESIAN_POINT('Ctrl Pts',(-7.13707306322478,-0.102214075074238,
5.18772623636705E-17));
#12813=CARTESIAN_POINT('Ctrl Pts',(-7.1412671846214,-0.114535293399235,
3.12250225675825E-17));
#12814=CARTESIAN_POINT('Ctrl Pts',(-7.14321202162556,-0.120248709647508,
2.16484661506902E-17));
#12815=CARTESIAN_POINT('Ctrl Pts',(-7.14535294266045,-0.125914390083585,
4.01380311714632E-17));
#12816=CARTESIAN_POINT('Ctrl Pts',(-7.14767192915255,-0.131498838079198,
3.81639164714898E-17));
#12817=CARTESIAN_POINT('Ctrl Pts',(-7.15418636647591,-0.14718652603121,
3.26182841334338E-17));
#12818=CARTESIAN_POINT('Ctrl Pts',(-7.16211292622978,-0.162272159028203,
2.16855313984206E-17));
#12819=CARTESIAN_POINT('Ctrl Pts',(-7.17127396198873,-0.176613249443012,
-1.04083408558608E-17));
#12820=CARTESIAN_POINT('Ctrl Pts',(-7.17662531782903,-0.18499049847543,
-2.91557549305296E-17));
#12821=CARTESIAN_POINT('Ctrl Pts',(-7.18239894289445,-0.193113697063826,
2.13680762433296E-17));
#12822=CARTESIAN_POINT('Ctrl Pts',(-7.18856704204723,-0.200952684844035,
2.08166817117217E-17));
#12823=CARTESIAN_POINT('Ctrl Pts',(-7.19257962089004,-0.206052239137303,
2.04579789774165E-17));
#12824=CARTESIAN_POINT('Ctrl Pts',(-7.1967592496289,-0.211031481079785,
3.56529973313533E-17));
#12825=CARTESIAN_POINT('Ctrl Pts',(-7.20109934731034,-0.215881483781976,
3.81639164714898E-17));
#12826=CARTESIAN_POINT('Ctrl Pts',(-7.20432878913168,-0.219490343008123,
4.00322770191852E-17));
#12827=CARTESIAN_POINT('Ctrl Pts',(-7.20764437108191,-0.223024398793103,
4.33361061948454E-19));
#12828=CARTESIAN_POINT('Ctrl Pts',(-7.21103723976682,-0.226474616868443,
3.46944695195361E-18));
#12829=CARTESIAN_POINT('Ctrl Pts',(-7.22024722842187,-0.235840281231676,
1.17109438089107E-17));
#12830=CARTESIAN_POINT('Ctrl Pts',(-7.23003736548959,-0.24460178169824,
3.42136972519736E-17));
#12831=CARTESIAN_POINT('Ctrl Pts',(-7.24034429477035,-0.252691942380673,
3.12250225675825E-17));
#12832=CARTESIAN_POINT('Ctrl Pts',(-7.24508022119563,-0.256409286772693,
2.98517577445839E-17));
#12833=CARTESIAN_POINT('Ctrl Pts',(-7.24992543835673,-0.259984791203115,
2.74594575473033E-17));
#12834=CARTESIAN_POINT('Ctrl Pts',(-7.25487463133442,-0.263411298803592,
1.73472347597681E-17));
#12835=CARTESIAN_POINT('Ctrl Pts',(-7.26003204798081,-0.266981967277684,
6.80956803886786E-18));
#12836=CARTESIAN_POINT('Ctrl Pts',(-7.26529590651007,-0.270386211806602,
-2.31583854274773E-17));
#12837=CARTESIAN_POINT('Ctrl Pts',(-7.27065460638826,-0.273613872126434,
-2.08166817117217E-17));
#12838=CARTESIAN_POINT('Ctrl Pts',(-7.28259601671275,-0.280806440686599,
-1.55983926558145E-17));
#12839=CARTESIAN_POINT('Ctrl Pts',(-7.29501481903722,-0.287128105902613,
9.97222803653275E-18));
#12840=CARTESIAN_POINT('Ctrl Pts',(-7.30784325376688,-0.292493143353308,
-6.93889390390723E-18));
#12841=CARTESIAN_POINT('Ctrl Pts',(-7.31199336468935,-0.29422877992884,
-1.2253478561421E-17));
#12842=CARTESIAN_POINT('Ctrl Pts',(-7.31618644117717,-0.295864187143585,
2.68855459144816E-18));
#12843=CARTESIAN_POINT('Ctrl Pts',(-7.32041913648099,-0.297400286396329,
0.));
#12844=CARTESIAN_POINT('Ctrl Pts',(-7.65166448275063,-0.000213511554003356,
-0.161258330249198));
#12845=CARTESIAN_POINT('Ctrl Pts',(-7.65185372337913,-0.0226803085523069,
-0.15983892928355));
#12846=CARTESIAN_POINT('Ctrl Pts',(-7.64908704070277,-0.0451012973586514,
-0.158419528317902));
#12847=CARTESIAN_POINT('Ctrl Pts',(-7.64317712569085,-0.0666606195194149,
-0.157000127352254));
#12848=CARTESIAN_POINT('Ctrl Pts',(-7.62138724315195,-0.146149934772504,
-0.151766789773845));
#12849=CARTESIAN_POINT('Ctrl Pts',(-7.55686825614531,-0.213925752522132,
-0.146533452195437));
#12850=CARTESIAN_POINT('Ctrl Pts',(-7.47854744501815,-0.239601546944206,
-0.141300114617028));
#12851=CARTESIAN_POINT('Ctrl Pts',(-7.40022663389099,-0.265277341366279,
-0.13606677703862));
#12852=CARTESIAN_POINT('Ctrl Pts',(-7.3081039986433,-0.248853112460798,
-0.130833439460212));
#12853=CARTESIAN_POINT('Ctrl Pts',(-7.24348340053965,-0.197690549691385,
-0.125600101881803));
#12854=CARTESIAN_POINT('Ctrl Pts',(-7.17886280243601,-0.146527986921971,
-0.120366764303395));
#12855=CARTESIAN_POINT('Ctrl Pts',(-7.14174424147641,-0.0606270902886238,
-0.115133426724986));
#12856=CARTESIAN_POINT('Ctrl Pts',(-7.14876952689325,0.0214936401339547,
-0.109900089146578));
#12857=CARTESIAN_POINT('Ctrl Pts',(-7.1557948123101,0.103614370556533,-0.104666751568169));
#12858=CARTESIAN_POINT('Ctrl Pts',(-7.20696394410339,0.181954934768343,
-0.099433413989761));
#12859=CARTESIAN_POINT('Ctrl Pts',(-7.27933595568927,0.221399880363371,
-0.0942000764113526));
#12860=CARTESIAN_POINT('Ctrl Pts',(-7.35170796727516,0.260844825958399,
-0.0889667388329441));
#12861=CARTESIAN_POINT('Ctrl Pts',(-7.44528285865364,0.261394152936645,
-0.0837334012545357));
#12862=CARTESIAN_POINT('Ctrl Pts',(-7.51810394466837,0.222783588644352,
-0.0785000636761272));
#12863=CARTESIAN_POINT('Ctrl Pts',(-7.59092503068311,0.184173024352059,
-0.0732667260977187));
#12864=CARTESIAN_POINT('Ctrl Pts',(-7.64299231133411,0.106402568789228,
-0.0680333885193103));
#12865=CARTESIAN_POINT('Ctrl Pts',(-7.65096506662493,0.0243772475207652,
-0.0628000509409019));
#12866=CARTESIAN_POINT('Ctrl Pts',(-7.6517479807543,0.0163224683829433,
-0.0622861440436673));
#12867=CARTESIAN_POINT('Ctrl Pts',(-7.6521056921332,0.00822665964822356,
-0.0617722371464327));
#12868=CARTESIAN_POINT('Ctrl Pts',(-7.65205352925247,0.000126382978640343,
-0.0612583302491982));
#12869=CARTESIAN_POINT('Ctrl Pts',(-7.47937992825329,-0.29692229537457,
0.));
#12870=CARTESIAN_POINT('Ctrl Pts',(-7.57701400584231,-0.270820563726849,
-0.00523333757840845));
#12871=CARTESIAN_POINT('Ctrl Pts',(-7.74292936377346,-0.115237711690175,
-0.0157000127352254));
#12872=CARTESIAN_POINT('Ctrl Pts',(-7.68530366248674,0.2230159413608,-0.0314000254704506));
#12873=CARTESIAN_POINT('Ctrl Pts',(-7.37136424514298,0.36072194419717,-0.0471000382056761));
#12874=CARTESIAN_POINT('Ctrl Pts',(-7.0833377209053,0.175239119455976,-0.0628000509409012));
#12875=CARTESIAN_POINT('Ctrl Pts',(-7.07914899542098,-0.167517421922754,
-0.0785000636761269));
#12876=CARTESIAN_POINT('Ctrl Pts',(-7.3627280810489,-0.359992553262469,
-0.0942000764113519));
#12877=CARTESIAN_POINT('Ctrl Pts',(-7.67970068592657,-0.229692080624575,
-0.109900089146577));
#12878=CARTESIAN_POINT('Ctrl Pts',(-7.74587716255528,0.106591926360324,
-0.125600101881803));
#12879=CARTESIAN_POINT('Ctrl Pts',(-7.50189525062872,0.347285780617978,
-0.141300114617028));
#12880=CARTESIAN_POINT('Ctrl Pts',(-7.16654636885183,0.276569183243976,
-0.157000127352254));
#12881=CARTESIAN_POINT('Ctrl Pts',(-7.04053587339322,-0.0421516562996225,
-0.172700140087479));
#12882=CARTESIAN_POINT('Ctrl Pts',(-7.23686116352416,-0.323073708797981,
-0.188400152822704));
#12883=CARTESIAN_POINT('Ctrl Pts',(-7.5794741897514,-0.314292959115147,
-0.204100165557929));
#12884=CARTESIAN_POINT('Ctrl Pts',(-7.76115119822227,-0.0236824539723921,
-0.219800178293155));
#12885=CARTESIAN_POINT('Ctrl Pts',(-7.61898035843412,0.288164213987784,
-0.23550019102838));
#12886=CARTESIAN_POINT('Ctrl Pts',(-7.28044778202723,0.341611326648396,
-0.251200203763605));
#12887=CARTESIAN_POINT('Ctrl Pts',(-7.04911880083639,0.0887322557395692,
-0.266900216498831));
#12888=CARTESIAN_POINT('Ctrl Pts',(-7.13242836981262,-0.243713865431744,
-0.282600229234056));
#12889=CARTESIAN_POINT('Ctrl Pts',(-7.45567198026117,-0.357619432680664,
-0.298300241969282));
#12890=CARTESIAN_POINT('Ctrl Pts',(-7.72899399503084,-0.150844220183267,
-0.314000254704507));
#12891=CARTESIAN_POINT('Ctrl Pts',(-7.70730393668735,0.191194449893827,
-0.329700267439732));
#12892=CARTESIAN_POINT('Ctrl Pts',(-7.41005149094087,0.36178722340353,-0.345400280174957));
#12893=CARTESIAN_POINT('Ctrl Pts',(-7.10378577645897,0.207961922416443,
-0.361100292910183));
#12894=CARTESIAN_POINT('Ctrl Pts',(-7.06313819816462,-0.132344829277446,
-0.376800305645408));
#12895=CARTESIAN_POINT('Ctrl Pts',(-7.32455782918916,-0.35397670301188,
-0.392500318380633));
#12896=CARTESIAN_POINT('Ctrl Pts',(-7.65362717858442,-0.25819427119465,
-0.408200331115859));
#12897=CARTESIAN_POINT('Ctrl Pts',(-7.75526660373307,0.069113440562637,
-0.423900343851084));
#12898=CARTESIAN_POINT('Ctrl Pts',(-7.53833505704833,0.334446467171126,
-0.43960035658631));
#12899=CARTESIAN_POINT('Ctrl Pts',(-7.19735713758398,0.299878138056265,
-0.455300369321535));
#12900=CARTESIAN_POINT('Ctrl Pts',(-7.03809101690294,-0.0035937942090703,
-0.47100038205676));
#12901=CARTESIAN_POINT('Ctrl Pts',(-7.20335215339251,-0.30384313701778,
-0.486700394791986));
#12902=CARTESIAN_POINT('Ctrl Pts',(-7.54494930042661,-0.331633423345088,
-0.50240040752721));
#12903=CARTESIAN_POINT('Ctrl Pts',(-7.75656901931451,-0.0620448385777456,
-0.518100420262437));
#12904=CARTESIAN_POINT('Ctrl Pts',(-7.64844987755816,0.263179950525062,
-0.533800432997661));
#12905=CARTESIAN_POINT('Ctrl Pts',(-7.31754334759326,0.352408748413955,
-0.549500445732887));
#12906=CARTESIAN_POINT('Ctrl Pts',(-7.06057648784951,0.125629250314373,
-0.565200458468112));
#12907=CARTESIAN_POINT('Ctrl Pts',(-7.10797394984171,-0.213803221083396,
-0.580900471203338));
#12908=CARTESIAN_POINT('Ctrl Pts',(-7.41723396832727,-0.361516254045136,
-0.596600483938562));
#12909=CARTESIAN_POINT('Ctrl Pts',(-7.71104013066228,-0.185054272366607,
-0.612300496673789));
#12910=CARTESIAN_POINT('Ctrl Pts',(-7.72593360653096,0.157347809231622,
-0.628000509409013));
#12911=CARTESIAN_POINT('Ctrl Pts',(-7.44855932549587,0.358654280875835,
-0.643700522144239));
#12912=CARTESIAN_POINT('Ctrl Pts',(-7.12764136094462,0.238352663458736,
-0.659400534879464));
#12913=CARTESIAN_POINT('Ctrl Pts',(-7.05095014313138,-0.0956833759672795,
-0.675100547614689));
#12914=CARTESIAN_POINT('Ctrl Pts',(-7.28725499370478,-0.34391658738075,
-0.690800560349915));
#12915=CARTESIAN_POINT('Ctrl Pts',(-7.62465995186745,-0.283761795119453,
-0.70650057308514));
#12916=CARTESIAN_POINT('Ctrl Pts',(-7.76060900814316,0.0308556130297948,
-0.722200585820366));
#12917=CARTESIAN_POINT('Ctrl Pts',(-7.57319886321716,0.317782926109968,
-0.737900598555591));
#12918=CARTESIAN_POINT('Ctrl Pts',(-7.23047488314852,0.319794760031351,
-0.753600611290816));
#12919=CARTESIAN_POINT('Ctrl Pts',(-7.03977528830754,0.0349557588279105,
-0.769300624026042));
#12920=CARTESIAN_POINT('Ctrl Pts',(-7.17207333714996,-0.281051176556267,
-0.785000636761267));
#12921=CARTESIAN_POINT('Ctrl Pts',(-7.50879381804844,-0.345395707969619,
-0.800700649496492));
#12922=CARTESIAN_POINT('Ctrl Pts',(-7.74788417951995,-0.0992818028310835,
-0.816400662231718));
#12923=CARTESIAN_POINT('Ctrl Pts',(-7.69928159504458,0.122915673814362,
-0.826867337388535));
#12924=CARTESIAN_POINT('Ctrl Pts',(-7.63360626576962,0.199730155693063,
-0.832100674966943));
#12925=CARTESIAN_POINT('Ctrl Pts',(-7.47459328543469,-0.279017756984216,
0.0107002249889811));
#12926=CARTESIAN_POINT('Ctrl Pts',(-7.5663399873782,-0.254489970653575,
0.00546688741057261));
#12927=CARTESIAN_POINT('Ctrl Pts',(-7.7222505799485,-0.108288829557998,
-0.0049997877462443));
#12928=CARTESIAN_POINT('Ctrl Pts',(-7.66809973251085,0.209567986976916,
-0.0206998004814696));
#12929=CARTESIAN_POINT('Ctrl Pts',(-7.37309099311766,0.338970260343406,
-0.036399813216695));
#12930=CARTESIAN_POINT('Ctrl Pts',(-7.10243258855636,0.164672127382063,
-0.0520998259519203));
#12931=CARTESIAN_POINT('Ctrl Pts',(-7.09849644496774,-0.157416051434272,
-0.0677998386871457));
#12932=CARTESIAN_POINT('Ctrl Pts',(-7.36497559332446,-0.338284851986623,
-0.083499851422371));
#12933=CARTESIAN_POINT('Ctrl Pts',(-7.66283461777677,-0.215841552255477,
-0.0991998641575963));
#12934=CARTESIAN_POINT('Ctrl Pts',(-7.72502062523293,0.100164388693566,
-0.114899876892822));
#12935=CARTESIAN_POINT('Ctrl Pts',(-7.49575092446967,0.326344303038281,
-0.130599889628047));
#12936=CARTESIAN_POINT('Ctrl Pts',(-7.18062372028813,0.259891946013495,
-0.146299902363272));
#12937=CARTESIAN_POINT('Ctrl Pts',(-7.06221171032109,-0.0396098938244216,
-0.161999915098498));
#12938=CARTESIAN_POINT('Ctrl Pts',(-7.24669850348192,-0.303592229258729,
-0.177699927833723));
#12939=CARTESIAN_POINT('Ctrl Pts',(-7.56865182117034,-0.295340962448153,
-0.193399940568948));
#12940=CARTESIAN_POINT('Ctrl Pts',(-7.73937363017156,-0.022254392109299,
-0.209099953304174));
#12941=CARTESIAN_POINT('Ctrl Pts',(-7.60577575138577,0.270787791561971,
-0.224799966039399));
#12942=CARTESIAN_POINT('Ctrl Pts',(-7.28765683068976,0.321012021012421,
-0.240499978774624));
#12943=CARTESIAN_POINT('Ctrl Pts',(-7.07027708365565,0.0833816636685102,
-0.25619999150985));
#12944=CARTESIAN_POINT('Ctrl Pts',(-7.14856305083687,-0.229017817584008,
-0.271900004245075));
#12945=CARTESIAN_POINT('Ctrl Pts',(-7.4523149366057,-0.336054831566793,
-0.287600016980301));
#12946=CARTESIAN_POINT('Ctrl Pts',(-7.70915551975974,-0.141748250721535,
-0.303300029715525));
#12947=CARTESIAN_POINT('Ctrl Pts',(-7.688773380991,0.179665344732397,-0.319000042450751));
#12948=CARTESIAN_POINT('Ctrl Pts',(-7.40944538184016,0.339971302768818,
-0.334700055185976));
#12949=CARTESIAN_POINT('Ctrl Pts',(-7.12164761782211,0.195421731660677,
-0.350400067921202));
#12950=CARTESIAN_POINT('Ctrl Pts',(-7.08345110547122,-0.124364380811717,
-0.366100080656427));
#12951=CARTESIAN_POINT('Ctrl Pts',(-7.32910702358977,-0.33263176001805,
-0.381800093391652));
#12952=CARTESIAN_POINT('Ctrl Pts',(-7.6383333538143,-0.242625048833148,
-0.397500106126878));
#12953=CARTESIAN_POINT('Ctrl Pts',(-7.73384387918716,0.064945871238541,
-0.413200118862103));
#12954=CARTESIAN_POINT('Ctrl Pts',(-7.52999339534681,0.314279205553302,
-0.428900131597329));
#12955=CARTESIAN_POINT('Ctrl Pts',(-7.20957658680075,0.281795361117998,
-0.444600144332554));
#12956=CARTESIAN_POINT('Ctrl Pts',(-7.05991427969802,-0.00337708691768223,
-0.460300157067779));
#12957=CARTESIAN_POINT('Ctrl Pts',(-7.21521010065283,-0.285521268986558,
-0.476000169803004));
#12958=CARTESIAN_POINT('Ctrl Pts',(-7.53620879708761,-0.311635789444555,
-0.49170018253823));
#12959=CARTESIAN_POINT('Ctrl Pts',(-7.73506775856522,-0.0583035089048183,
-0.507400195273455));
#12960=CARTESIAN_POINT('Ctrl Pts',(-7.63346824620169,0.247310089618177,
-0.523100208008681));
#12961=CARTESIAN_POINT('Ctrl Pts',(-7.32251551816297,0.331158353737076,
-0.538800220743905));
#12962=CARTESIAN_POINT('Ctrl Pts',(-7.08104386735775,0.118053754064193,
-0.554500233479132));
#12963=CARTESIAN_POINT('Ctrl Pts',(-7.12558324260111,-0.200910797578991,
-0.570200246214356));
#12964=CARTESIAN_POINT('Ctrl Pts',(-7.41619475284112,-0.339716672975878,
-0.585900258949582));
#12965=CARTESIAN_POINT('Ctrl Pts',(-7.6922842809092,-0.173895422473886,
-0.601600271684807));
#12966=CARTESIAN_POINT('Ctrl Pts',(-7.70627967396427,0.147859670634715,
-0.617300284420033));
#12967=CARTESIAN_POINT('Ctrl Pts',(-7.44563117789263,0.337027277983696,
-0.633000297155258));
#12968=CARTESIAN_POINT('Ctrl Pts',(-7.14406470060242,0.223979898328531,
-0.648700309890483));
#12969=CARTESIAN_POINT('Ctrl Pts',(-7.07199799524557,-0.0899136284440642,
-0.664400322625708));
#12970=CARTESIAN_POINT('Ctrl Pts',(-7.29405356466082,-0.323178273560057,
-0.680100335360934));
#12971=CARTESIAN_POINT('Ctrl Pts',(-7.61111286296356,-0.266650840389621,
-0.695800348096159));
#12972=CARTESIAN_POINT('Ctrl Pts',(-7.73886413438061,0.0289950066804033,
-0.711500360831385));
#12973=CARTESIAN_POINT('Ctrl Pts',(-7.56275489944635,0.298620482975957,
-0.72720037356661));
#12974=CARTESIAN_POINT('Ctrl Pts',(-7.24069731847952,0.300511002471844,
-0.742900386301835));
#12975=CARTESIAN_POINT('Ctrl Pts',(-7.06149698883364,0.0328479119748854,
-0.75860039903706));
#12976=CARTESIAN_POINT('Ctrl Pts',(-7.18581741009011,-0.264103673257608,
-0.774300411772286));
#12977=CARTESIAN_POINT('Ctrl Pts',(-7.5022335053935,-0.324568202559814,
-0.790000424507511));
#12978=CARTESIAN_POINT('Ctrl Pts',(-7.7269066182366,-0.0932950686654655,
-0.805700437242737));
#12979=CARTESIAN_POINT('Ctrl Pts',(-7.68123478989901,0.11550380736018,-0.816167112399554));
#12980=CARTESIAN_POINT('Ctrl Pts',(-7.61951971040191,0.187686343907874,
-0.821400449977962));
#12981=CARTESIAN_POINT('Ctrl Pts',(-7.4698066426161,-0.261113218593861,
0.0214004499779621));
#12982=CARTESIAN_POINT('Ctrl Pts',(-7.55566596891409,-0.2381593775803,0.0161671123995537));
#12983=CARTESIAN_POINT('Ctrl Pts',(-7.70157179612354,-0.101339947425821,
0.00570043724273678));
#12984=CARTESIAN_POINT('Ctrl Pts',(-7.65089580253497,0.196120032593032,
-0.00999957549248853));
#12985=CARTESIAN_POINT('Ctrl Pts',(-7.37481774109234,0.317218576489643,
-0.0256995882277139));
#12986=CARTESIAN_POINT('Ctrl Pts',(-7.12152745620743,0.154105135308149,
-0.0413996009629392));
#12987=CARTESIAN_POINT('Ctrl Pts',(-7.1178438945145,-0.14731468094579,-0.0570996136981647));
#12988=CARTESIAN_POINT('Ctrl Pts',(-7.36722310560002,-0.316577150710778,
-0.0727996264333899));
#12989=CARTESIAN_POINT('Ctrl Pts',(-7.64596854962699,-0.20199102388638,
-0.0884996391686153));
#12990=CARTESIAN_POINT('Ctrl Pts',(-7.70416408791058,0.0937368510268085,
-0.104199651903841));
#12991=CARTESIAN_POINT('Ctrl Pts',(-7.48960659831061,0.305402825458584,
-0.119899664639066));
#12992=CARTESIAN_POINT('Ctrl Pts',(-7.19470107172442,0.243214708783014,
-0.135599677374291));
#12993=CARTESIAN_POINT('Ctrl Pts',(-7.08388754724896,-0.0370681313492207,
-0.151299690109517));
#12994=CARTESIAN_POINT('Ctrl Pts',(-7.25653584343968,-0.284110749719476,
-0.166999702844742));
#12995=CARTESIAN_POINT('Ctrl Pts',(-7.55782945258926,-0.276388965781158,
-0.182699715579967));
#12996=CARTESIAN_POINT('Ctrl Pts',(-7.71759606212085,-0.0208263302462058,
-0.198399728315193));
#12997=CARTESIAN_POINT('Ctrl Pts',(-7.59257114433741,0.253411369136158,
-0.214099741050418));
#12998=CARTESIAN_POINT('Ctrl Pts',(-7.29486587935229,0.300412715376446,
-0.229799753785643));
#12999=CARTESIAN_POINT('Ctrl Pts',(-7.09143536647491,0.078031071597451,
-0.245499766520869));
#13000=CARTESIAN_POINT('Ctrl Pts',(-7.16469773186114,-0.214321769736272,
-0.261199779256094));
#13001=CARTESIAN_POINT('Ctrl Pts',(-7.44895789295024,-0.314490230452922,
-0.276899791991319));
#13002=CARTESIAN_POINT('Ctrl Pts',(-7.68931704448864,-0.132652281259804,
-0.292599804726545));
#13003=CARTESIAN_POINT('Ctrl Pts',(-7.67024282529466,0.168136239570967,
-0.30829981746177));
#13004=CARTESIAN_POINT('Ctrl Pts',(-7.40883927273945,0.318155382134106,
-0.323999830196995));
#13005=CARTESIAN_POINT('Ctrl Pts',(-7.13950945918524,0.182881540904911,
-0.339699842932221));
#13006=CARTESIAN_POINT('Ctrl Pts',(-7.10376401277782,-0.116383932345987,
-0.355399855667446));
#13007=CARTESIAN_POINT('Ctrl Pts',(-7.33365621799037,-0.311286817024221,
-0.371099868402672));
#13008=CARTESIAN_POINT('Ctrl Pts',(-7.62303952904418,-0.227055826471647,
-0.386799881137896));
#13009=CARTESIAN_POINT('Ctrl Pts',(-7.71242115464125,0.0607783019144452,
-0.402499893873122));
#13010=CARTESIAN_POINT('Ctrl Pts',(-7.52165173364529,0.294111943935478,
-0.418199906608347));
#13011=CARTESIAN_POINT('Ctrl Pts',(-7.22179603601754,0.263712584179732,
-0.433899919343573));
#13012=CARTESIAN_POINT('Ctrl Pts',(-7.08173754249308,-0.00316037962629422,
-0.449599932078798));
#13013=CARTESIAN_POINT('Ctrl Pts',(-7.22706804791315,-0.267199400955335,
-0.465299944814023));
#13014=CARTESIAN_POINT('Ctrl Pts',(-7.52746829374862,-0.291638155544021,
-0.480999957549249));
#13015=CARTESIAN_POINT('Ctrl Pts',(-7.71356649781592,-0.0545621792318911,
-0.496699970284474));
#13016=CARTESIAN_POINT('Ctrl Pts',(-7.61848661484522,0.231440228711292,
-0.512399983019699));
#13017=CARTESIAN_POINT('Ctrl Pts',(-7.3274876887327,0.309907959060197,-0.528099995754925));
#13018=CARTESIAN_POINT('Ctrl Pts',(-7.10151124686598,0.110478257814012,
-0.54380000849015));
#13019=CARTESIAN_POINT('Ctrl Pts',(-7.1431925353605,-0.188018374074586,
-0.559500021225376));
#13020=CARTESIAN_POINT('Ctrl Pts',(-7.41515553735499,-0.31791709190662,
-0.575200033960601));
#13021=CARTESIAN_POINT('Ctrl Pts',(-7.67352843115613,-0.162736572581166,
-0.590900046695826));
#13022=CARTESIAN_POINT('Ctrl Pts',(-7.68662574139757,0.138371532037808,
-0.606600059431052));
#13023=CARTESIAN_POINT('Ctrl Pts',(-7.44270303028938,0.315400275091557,
-0.622300072166277));
#13024=CARTESIAN_POINT('Ctrl Pts',(-7.16048804026023,0.209607133198326,
-0.638000084901502));
#13025=CARTESIAN_POINT('Ctrl Pts',(-7.09304584735977,-0.0841438809208489,
-0.653700097636728));
#13026=CARTESIAN_POINT('Ctrl Pts',(-7.30085213561686,-0.302439959739364,
-0.669400110371953));
#13027=CARTESIAN_POINT('Ctrl Pts',(-7.59756577405967,-0.249539885659789,
-0.685100123107178));
#13028=CARTESIAN_POINT('Ctrl Pts',(-7.71711926061806,0.0271344003310113,
-0.700800135842403));
#13029=CARTESIAN_POINT('Ctrl Pts',(-7.55231093567554,0.279458039841947,
-0.716500148577629));
#13030=CARTESIAN_POINT('Ctrl Pts',(-7.25091975381051,0.281227244912337,
-0.732200161312854));
#13031=CARTESIAN_POINT('Ctrl Pts',(-7.08321868935976,0.0307400651218602,
-0.74790017404808));
#13032=CARTESIAN_POINT('Ctrl Pts',(-7.19956148303025,-0.247156169958949,
-0.763600186783305));
#13033=CARTESIAN_POINT('Ctrl Pts',(-7.49567319273855,-0.303740697150009,
-0.77930019951853));
#13034=CARTESIAN_POINT('Ctrl Pts',(-7.70592905695325,-0.0873083344998472,
-0.795000212253755));
#13035=CARTESIAN_POINT('Ctrl Pts',(-7.66318798475343,0.108091940905998,
-0.805466887410572));
#13036=CARTESIAN_POINT('Ctrl Pts',(-7.60543315503421,0.175642532122684,
-0.810700224988981));
#13037=CARTESIAN_POINT('Ctrl Pts',(-7.46501999979751,-0.243208680203507,
0.0321006749669432));
#13038=CARTESIAN_POINT('Ctrl Pts',(-7.54499195044998,-0.221828784507026,
0.0268673373885347));
#13039=CARTESIAN_POINT('Ctrl Pts',(-7.68089301229858,-0.094391065293644,
0.0164006622317178));
#13040=CARTESIAN_POINT('Ctrl Pts',(-7.6336918725591,0.182672078209147,0.000700649496492535));
#13041=CARTESIAN_POINT('Ctrl Pts',(-7.37654448906701,0.295466892635879,
-0.0149993632387329));
#13042=CARTESIAN_POINT('Ctrl Pts',(-7.1406223238585,0.143538143234235,-0.0306993759739581));
#13043=CARTESIAN_POINT('Ctrl Pts',(-7.13719134406127,-0.137213310457307,
-0.0463993887091836));
#13044=CARTESIAN_POINT('Ctrl Pts',(-7.36947061787559,-0.294869449434932,
-0.0620994014444088));
#13045=CARTESIAN_POINT('Ctrl Pts',(-7.62910248147719,-0.188140495517282,
-0.0777994141796343));
#13046=CARTESIAN_POINT('Ctrl Pts',(-7.68330755058823,0.0873093133600507,
-0.0934994269148595));
#13047=CARTESIAN_POINT('Ctrl Pts',(-7.48346227215155,0.284461347878887,
-0.109199439650085));
#13048=CARTESIAN_POINT('Ctrl Pts',(-7.20877842316073,0.226537471552532,
-0.12489945238531));
#13049=CARTESIAN_POINT('Ctrl Pts',(-7.10556338417682,-0.0345263688740197,
-0.140599465120536));
#13050=CARTESIAN_POINT('Ctrl Pts',(-7.26637318339745,-0.264629270180224,
-0.156299477855761));
#13051=CARTESIAN_POINT('Ctrl Pts',(-7.54700708400818,-0.257436969114164,
-0.171999490590986));
#13052=CARTESIAN_POINT('Ctrl Pts',(-7.69581849407014,-0.0193982683831129,
-0.187699503326212));
#13053=CARTESIAN_POINT('Ctrl Pts',(-7.57936653728905,0.236034946710346,
-0.203399516061437));
#13054=CARTESIAN_POINT('Ctrl Pts',(-7.30207492801482,0.279813409740471,
-0.219099528796662));
#13055=CARTESIAN_POINT('Ctrl Pts',(-7.11259364929416,0.0726804795263919,
-0.234799541531888));
#13056=CARTESIAN_POINT('Ctrl Pts',(-7.1808324128854,-0.199625721888536,
-0.250499554267113));
#13057=CARTESIAN_POINT('Ctrl Pts',(-7.44560084929478,-0.292925629339051,
-0.266199567002339));
#13058=CARTESIAN_POINT('Ctrl Pts',(-7.66947856921755,-0.123556311798072,
-0.281899579737563));
#13059=CARTESIAN_POINT('Ctrl Pts',(-7.65171226959831,0.156607134409536,
-0.297599592472789));
#13060=CARTESIAN_POINT('Ctrl Pts',(-7.40823316363873,0.296339461499394,
-0.313299605208014));
#13061=CARTESIAN_POINT('Ctrl Pts',(-7.15737130054838,0.170341350149144,
-0.32899961794324));
#13062=CARTESIAN_POINT('Ctrl Pts',(-7.12407692008441,-0.108403483880257,
-0.344699630678465));
#13063=CARTESIAN_POINT('Ctrl Pts',(-7.33820541239099,-0.289941874030391,
-0.360399643413691));
#13064=CARTESIAN_POINT('Ctrl Pts',(-7.60774570427405,-0.211486604110145,
-0.376099656148916));
#13065=CARTESIAN_POINT('Ctrl Pts',(-7.69099843009533,0.0566107325903492,
-0.391799668884141));
#13066=CARTESIAN_POINT('Ctrl Pts',(-7.51331007194377,0.273944682317654,
-0.407499681619366));
#13067=CARTESIAN_POINT('Ctrl Pts',(-7.23401548523432,0.245629807241466,
-0.423199694354592));
#13068=CARTESIAN_POINT('Ctrl Pts',(-7.10356080528816,-0.00294367233490627,
-0.438899707089817));
#13069=CARTESIAN_POINT('Ctrl Pts',(-7.23892599517347,-0.248877532924113,
-0.454599719825043));
#13070=CARTESIAN_POINT('Ctrl Pts',(-7.51872779040962,-0.271640521643488,
-0.470299732560268));
#13071=CARTESIAN_POINT('Ctrl Pts',(-7.69206523706663,-0.0508208495589636,
-0.485999745295494));
#13072=CARTESIAN_POINT('Ctrl Pts',(-7.60350498348874,0.215570367804407,
-0.501699758030718));
#13073=CARTESIAN_POINT('Ctrl Pts',(-7.33245985930243,0.288657564383319,
-0.517399770765944));
#13074=CARTESIAN_POINT('Ctrl Pts',(-7.12197862637422,0.102902761563831,
-0.533099783501169));
#13075=CARTESIAN_POINT('Ctrl Pts',(-7.1608018281199,-0.175125950570181,
-0.548799796236394));
#13076=CARTESIAN_POINT('Ctrl Pts',(-7.41411632186885,-0.296117510837361,
-0.56449980897162));
#13077=CARTESIAN_POINT('Ctrl Pts',(-7.65477258140305,-0.151577722688444,
-0.580199821706845));
#13078=CARTESIAN_POINT('Ctrl Pts',(-7.66697180883088,0.128883393440901,
-0.59589983444207));
#13079=CARTESIAN_POINT('Ctrl Pts',(-7.43977488268614,0.293773272199418,
-0.611599847177296));
#13080=CARTESIAN_POINT('Ctrl Pts',(-7.17691137991803,0.195234368068121,
-0.627299859912521));
#13081=CARTESIAN_POINT('Ctrl Pts',(-7.11409369947397,-0.0783741333976333,
-0.642999872647747));
#13082=CARTESIAN_POINT('Ctrl Pts',(-7.30765070657289,-0.281701645918672,
-0.658699885382972));
#13083=CARTESIAN_POINT('Ctrl Pts',(-7.58401868515578,-0.232428930929957,
-0.674399898118197));
#13084=CARTESIAN_POINT('Ctrl Pts',(-7.69537438685551,0.0252737939816199,
-0.690099910853423));
#13085=CARTESIAN_POINT('Ctrl Pts',(-7.54186697190474,0.260295596707937,
-0.705799923588648));
#13086=CARTESIAN_POINT('Ctrl Pts',(-7.2611421891415,0.261943487352831,-0.721499936323873));
#13087=CARTESIAN_POINT('Ctrl Pts',(-7.10494038988587,0.028632218268835,
-0.737199949059099));
#13088=CARTESIAN_POINT('Ctrl Pts',(-7.2133055559704,-0.23020866666029,-0.752899961794324));
#13089=CARTESIAN_POINT('Ctrl Pts',(-7.4891128800836,-0.282913191740204,
-0.76859997452955));
#13090=CARTESIAN_POINT('Ctrl Pts',(-7.68495149566991,-0.0813216003342288,
-0.784299987264774));
#13091=CARTESIAN_POINT('Ctrl Pts',(-7.64514117960785,0.100680074451816,
-0.794766662421591));
#13092=CARTESIAN_POINT('Ctrl Pts',(-7.59134659966651,0.163598720337494,
-0.8));
#13093=CARTESIAN_POINT('Ctrl Pts',(-7.65159361924534,0.000201202514259572,
-0.0887416697508019));
#13094=CARTESIAN_POINT('Ctrl Pts',(-7.65178908806815,0.0253219403653002,
-0.0903275888054878));
#13095=CARTESIAN_POINT('Ctrl Pts',(-7.64832166662565,0.0503900135757667,
-0.0919135078601737));
#13096=CARTESIAN_POINT('Ctrl Pts',(-7.64096582599694,0.0742596843003013,
-0.0934994269148595));
#13097=CARTESIAN_POINT('Ctrl Pts',(-7.616692457776,0.153026658199663,-0.098732764493268));
#13098=CARTESIAN_POINT('Ctrl Pts',(-7.55007736496378,0.218744003039275,
-0.103966102071676));
#13099=CARTESIAN_POINT('Ctrl Pts',(-7.4709891770592,0.241948696071355,-0.109199439650085));
#13100=CARTESIAN_POINT('Ctrl Pts',(-7.39190098915461,0.265153389103436,
-0.114432777228493));
#13101=CARTESIAN_POINT('Ctrl Pts',(-7.30033970615767,0.245845430327984,
-0.119666114806902));
#13102=CARTESIAN_POINT('Ctrl Pts',(-7.23735655816188,0.192680810869166,
-0.12489945238531));
#13103=CARTESIAN_POINT('Ctrl Pts',(-7.17437341016609,0.139516191410348,
-0.130132789963719));
#13104=CARTESIAN_POINT('Ctrl Pts',(-7.13996839717146,0.0524949112681644,
-0.135366127542127));
#13105=CARTESIAN_POINT('Ctrl Pts',(-7.14956752387758,-0.0293662123539616,
-0.140599465120536));
#13106=CARTESIAN_POINT('Ctrl Pts',(-7.1591666505837,-0.111227335976088,
-0.145832802698944));
#13107=CARTESIAN_POINT('Ctrl Pts',(-7.21276991699057,-0.187928303078155,
-0.151066140277352));
#13108=CARTESIAN_POINT('Ctrl Pts',(-7.28634386696247,-0.225080069784846,
-0.156299477855761));
#13109=CARTESIAN_POINT('Ctrl Pts',(-7.35991781693436,-0.262231836491537,
-0.161532815434169));
#13110=CARTESIAN_POINT('Ctrl Pts',(-7.45346245047127,-0.25983440280285,
-0.166766153012578));
#13111=CARTESIAN_POINT('Ctrl Pts',(-7.52503666891672,-0.218962569169999,
-0.171999490590986));
#13112=CARTESIAN_POINT('Ctrl Pts',(-7.59661088736217,-0.178090735537147,
-0.177232828169395));
#13113=CARTESIAN_POINT('Ctrl Pts',(-7.64621469071615,-0.0987445019601298,
-0.182466165747803));
#13114=CARTESIAN_POINT('Ctrl Pts',(-7.65160793292963,-0.016499182656045,
-0.187699503326212));
#13115=CARTESIAN_POINT('Ctrl Pts',(-7.65196593620322,-0.0110397405648857,
-0.188046892134408));
#13116=CARTESIAN_POINT('Ctrl Pts',(-7.65212913444403,-0.00556752422984645,
-0.188394280942605));
#13117=CARTESIAN_POINT('Ctrl Pts',(-7.65210261813639,-9.36994259479408E-5,
-0.188741669750802));
#13118=CARTESIAN_POINT('Ctrl Pts',(-7.47937992825329,-0.29692229537457,
0.));
#13119=CARTESIAN_POINT('Ctrl Pts',(-7.49619114386871,-0.290772677607239,
-8.69477011477833E-19));
#13120=CARTESIAN_POINT('Ctrl Pts',(-7.51233082429301,-0.283071243582746,
-2.76754902901489E-17));
#13121=CARTESIAN_POINT('Ctrl Pts',(-7.52766936287682,-0.274000229956832,
-3.51281503885303E-17));
#13122=CARTESIAN_POINT('Ctrl Pts',(-7.53764505481519,-0.268100734577494,
-3.99751207082049E-17));
#13123=CARTESIAN_POINT('Ctrl Pts',(-7.5472814350885,-0.261620842282721,
9.85568025155778E-18));
#13124=CARTESIAN_POINT('Ctrl Pts',(-7.55653522793476,-0.254602062866676,
1.64798730217797E-17));
#13125=CARTESIAN_POINT('Ctrl Pts',(-7.56394892482147,-0.248978952000698,
2.1786859911754E-17));
#13126=CARTESIAN_POINT('Ctrl Pts',(-7.57111696210311,-0.243009806706639,
1.89150345061034E-17));
#13127=CARTESIAN_POINT('Ctrl Pts',(-7.57801342324538,-0.236714009089512,
2.86229373536173E-17));
#13128=CARTESIAN_POINT('Ctrl Pts',(-7.58154042561042,-0.233494199301952,
3.35877730275079E-17));
#13129=CARTESIAN_POINT('Ctrl Pts',(-7.58499006695748,-0.23019457260616,
-3.76648489097615E-18));
#13130=CARTESIAN_POINT('Ctrl Pts',(-7.5883566289172,-0.226821418549513,
8.67361737988404E-19));
#13131=CARTESIAN_POINT('Ctrl Pts',(-7.60071585533099,-0.21443799141716,
1.78790075474068E-17));
#13132=CARTESIAN_POINT('Ctrl Pts',(-7.61197268590976,-0.201052893031173,
4.33275306678286E-18));
#13133=CARTESIAN_POINT('Ctrl Pts',(-7.62197690688824,-0.186813942786284,
1.04083408558608E-17));
#13134=CARTESIAN_POINT('Ctrl Pts',(-7.62826586469373,-0.177862905271498,
1.42276402627068E-17));
#13135=CARTESIAN_POINT('Ctrl Pts',(-7.63405901293069,-0.168573843374886,
-1.87641832666448E-17));
#13136=CARTESIAN_POINT('Ctrl Pts',(-7.63930885204487,-0.158980190860473,
-2.60208521396521E-17));
#13137=CARTESIAN_POINT('Ctrl Pts',(-7.64155361520625,-0.154878069389871,
-2.9123709695134E-17));
#13138=CARTESIAN_POINT('Ctrl Pts',(-7.64369893607691,-0.150720243293487,
-2.44962438590674E-18));
#13139=CARTESIAN_POINT('Ctrl Pts',(-7.64574058754886,-0.146509291490871,
0.));
#13140=CARTESIAN_POINT('Ctrl Pts',(-7.64768690274554,-0.142494972887256,
2.3352375437085E-18));
#13141=CARTESIAN_POINT('Ctrl Pts',(-7.6495350879677,-0.138440370831646,
-9.39867744994685E-18));
#13142=CARTESIAN_POINT('Ctrl Pts',(-7.65128174628091,-0.134349965575425,
-6.93889390390723E-18));
#13143=CARTESIAN_POINT('Ctrl Pts',(-7.65753758940913,-0.11969974267822,
1.87108334065775E-18));
#13144=CARTESIAN_POINT('Ctrl Pts',(-7.66249839256794,-0.104582615525194,
3.46944695195361E-18));
#13145=CARTESIAN_POINT('Ctrl Pts',(-7.66602473772058,-0.0891085568120877,
3.46944695195361E-18));
#13146=CARTESIAN_POINT('Ctrl Pts',(-7.66854165586043,-0.0780639944149697,
-3.18384531345276E-19));
#13147=CARTESIAN_POINT('Ctrl Pts',(-7.67032673519256,-0.0668371954593955,
-2.99514844422014E-17));
#13148=CARTESIAN_POINT('Ctrl Pts',(-7.67139185115297,-0.0554969491587786,
-3.12250225675825E-17));
#13149=CARTESIAN_POINT('Ctrl Pts',(-7.67180517284341,-0.0510963299350149,
-3.17192231526653E-17));
#13150=CARTESIAN_POINT('Ctrl Pts',(-7.67210997162644,-0.0466786569219802,
1.16129547820002E-17));
#13151=CARTESIAN_POINT('Ctrl Pts',(-7.67230655013972,-0.0422481088180091,
1.04083408558608E-17));
#13152=CARTESIAN_POINT('Ctrl Pts',(-7.6725090500926,-0.0376841014537716,
9.16744092633848E-18));
#13153=CARTESIAN_POINT('Ctrl Pts',(-7.67259625011215,-0.0331162258874048,
8.24472046592442E-18));
#13154=CARTESIAN_POINT('Ctrl Pts',(-7.67256982465584,-0.0285510304520631,
1.04083408558608E-17));
#13155=CARTESIAN_POINT('Ctrl Pts',(-7.67247174711471,-0.0116074008728858,
1.84385737245866E-17));
#13156=CARTESIAN_POINT('Ctrl Pts',(-7.6708130923532,0.00531022346404731,
1.85851794107315E-17));
#13157=CARTESIAN_POINT('Ctrl Pts',(-7.66764846010905,0.0219708181576634,
3.46944695195361E-18));
#13158=CARTESIAN_POINT('Ctrl Pts',(-7.66599431782927,0.0306792531235465,
-4.43149389077601E-18));
#13159=CARTESIAN_POINT('Ctrl Pts',(-7.66392781727349,0.0393172333562807,
-5.69158656397132E-18));
#13160=CARTESIAN_POINT('Ctrl Pts',(-7.66145136629352,0.0478487584034829,
-3.46944695195361E-18));
#13161=CARTESIAN_POINT('Ctrl Pts',(-7.66000105406562,0.0528451727071283,
-2.16806999053646E-18));
#13162=CARTESIAN_POINT('Ctrl Pts',(-7.65840948355064,0.0578066853598702,
-4.88676934904438E-17));
#13163=CARTESIAN_POINT('Ctrl Pts',(-7.6566784834973,0.0627203082789222,
-2.42861286636753E-17));
#13164=CARTESIAN_POINT('Ctrl Pts',(-7.65135793333965,0.077823240913812,
5.12698762953888E-17));
#13165=CARTESIAN_POINT('Ctrl Pts',(-7.64474871423961,0.0924063141758472,
-3.57806052195261E-17));
#13166=CARTESIAN_POINT('Ctrl Pts',(-7.63687440208771,0.106254953674968,
-3.12250225675825E-17));
#13167=CARTESIAN_POINT('Ctrl Pts',(-7.63280782486428,0.113406887821882,
-2.88723562908995E-17));
#13168=CARTESIAN_POINT('Ctrl Pts',(-7.62839916570184,0.12036724850192,5.48664495430319E-17));
#13169=CARTESIAN_POINT('Ctrl Pts',(-7.62366911690659,0.127074854237358,
3.12250225675825E-17));
#13170=CARTESIAN_POINT('Ctrl Pts',(-7.61642299052403,0.137350468927051,
-4.9921022748546E-18));
#13171=CARTESIAN_POINT('Ctrl Pts',(-7.60841822005153,0.147045784154728,
-4.13752983739663E-17));
#13172=CARTESIAN_POINT('Ctrl Pts',(-7.59965866901871,0.156042617987613,
-3.46944695195361E-17));
#13173=CARTESIAN_POINT('Ctrl Pts',(-7.59707213175836,0.158699220574521,
-3.26179135892075E-17));
#13174=CARTESIAN_POINT('Ctrl Pts',(-7.59441969136407,0.161294781931434,
-1.60581715346596E-17));
#13175=CARTESIAN_POINT('Ctrl Pts',(-7.59170406260212,0.16382811505057,-1.38777878078145E-17));
#13176=CARTESIAN_POINT('Origin',(7.4,0.,0.220842344717745));
#13177=CARTESIAN_POINT('Ctrl Pts',(7.09227939521384,0.000154311006394908,
-0.0291576552822542));
#13178=CARTESIAN_POINT('Ctrl Pts',(7.09221571350587,0.0100435698963641,
-0.0296715621794889));
#13179=CARTESIAN_POINT('Ctrl Pts',(7.09709968515426,0.120578449441071,-0.035418806655132));
#13180=CARTESIAN_POINT('Ctrl Pts',(7.23047491327011,0.319794756266977,-0.0463993887091836));
#13181=CARTESIAN_POINT('Ctrl Pts',(7.5731988395346,0.317782877693097,-0.0620994014444088));
#13182=CARTESIAN_POINT('Ctrl Pts',(7.76060897472171,0.0308556191331042,
-0.0777994141796343));
#13183=CARTESIAN_POINT('Ctrl Pts',(7.62465992779684,-0.283761771610304,
-0.0934994269148594));
#13184=CARTESIAN_POINT('Ctrl Pts',(7.2872550057463,-0.343916549876741,-0.109199439650085));
#13185=CARTESIAN_POINT('Ctrl Pts',(7.10835469415216,-0.155985587810117,
-0.12108551577255));
#13186=CARTESIAN_POINT('Ctrl Pts',(7.09252332370173,-0.0276893492462785,
-0.127738254316606));
#13187=CARTESIAN_POINT('Ctrl Pts',(7.09275435891078,-0.000260665786541426,
-0.129157655282254));
#13188=CARTESIAN_POINT('Ctrl Pts',(7.09298021495369,-0.000306384811325677,
-0.0208423447177452));
#13189=CARTESIAN_POINT('Ctrl Pts',(7.09344513148094,0.0677879045700394,
-0.0243615716353137));
#13190=CARTESIAN_POINT('Ctrl Pts',(7.14897196854486,0.238050685086685,-0.0331141361312906));
#13191=CARTESIAN_POINT('Ctrl Pts',(7.42863574892529,0.360721777030891,-0.047100038205676));
#13192=CARTESIAN_POINT('Ctrl Pts',(7.71666223333994,0.175239166203998,-0.0628000509409013));
#13193=CARTESIAN_POINT('Ctrl Pts',(7.72085097116846,-0.167517439243982,
-0.0785000636761268));
#13194=CARTESIAN_POINT('Ctrl Pts',(7.43727190914667,-0.359992487166362,
-0.094200076411352));
#13195=CARTESIAN_POINT('Ctrl Pts',(7.15231797731739,-0.242854213543255,
-0.108314170091892));
#13196=CARTESIAN_POINT('Ctrl Pts',(7.09338979712027,-0.0702887118513222,
-0.117194926194023));
#13197=CARTESIAN_POINT('Ctrl Pts',(7.09284095646985,0.000245638412278346,
-0.120842344717745));
#13198=CARTESIAN_POINT('Ctrl Pts',(7.59134659966651,0.163598720337495,0.));
#13199=CARTESIAN_POINT('Ctrl Pts',(7.64514117960785,0.100680074451818,-0.00523333757840845));
#13200=CARTESIAN_POINT('Ctrl Pts',(7.68495172974597,-0.0813213515576848,
-0.0157000127352253));
#13201=CARTESIAN_POINT('Ctrl Pts',(7.48911277275958,-0.282913268514194,
-0.0314000254704507));
#13202=CARTESIAN_POINT('Ctrl Pts',(7.213305621753,-0.230208577870288,-0.047100038205676));
#13203=CARTESIAN_POINT('Ctrl Pts',(7.10494039731525,0.0286321757004985,
-0.0628000509409014));
#13204=CARTESIAN_POINT('Ctrl Pts',(7.26114221381406,0.261943484269437,-0.0785000636761267));
#13205=CARTESIAN_POINT('Ctrl Pts',(7.54186695250638,0.260295557049739,-0.094200076411352));
#13206=CARTESIAN_POINT('Ctrl Pts',(7.69537435948004,0.0252737989808328,
-0.109900089146577));
#13207=CARTESIAN_POINT('Ctrl Pts',(7.58401866543957,-0.232428911673642,
-0.125600101881803));
#13208=CARTESIAN_POINT('Ctrl Pts',(7.30765071643609,-0.281701615199185,
-0.141300114617028));
#13209=CARTESIAN_POINT('Ctrl Pts',(7.11409372805788,-0.0783741267420522,
-0.157000127352254));
#13210=CARTESIAN_POINT('Ctrl Pts',(7.17691140254618,0.195234349047302,-0.172700140087479));
#13211=CARTESIAN_POINT('Ctrl Pts',(7.43977487861582,0.293773242201156,-0.188400152822704));
#13212=CARTESIAN_POINT('Ctrl Pts',(7.66697178192527,0.128883380631593,-0.204100165557929));
#13213=CARTESIAN_POINT('Ctrl Pts',(7.65477255568824,-0.15157770749914,-0.219800178293155));
#13214=CARTESIAN_POINT('Ctrl Pts',(7.41411632045071,-0.29611748091033,-0.23550019102838));
#13215=CARTESIAN_POINT('Ctrl Pts',(7.16080185224803,-0.175125932931451,
-0.251200203763606));
#13216=CARTESIAN_POINT('Ctrl Pts',(7.12197865442297,0.102902751197641,-0.266900216498831));
#13217=CARTESIAN_POINT('Ctrl Pts',(7.33245986611545,0.288657535255061,-0.282600229234056));
#13218=CARTESIAN_POINT('Ctrl Pts',(7.60350496295894,0.215570346061205,-0.298300241969282));
#13219=CARTESIAN_POINT('Ctrl Pts',(7.69206520760226,-0.050820844434144,
-0.314000254704507));
#13220=CARTESIAN_POINT('Ctrl Pts',(7.51872777843214,-0.271640494238638,
-0.329700267439732));
#13221=CARTESIAN_POINT('Ctrl Pts',(7.23892601142296,-0.248877507817314,
-0.345400280174957));
#13222=CARTESIAN_POINT('Ctrl Pts',(7.10356083519368,-0.00294367203764689,
-0.361100292910183));
#13223=CARTESIAN_POINT('Ctrl Pts',(7.23401550197922,0.245629782461581,-0.376800305645408));
#13224=CARTESIAN_POINT('Ctrl Pts',(7.51331006051279,0.273944654681539,-0.392500318380634));
#13225=CARTESIAN_POINT('Ctrl Pts',(7.69099840073869,0.0566107268792646,
-0.408200331115859));
#13226=CARTESIAN_POINT('Ctrl Pts',(7.60774568331619,-0.21148658277481,-0.423900343851084));
#13227=CARTESIAN_POINT('Ctrl Pts',(7.33820541862493,-0.28994184478043,-0.43960035658631));
#13228=CARTESIAN_POINT('Ctrl Pts',(7.12407694792028,-0.108403472944119,
-0.455300369321535));
#13229=CARTESIAN_POINT('Ctrl Pts',(7.15737132502519,0.170341332964446,-0.47100038205676));
#13230=CARTESIAN_POINT('Ctrl Pts',(7.40823316280845,0.296339431604435,-0.486700394791985));
#13231=CARTESIAN_POINT('Ctrl Pts',(7.6517122442044,0.156607118609695,-0.502400407527211));
#13232=CARTESIAN_POINT('Ctrl Pts',(7.66947854203298,-0.123556299331602,
-0.518100420262436));
#13233=CARTESIAN_POINT('Ctrl Pts',(7.44560084469238,-0.292925599791504,
-0.533800432997662));
#13234=CARTESIAN_POINT('Ctrl Pts',(7.18083243499946,-0.199625701743059,
-0.549500445732886));
#13235=CARTESIAN_POINT('Ctrl Pts',(7.11259367828104,0.0726804721812103,
-0.565200458468113));
#13236=CARTESIAN_POINT('Ctrl Pts',(7.30207493790754,0.27981338153719,-0.580900471203337));
#13237=CARTESIAN_POINT('Ctrl Pts',(7.57936651916845,0.236034922850711,-0.596600483938564));
#13238=CARTESIAN_POINT('Ctrl Pts',(7.69581846427466,-0.0193982663347125,
-0.612300496673787));
#13239=CARTESIAN_POINT('Ctrl Pts',(7.54700706909094,-0.257436943317534,
-0.628000509409014));
#13240=CARTESIAN_POINT('Ctrl Pts',(7.26637319703535,-0.264629243152998,
-0.643700522144239));
#13241=CARTESIAN_POINT('Ctrl Pts',(7.1055634135989,-0.0345263660164505,
-0.659400534879464));
#13242=CARTESIAN_POINT('Ctrl Pts',(7.20877844294678,0.226537449876541,-0.67510054761469));
#13243=CARTESIAN_POINT('Ctrl Pts',(7.48346226287904,0.284461316975979,-0.690800560349915));
#13244=CARTESIAN_POINT('Ctrl Pts',(7.68330752343249,0.0873093086589616,
-0.706500573085141));
#13245=CARTESIAN_POINT('Ctrl Pts',(7.62910245608525,-0.188140484130538,
-0.722200585820366));
#13246=CARTESIAN_POINT('Ctrl Pts',(7.36947062435342,-0.294869405764503,
-0.737900598555591));
#13247=CARTESIAN_POINT('Ctrl Pts',(7.13719136614053,-0.137213321891836,
-0.753600611290817));
#13248=CARTESIAN_POINT('Ctrl Pts',(7.14062235409354,0.143538174106571,-0.769300624026041));
#13249=CARTESIAN_POINT('Ctrl Pts',(7.37654449298423,0.295466782201871,-0.785000636761268));
#13250=CARTESIAN_POINT('Ctrl Pts',(7.63369182760114,0.182672202271517,-0.800700649496493));
#13251=CARTESIAN_POINT('Ctrl Pts',(7.68089306428376,-0.0943914029012692,
-0.816400662231718));
#13252=CARTESIAN_POINT('Ctrl Pts',(7.54499195044998,-0.221828784507026,
-0.826867337388535));
#13253=CARTESIAN_POINT('Ctrl Pts',(7.46501999979751,-0.243208680203507,
-0.832100674966943));
#13254=CARTESIAN_POINT('Ctrl Pts',(7.60543315503421,0.175642532122685,0.0107002249889811));
#13255=CARTESIAN_POINT('Ctrl Pts',(7.66318798475343,0.108091940906,0.00546688741057261));
#13256=CARTESIAN_POINT('Ctrl Pts',(7.70592930826152,-0.0873080674088697,
-0.00499978774624429));
#13257=CARTESIAN_POINT('Ctrl Pts',(7.49567307751356,-0.303740779575947,
-0.0206998004814696));
#13258=CARTESIAN_POINT('Ctrl Pts',(7.19956155365563,-0.247156074632404,
-0.036399813216695));
#13259=CARTESIAN_POINT('Ctrl Pts',(7.08321869733608,0.0307400194197276,
-0.0520998259519203));
#13260=CARTESIAN_POINT('Ctrl Pts',(7.25091978029941,0.28122724160195,-0.0677998386871457));
#13261=CARTESIAN_POINT('Ctrl Pts',(7.55231091484912,0.279457997264192,-0.083499851422371));
#13262=CARTESIAN_POINT('Ctrl Pts',(7.71711923122726,0.0271344056982565,
-0.0991998641575963));
#13263=CARTESIAN_POINT('Ctrl Pts',(7.597565752892,-0.249539864985863,-0.114899876892822));
#13264=CARTESIAN_POINT('Ctrl Pts',(7.30085214620616,-0.302439926758371,
-0.130599889628047));
#13265=CARTESIAN_POINT('Ctrl Pts',(7.09304587804797,-0.084143873775297,
-0.146299902363272));
#13266=CARTESIAN_POINT('Ctrl Pts',(7.16048806455421,0.209607112777233,-0.161999915098498));
#13267=CARTESIAN_POINT('Ctrl Pts',(7.44270302591942,0.315400242884882,-0.177699927833723));
#13268=CARTESIAN_POINT('Ctrl Pts',(7.68662571251122,0.138371518285505,-0.193399940568948));
#13269=CARTESIAN_POINT('Ctrl Pts',(7.67352840354824,-0.162736556273655,
-0.209099953304174));
#13270=CARTESIAN_POINT('Ctrl Pts',(7.41515553583245,-0.317917059776419,
-0.224799966039399));
#13271=CARTESIAN_POINT('Ctrl Pts',(7.14319256126489,-0.188018355137328,
-0.240499978774624));
#13272=CARTESIAN_POINT('Ctrl Pts',(7.10151127697963,0.110478246684683,-0.25619999150985));
#13273=CARTESIAN_POINT('Ctrl Pts',(7.32748769604729,0.309907927787576,-0.271900004245075));
#13274=CARTESIAN_POINT('Ctrl Pts',(7.61848659280405,0.231440205367399,-0.2876000169803));
#13275=CARTESIAN_POINT('Ctrl Pts',(7.71356646618244,-0.0545621737297924,
-0.303300029715526));
#13276=CARTESIAN_POINT('Ctrl Pts',(7.52746828088937,-0.291638126121681,
-0.319000042450751));
#13277=CARTESIAN_POINT('Ctrl Pts',(7.2270680653589,-0.267199374000224,-0.334700055185976));
#13278=CARTESIAN_POINT('Ctrl Pts',(7.08173757460019,-0.0031603793071512,
-0.350400067921202));
#13279=CARTESIAN_POINT('Ctrl Pts',(7.22179605399517,0.263712557575601,-0.366100080656427));
#13280=CARTESIAN_POINT('Ctrl Pts',(7.52165172137279,0.294111914264847,-0.381800093391652));
#13281=CARTESIAN_POINT('Ctrl Pts',(7.71242112312342,0.060778295782922,-0.397500106126878));
#13282=CARTESIAN_POINT('Ctrl Pts',(7.62303950654344,-0.227055803565647,
-0.413200118862103));
#13283=CARTESIAN_POINT('Ctrl Pts',(7.33365622468325,-0.311286785620935,
-0.428900131597329));
#13284=CARTESIAN_POINT('Ctrl Pts',(7.10376404266291,-0.116383920604752,
-0.444600144332554));
#13285=CARTESIAN_POINT('Ctrl Pts',(7.13950948546398,0.182881522455109,-0.460300157067779));
#13286=CARTESIAN_POINT('Ctrl Pts',(7.40883927184805,0.31815535003834,-0.476000169803005));
#13287=CARTESIAN_POINT('Ctrl Pts',(7.67024279803129,0.168136222607972,-0.49170018253823));
#13288=CARTESIAN_POINT('Ctrl Pts',(7.68931701530281,-0.132652267875577,
-0.507400195273454));
#13289=CARTESIAN_POINT('Ctrl Pts',(7.44895788800903,-0.314490198730143,
-0.523100208008681));
#13290=CARTESIAN_POINT('Ctrl Pts',(7.1646977556032,-0.214321748107725,-0.538800220743906));
#13291=CARTESIAN_POINT('Ctrl Pts',(7.09143539759574,0.0780310637115318,
-0.554500233479131));
#13292=CARTESIAN_POINT('Ctrl Pts',(7.29486588997329,0.300412685096896,-0.570200246214357));
#13293=CARTESIAN_POINT('Ctrl Pts',(7.5925711248828,0.253411343520026,-0.585900258949582));
#13294=CARTESIAN_POINT('Ctrl Pts',(7.71759603013189,-0.0208263280470064,
-0.601600271684807));
#13295=CARTESIAN_POINT('Ctrl Pts',(7.55782943657383,-0.276388938085432,
-0.617300284420033));
#13296=CARTESIAN_POINT('Ctrl Pts',(7.25653585808158,-0.28411072070256,-0.633000297155258));
#13297=CARTESIAN_POINT('Ctrl Pts',(7.08388757883703,-0.0370681282812828,
-0.648700309890483));
#13298=CARTESIAN_POINT('Ctrl Pts',(7.19470109296709,0.243214685511279,-0.664400322625709));
#13299=CARTESIAN_POINT('Ctrl Pts',(7.48960658835547,0.305402792280665,-0.680100335360934));
#13300=CARTESIAN_POINT('Ctrl Pts',(7.70416405875568,0.0937368459796346,
-0.695800348096159));
#13301=CARTESIAN_POINT('Ctrl Pts',(7.64596852236574,-0.201991011661366,
-0.711500360831385));
#13302=CARTESIAN_POINT('Ctrl Pts',(7.36722311255473,-0.316577103825418,
-0.727200373566609));
#13303=CARTESIAN_POINT('Ctrl Pts',(7.1178439182192,-0.147314693222106,-0.742900386301836));
#13304=CARTESIAN_POINT('Ctrl Pts',(7.12152748866831,0.154105168453245,-0.758600399037061));
#13305=CARTESIAN_POINT('Ctrl Pts',(7.37481774529794,0.317218457925703,-0.774300411772286));
#13306=CARTESIAN_POINT('Ctrl Pts',(7.65089575426731,0.196120165788626,-0.790000424507512));
#13307=CARTESIAN_POINT('Ctrl Pts',(7.70157185193576,-0.101340309887447,
-0.805700437242737));
#13308=CARTESIAN_POINT('Ctrl Pts',(7.55566596891409,-0.2381593775803,-0.816167112399554));
#13309=CARTESIAN_POINT('Ctrl Pts',(7.4698066426161,-0.261113218593862,-0.821400449977962));
#13310=CARTESIAN_POINT('Ctrl Pts',(7.61951971040191,0.187686343907875,0.0214004499779621));
#13311=CARTESIAN_POINT('Ctrl Pts',(7.68123478989901,0.115503807360182,0.0161671123995537));
#13312=CARTESIAN_POINT('Ctrl Pts',(7.72690688677709,-0.0932947832600543,
0.00570043724273678));
#13313=CARTESIAN_POINT('Ctrl Pts',(7.50223338226752,-0.3245682906377,-0.00999957549248855));
#13314=CARTESIAN_POINT('Ctrl Pts',(7.18581748555827,-0.264103571394519,
-0.0256995882277139));
#13315=CARTESIAN_POINT('Ctrl Pts',(7.06149699735691,0.0328478631389564,
-0.0413996009629392));
#13316=CARTESIAN_POINT('Ctrl Pts',(7.24069734678476,0.300510998934463,-0.0570996136981646));
#13317=CARTESIAN_POINT('Ctrl Pts',(7.56275487719186,0.298620437478645,-0.0727996264333898));
#13318=CARTESIAN_POINT('Ctrl Pts',(7.73886410297448,0.0289950124156803,
-0.0884996391686154));
#13319=CARTESIAN_POINT('Ctrl Pts',(7.61111284034442,-0.266650818298083,
-0.104199651903841));
#13320=CARTESIAN_POINT('Ctrl Pts',(7.29405357597622,-0.323178238317556,
-0.119899664639066));
#13321=CARTESIAN_POINT('Ctrl Pts',(7.07199802803806,-0.0899136208085419,
-0.135599677374291));
#13322=CARTESIAN_POINT('Ctrl Pts',(7.14406472656225,0.223979876507163,-0.151299690109517));
#13323=CARTESIAN_POINT('Ctrl Pts',(7.44563117322301,0.337027243568608,-0.166999702844742));
#13324=CARTESIAN_POINT('Ctrl Pts',(7.70627964309719,0.147859655939416,-0.182699715579967));
#13325=CARTESIAN_POINT('Ctrl Pts',(7.69228425140824,-0.173895405048169,
-0.198399728315193));
#13326=CARTESIAN_POINT('Ctrl Pts',(7.41619475121419,-0.339716638642509,
-0.214099741050418));
#13327=CARTESIAN_POINT('Ctrl Pts',(7.12558327028176,-0.200910777343205,
-0.229799753785644));
#13328=CARTESIAN_POINT('Ctrl Pts',(7.08104389953629,0.118053742171726,-0.245499766520869));
#13329=CARTESIAN_POINT('Ctrl Pts',(7.32251552597912,0.33115832032009,-0.261199779256094));
#13330=CARTESIAN_POINT('Ctrl Pts',(7.63346822264916,0.247310064673594,-0.276899791991319));
#13331=CARTESIAN_POINT('Ctrl Pts',(7.73506772476262,-0.0583035030254407,
-0.292599804726545));
#13332=CARTESIAN_POINT('Ctrl Pts',(7.53620878334662,-0.311635758004724,
-0.30829981746177));
#13333=CARTESIAN_POINT('Ctrl Pts',(7.21521011929483,-0.285521240183133,
-0.323999830196995));
#13334=CARTESIAN_POINT('Ctrl Pts',(7.05991431400671,-0.00337708657665555,
-0.339699842932221));
#13335=CARTESIAN_POINT('Ctrl Pts',(7.20957660601111,0.281795332689621,-0.355399855667446));
#13336=CARTESIAN_POINT('Ctrl Pts',(7.52999338223278,0.314279173848155,-0.371099868402671));
#13337=CARTESIAN_POINT('Ctrl Pts',(7.73384384550816,0.0649458646865791,
-0.386799881137897));
#13338=CARTESIAN_POINT('Ctrl Pts',(7.63833332977069,-0.242625024356483,
-0.402499893873122));
#13339=CARTESIAN_POINT('Ctrl Pts',(7.32910703074157,-0.332631726461441,
-0.418199906608347));
#13340=CARTESIAN_POINT('Ctrl Pts',(7.08345113740554,-0.124364368265385,
-0.433899919343573));
#13341=CARTESIAN_POINT('Ctrl Pts',(7.12164764590278,0.195421711945772,-0.449599932078798));
#13342=CARTESIAN_POINT('Ctrl Pts',(7.40944538088764,0.339971268472245,-0.465299944814024));
#13343=CARTESIAN_POINT('Ctrl Pts',(7.68877335185819,0.17966532660625,-0.480999957549249));
#13344=CARTESIAN_POINT('Ctrl Pts',(7.70915548857264,-0.141748236419551,
-0.496699970284474));
#13345=CARTESIAN_POINT('Ctrl Pts',(7.45231493132566,-0.336054797668783,
-0.5123999830197));
#13346=CARTESIAN_POINT('Ctrl Pts',(7.14856307620694,-0.229017794472391,
-0.528099995754925));
#13347=CARTESIAN_POINT('Ctrl Pts',(7.07027711691044,0.0833816552418533,
-0.543800008490151));
#13348=CARTESIAN_POINT('Ctrl Pts',(7.28765684203904,0.321011988656602,-0.559500021225375));
#13349=CARTESIAN_POINT('Ctrl Pts',(7.60577573059716,0.27078776418934,-0.575200033960601));
#13350=CARTESIAN_POINT('Ctrl Pts',(7.73937359598911,-0.0222543897593003,
-0.590900046695826));
#13351=CARTESIAN_POINT('Ctrl Pts',(7.56865180405673,-0.29534093285333,-0.606600059431052));
#13352=CARTESIAN_POINT('Ctrl Pts',(7.24669851912781,-0.303592198252122,
-0.622300072166277));
#13353=CARTESIAN_POINT('Ctrl Pts',(7.06221174407517,-0.0396098905461152,
-0.638000084901503));
#13354=CARTESIAN_POINT('Ctrl Pts',(7.1806237429874,0.259891921146016,-0.653700097636727));
#13355=CARTESIAN_POINT('Ctrl Pts',(7.4957509138319,0.326344267585352,-0.669400110371953));
#13356=CARTESIAN_POINT('Ctrl Pts',(7.72502059407888,0.100164383300307,-0.685100123107178));
#13357=CARTESIAN_POINT('Ctrl Pts',(7.66283458864623,-0.215841539192194,
-0.700800135842403));
#13358=CARTESIAN_POINT('Ctrl Pts',(7.36497560075606,-0.338284801886334,
-0.71650014857763));
#13359=CARTESIAN_POINT('Ctrl Pts',(7.09849647029787,-0.157416064552375,
-0.732200161312854));
#13360=CARTESIAN_POINT('Ctrl Pts',(7.10243262324309,0.164672162799918,-0.74790017404808));
#13361=CARTESIAN_POINT('Ctrl Pts',(7.37309099761164,0.338970133649535,-0.763600186783305));
#13362=CARTESIAN_POINT('Ctrl Pts',(7.66809968093348,0.209568129305734,-0.77930019951853));
#13363=CARTESIAN_POINT('Ctrl Pts',(7.72225063958776,-0.108289216873624,
-0.795000212253756));
#13364=CARTESIAN_POINT('Ctrl Pts',(7.5663399873782,-0.254489970653575,-0.805466887410573));
#13365=CARTESIAN_POINT('Ctrl Pts',(7.47459328543469,-0.279017756984216,
-0.810700224988981));
#13366=CARTESIAN_POINT('Ctrl Pts',(7.63360626576962,0.199730155693065,0.0321006749669432));
#13367=CARTESIAN_POINT('Ctrl Pts',(7.69928159504458,0.122915673814364,0.0268673373885347));
#13368=CARTESIAN_POINT('Ctrl Pts',(7.74788446529264,-0.0992814991112389,
0.0164006622317179));
#13369=CARTESIAN_POINT('Ctrl Pts',(7.50879368702149,-0.345395801699454,
0.000700649496492501));
#13370=CARTESIAN_POINT('Ctrl Pts',(7.17207341746091,-0.281051068156635,
-0.0149993632387328));
#13371=CARTESIAN_POINT('Ctrl Pts',(7.03977529737773,0.0349557068581856,
-0.0306993759739581));
#13372=CARTESIAN_POINT('Ctrl Pts',(7.23047491327011,0.319794756266977,-0.0463993887091836));
#13373=CARTESIAN_POINT('Ctrl Pts',(7.5731988395346,0.317782877693097,-0.0620994014444088));
#13374=CARTESIAN_POINT('Ctrl Pts',(7.76060897472171,0.0308556191331042,
-0.0777994141796343));
#13375=CARTESIAN_POINT('Ctrl Pts',(7.62465992779684,-0.283761771610304,
-0.0934994269148594));
#13376=CARTESIAN_POINT('Ctrl Pts',(7.2872550057463,-0.343916549876741,-0.109199439650085));
#13377=CARTESIAN_POINT('Ctrl Pts',(7.05095017802815,-0.0956833678417867,
-0.12489945238531));
#13378=CARTESIAN_POINT('Ctrl Pts',(7.12764138857029,0.238352640237094,-0.140599465120536));
#13379=CARTESIAN_POINT('Ctrl Pts',(7.4485593205266,0.358654244252335,-0.156299477855761));
#13380=CARTESIAN_POINT('Ctrl Pts',(7.72593357368315,0.157347793593328,-0.171999490590986));
#13381=CARTESIAN_POINT('Ctrl Pts',(7.71104009926825,-0.185054253822684,
-0.187699503326212));
#13382=CARTESIAN_POINT('Ctrl Pts',(7.41723396659593,-0.361516217508599,
-0.203399516061437));
#13383=CARTESIAN_POINT('Ctrl Pts',(7.10797397929862,-0.213803199549082,
-0.219099528796662));
#13384=CARTESIAN_POINT('Ctrl Pts',(7.06057652209295,0.125629237658768,-0.234799541531888));
#13385=CARTESIAN_POINT('Ctrl Pts',(7.31754335591095,0.352408712852604,-0.250499554267113));
#13386=CARTESIAN_POINT('Ctrl Pts',(7.64844985249427,0.263179923979787,-0.266199567002338));
#13387=CARTESIAN_POINT('Ctrl Pts',(7.75656898334281,-0.062044832321089,
-0.281899579737564));
#13388=CARTESIAN_POINT('Ctrl Pts',(7.54494928580385,-0.331633389887768,
-0.297599592472789));
#13389=CARTESIAN_POINT('Ctrl Pts',(7.20335217323078,-0.303843106366043,
-0.313299605208014));
#13390=CARTESIAN_POINT('Ctrl Pts',(7.03809105341322,-0.00359379384616002,
-0.32899961794324));
#13391=CARTESIAN_POINT('Ctrl Pts',(7.19735715802706,0.299878107803642,-0.344699630678465));
#13392=CARTESIAN_POINT('Ctrl Pts',(7.53833504309277,0.334446433431464,-0.36039964341369));
#13393=CARTESIAN_POINT('Ctrl Pts',(7.75526656789289,0.0691134335902364,
-0.376099656148916));
#13394=CARTESIAN_POINT('Ctrl Pts',(7.65362715299794,-0.25819424514732,-0.391799668884141));
#13395=CARTESIAN_POINT('Ctrl Pts',(7.32455783679988,-0.353976667301946,
-0.407499681619366));
#13396=CARTESIAN_POINT('Ctrl Pts',(7.06313823214816,-0.132344815926019,
-0.423199694354592));
#13397=CARTESIAN_POINT('Ctrl Pts',(7.10378580634158,0.207961901436435,-0.438899707089817));
#13398=CARTESIAN_POINT('Ctrl Pts',(7.41005148992723,0.36178718690615,-0.454599719825043));
#13399=CARTESIAN_POINT('Ctrl Pts',(7.70730390568508,0.191194430604527,-0.470299732560268));
#13400=CARTESIAN_POINT('Ctrl Pts',(7.72899396184246,-0.150844204963527,
-0.485999745295493));
#13401=CARTESIAN_POINT('Ctrl Pts',(7.45567197464232,-0.357619396607422,
-0.501699758030719));
#13402=CARTESIAN_POINT('Ctrl Pts',(7.13242839681067,-0.243713840837058,
-0.517399770765943));
#13403=CARTESIAN_POINT('Ctrl Pts',(7.04911883622514,0.088732246772175,-0.533099783501169));
#13404=CARTESIAN_POINT('Ctrl Pts',(7.28044779410479,0.341611292216308,-0.548799796236394));
#13405=CARTESIAN_POINT('Ctrl Pts',(7.61898033631151,0.288164184858654,-0.564499808971621));
#13406=CARTESIAN_POINT('Ctrl Pts',(7.76115116184634,-0.0236824514715945,
-0.580199821706845));
#13407=CARTESIAN_POINT('Ctrl Pts',(7.57947417153963,-0.314292927621228,
-0.595899834442071));
#13408=CARTESIAN_POINT('Ctrl Pts',(7.23686118017403,-0.323073675801685,
-0.611599847177295));
#13409=CARTESIAN_POINT('Ctrl Pts',(7.0405359093133,-0.0421516528109474,
-0.627299859912522));
#13410=CARTESIAN_POINT('Ctrl Pts',(7.16654639300772,0.276569156780754,-0.642999872647746));
#13411=CARTESIAN_POINT('Ctrl Pts',(7.50189523930833,0.347285742890038,-0.658699885382972));
#13412=CARTESIAN_POINT('Ctrl Pts',(7.74587712940208,0.10659192062098,-0.674399898118197));
#13413=CARTESIAN_POINT('Ctrl Pts',(7.67970065492672,-0.229692066723022,
-0.690099910853423));
#13414=CARTESIAN_POINT('Ctrl Pts',(7.36272808895739,-0.359992499947249,
-0.705799923588647));
#13415=CARTESIAN_POINT('Ctrl Pts',(7.07914902237653,-0.167517435882645,
-0.721499936323874));
#13416=CARTESIAN_POINT('Ctrl Pts',(7.08333775781787,0.175239157146592,-0.737199949059098));
#13417=CARTESIAN_POINT('Ctrl Pts',(7.37136424992534,0.360721809373367,-0.752899961794324));
#13418=CARTESIAN_POINT('Ctrl Pts',(7.68530360759964,0.223016092822843,-0.768599974529549));
#13419=CARTESIAN_POINT('Ctrl Pts',(7.74292942723977,-0.115238123859802,
-0.784299987264775));
#13420=CARTESIAN_POINT('Ctrl Pts',(7.57701400584231,-0.270820563726849,
-0.794766662421592));
#13421=CARTESIAN_POINT('Ctrl Pts',(7.47937992825329,-0.29692229537457,-0.8));
#13422=CARTESIAN_POINT('Ctrl Pts',(7.59134659966651,0.163598720337495,0.));
#13423=CARTESIAN_POINT('Ctrl Pts',(7.60250981747379,0.153108036753198,-2.76372047324665E-18));
#13424=CARTESIAN_POINT('Ctrl Pts',(7.61257002986606,0.141586745509806,-2.10635142953706E-17));
#13425=CARTESIAN_POINT('Ctrl Pts',(7.62152230270038,0.129252348737935,-1.17093834628434E-17));
#13426=CARTESIAN_POINT('Ctrl Pts',(7.62952885125357,0.118220966154305,-3.34342946773069E-18));
#13427=CARTESIAN_POINT('Ctrl Pts',(7.63664920495495,0.106537870238012,-2.15761777783297E-17));
#13428=CARTESIAN_POINT('Ctrl Pts',(7.64286041237134,0.0943311530405987,
-2.77555756156289E-17));
#13429=CARTESIAN_POINT('Ctrl Pts',(7.64494079815862,0.0902426273700751,
-2.98253070821307E-17));
#13430=CARTESIAN_POINT('Ctrl Pts',(7.64691967101295,0.0860937108205726,
2.22114370828616E-17));
#13431=CARTESIAN_POINT('Ctrl Pts',(7.64879354491767,0.081893408177734,1.64798730217797E-17));
#13432=CARTESIAN_POINT('Ctrl Pts',(7.655493762727,0.0668748188792052,-4.01388992607871E-18));
#13433=CARTESIAN_POINT('Ctrl Pts',(7.6608110935522,0.0513021332299394,3.07095711685637E-17));
#13434=CARTESIAN_POINT('Ctrl Pts',(7.66472282738542,0.0354014324049846,
3.46944695195361E-17));
#13435=CARTESIAN_POINT('Ctrl Pts',(7.66742756504633,0.0244070176033393,
3.74497962120694E-17));
#13436=CARTESIAN_POINT('Ctrl Pts',(7.66945962470024,0.0132547133788681,
7.12360322228779E-17));
#13437=CARTESIAN_POINT('Ctrl Pts',(7.67079967407203,0.00201093560136876,
9.19403442267708E-17));
#13438=CARTESIAN_POINT('Ctrl Pts',(7.67155462684706,-0.00432354834646305,
1.03604674012976E-16));
#13439=CARTESIAN_POINT('Ctrl Pts',(7.67208975223811,-0.0106871591093033,
5.10024386813213E-17));
#13440=CARTESIAN_POINT('Ctrl Pts',(7.67239999929748,-0.017068447894435,
6.07153216591882E-17));
#13441=CARTESIAN_POINT('Ctrl Pts',(7.67261026346053,-0.0213932474537081,
6.72980470985737E-17));
#13442=CARTESIAN_POINT('Ctrl Pts',(7.67271673802996,-0.0257170992981115,
4.2195820725283E-17));
#13443=CARTESIAN_POINT('Ctrl Pts',(7.67271892939023,-0.0300345419010102,
4.33680868994202E-17));
#13444=CARTESIAN_POINT('Ctrl Pts',(7.67272693146828,-0.0458003258944295,
4.76487912385652E-17));
#13445=CARTESIAN_POINT('Ctrl Pts',(7.67134758489843,-0.0614867913330191,
6.01689604624523E-17));
#13446=CARTESIAN_POINT('Ctrl Pts',(7.66853812911313,-0.0769181334380825,
6.93889390390723E-17));
#13447=CARTESIAN_POINT('Ctrl Pts',(7.6662196457605,-0.0896527384696332,
7.30753135663338E-17));
#13448=CARTESIAN_POINT('Ctrl Pts',(7.66292674408646,-0.102214296971847,
6.38087454160287E-17));
#13449=CARTESIAN_POINT('Ctrl Pts',(7.65873262674493,-0.114535513997406,
6.24500451351651E-17));
#13450=CARTESIAN_POINT('Ctrl Pts',(7.65678779272614,-0.120248926396956,
6.18200087502971E-17));
#13451=CARTESIAN_POINT('Ctrl Pts',(7.65464687544019,-0.125914602381379,
5.65864599207131E-17));
#13452=CARTESIAN_POINT('Ctrl Pts',(7.65232789334325,-0.131499045448586,
5.89805981832114E-17));
#13453=CARTESIAN_POINT('Ctrl Pts',(7.64581346085479,-0.147186737645481,
6.57061576860812E-17));
#13454=CARTESIAN_POINT('Ctrl Pts',(7.63788690776836,-0.162272369755971,
2.69522798546906E-17));
#13455=CARTESIAN_POINT('Ctrl Pts',(7.62872587899731,-0.176613455703731,
2.08166817117217E-17));
#13456=CARTESIAN_POINT('Ctrl Pts',(7.62337452143084,-0.184990711219019,
1.7232610493544E-17));
#13457=CARTESIAN_POINT('Ctrl Pts',(7.61760089383393,-0.193113914513073,
7.21698909598366E-17));
#13458=CARTESIAN_POINT('Ctrl Pts',(7.61143279113021,-0.200952905400778,
8.32667268468867E-17));
#13459=CARTESIAN_POINT('Ctrl Pts',(7.60742014858138,-0.20605253974327,9.04857434516068E-17));
#13460=CARTESIAN_POINT('Ctrl Pts',(7.60324045059445,-0.211031857377795,
2.3759156340358E-17));
#13461=CARTESIAN_POINT('Ctrl Pts',(7.59890027835381,-0.215881931042746,
1.73472347597681E-17));
#13462=CARTESIAN_POINT('Ctrl Pts',(7.59567072863155,-0.219490901652473,
1.25760831990297E-17));
#13463=CARTESIAN_POINT('Ctrl Pts',(7.59235503385033,-0.22302506289888,3.58617524316929E-17));
#13464=CARTESIAN_POINT('Ctrl Pts',(7.58896204714281,-0.226475380907007,
3.81639164714898E-17));
#13465=CARTESIAN_POINT('Ctrl Pts',(7.57975197943177,-0.235841071143565,
4.44130086478315E-17));
#13466=CARTESIAN_POINT('Ctrl Pts',(7.56996175646191,-0.244602587321019,
6.41428917201894E-17));
#13467=CARTESIAN_POINT('Ctrl Pts',(7.5596547346654,-0.252692752680651,5.89805981832114E-17));
#13468=CARTESIAN_POINT('Ctrl Pts',(7.55492270000885,-0.256407011136178,
5.66105486765211E-17));
#13469=CARTESIAN_POINT('Ctrl Pts',(7.55008155466001,-0.259979662792626,
6.18911852966909E-17));
#13470=CARTESIAN_POINT('Ctrl Pts',(7.5451366005002,-0.263403568695713,5.89805981832114E-17));
#13471=CARTESIAN_POINT('Ctrl Pts',(7.53997605228505,-0.266976752779113,
5.59431129714072E-17));
#13472=CARTESIAN_POINT('Ctrl Pts',(7.53470889794899,-0.270383320907462,
7.04757199048251E-17));
#13473=CARTESIAN_POINT('Ctrl Pts',(7.5293467893667,-0.273613072908771,6.59194920871187E-17));
#13474=CARTESIAN_POINT('Ctrl Pts',(7.51740496593982,-0.280805976133378,
5.57724263840117E-17));
#13475=CARTESIAN_POINT('Ctrl Pts',(7.50498570886338,-0.287127913581425,
1.04560758728475E-17));
#13476=CARTESIAN_POINT('Ctrl Pts',(7.4921567849037,-0.292493152066132,-6.93889390390723E-18));
#13477=CARTESIAN_POINT('Ctrl Pts',(7.48800667626404,-0.294228786532378,
-5.43963370827884E-18));
#13478=CARTESIAN_POINT('Ctrl Pts',(7.48381360175906,-0.295864191924157,
9.75249754612042E-18));
#13479=CARTESIAN_POINT('Ctrl Pts',(7.47958090815733,-0.297400289619931,
6.93889390390723E-18));
#13480=CARTESIAN_POINT('Ctrl Pts',(7.1483354802531,-0.000213511019231185,
-0.161258330249198));
#13481=CARTESIAN_POINT('Ctrl Pts',(7.14814623960277,-0.0226803112827391,
-0.15983892928355));
#13482=CARTESIAN_POINT('Ctrl Pts',(7.15091292268037,-0.0451013034050039,
-0.158419528317902));
#13483=CARTESIAN_POINT('Ctrl Pts',(7.15682283853563,-0.0666606288533484,
-0.157000127352254));
#13484=CARTESIAN_POINT('Ctrl Pts',(7.17861272418395,-0.146149956227763,
-0.151766789773846));
#13485=CARTESIAN_POINT('Ctrl Pts',(7.24313172031002,-0.213925785713474,
-0.146533452195437));
#13486=CARTESIAN_POINT('Ctrl Pts',(7.32145254320697,-0.239601583202072,
-0.141300114617029));
#13487=CARTESIAN_POINT('Ctrl Pts',(7.39977336610391,-0.26527738069067,-0.13606677703862));
#13488=CARTESIAN_POINT('Ctrl Pts',(7.49189601577174,-0.248853146182156,
-0.130833439460212));
#13489=CARTESIAN_POINT('Ctrl Pts',(7.55651662294573,-0.197690577152153,
-0.125600101881803));
#13490=CARTESIAN_POINT('Ctrl Pts',(7.62113723011973,-0.14652800812215,-0.120366764303395));
#13491=CARTESIAN_POINT('Ctrl Pts',(7.65825579479988,-0.0606271045706585,
-0.115133426724986));
#13492=CARTESIAN_POINT('Ctrl Pts',(7.65123050931102,0.0214936402165713,
-0.109900089146578));
#13493=CARTESIAN_POINT('Ctrl Pts',(7.64420522382215,0.103614385003801,-0.104666751568169));
#13494=CARTESIAN_POINT('Ctrl Pts',(7.59303608816426,0.18195497102677,-0.099433413989761));
#13495=CARTESIAN_POINT('Ctrl Pts',(7.5206640638866,0.22139991857487,-0.0942000764113525));
#13496=CARTESIAN_POINT('Ctrl Pts',(7.44829203960894,0.260844866122971,-0.0889667388329441));
#13497=CARTESIAN_POINT('Ctrl Pts',(7.3547171267115,0.261394175196203,-0.0837334012545357));
#13498=CARTESIAN_POINT('Ctrl Pts',(7.28189603417964,0.222783611637997,-0.0785000636761272));
#13499=CARTESIAN_POINT('Ctrl Pts',(7.20907494164779,0.18417304807979,-0.0732667260977188));
#13500=CARTESIAN_POINT('Ctrl Pts',(7.15700766948152,0.106402611890144,-0.0680333885193103));
#13501=CARTESIAN_POINT('Ctrl Pts',(7.14903490413801,0.0243772682001904,
-0.0628000509409019));
#13502=CARTESIAN_POINT('Ctrl Pts',(7.14825198902148,0.0163224868606074,
-0.0622861440436673));
#13503=CARTESIAN_POINT('Ctrl Pts',(7.14789427647666,0.00822667552110126,
-0.0617722371464327));
#13504=CARTESIAN_POINT('Ctrl Pts',(7.14794643808389,0.00012639595204536,
-0.0612583302491982));
#13505=CARTESIAN_POINT('Ctrl Pts',(7.32062007174671,-0.29692229537457,0.));
#13506=CARTESIAN_POINT('Ctrl Pts',(7.22298599415769,-0.270820563726849,
-0.00523333757840845));
#13507=CARTESIAN_POINT('Ctrl Pts',(7.05707055753998,-0.115238222676569,
-0.0157000127352254));
#13508=CARTESIAN_POINT('Ctrl Pts',(7.11469640556356,0.223016129191749,-0.0314000254704506));
#13509=CARTESIAN_POINT('Ctrl Pts',(7.42863574892529,0.360721777030891,-0.047100038205676));
#13510=CARTESIAN_POINT('Ctrl Pts',(7.71666223333994,0.175239166203998,-0.0628000509409013));
#13511=CARTESIAN_POINT('Ctrl Pts',(7.72085097116846,-0.167517439243982,
-0.0785000636761268));
#13512=CARTESIAN_POINT('Ctrl Pts',(7.43727190914667,-0.359992487166362,
-0.094200076411352));
#13513=CARTESIAN_POINT('Ctrl Pts',(7.12029935249992,-0.229692063399103,
-0.109900089146577));
#13514=CARTESIAN_POINT('Ctrl Pts',(7.05412287853826,0.106591919249608,-0.125600101881803));
#13515=CARTESIAN_POINT('Ctrl Pts',(7.2981047634038,0.347285733851148,-0.141300114617028));
#13516=CARTESIAN_POINT('Ctrl Pts',(7.63345360120587,0.276569150443068,-0.157000127352253));
#13517=CARTESIAN_POINT('Ctrl Pts',(7.75946408208296,-0.0421516519758924,
-0.172700140087479));
#13518=CARTESIAN_POINT('Ctrl Pts',(7.56313881583769,-0.323073667897745,
-0.188400152822704));
#13519=CARTESIAN_POINT('Ctrl Pts',(7.22052583282271,-0.314292920077652,
-0.20410016555793));
#13520=CARTESIAN_POINT('Ctrl Pts',(7.03884884686676,-0.023682450872479,
-0.219800178293155));
#13521=CARTESIAN_POINT('Ctrl Pts',(7.18101966898755,0.28816417788129,-0.23550019102838));
#13522=CARTESIAN_POINT('Ctrl Pts',(7.51955220300225,0.341611283968803,-0.251200203763605));
#13523=CARTESIAN_POINT('Ctrl Pts',(7.7508811552982,0.0887322446241938,-0.266900216498831));
#13524=CARTESIAN_POINT('Ctrl Pts',(7.66757159672246,-0.243713834945875,
-0.282600229234056));
#13525=CARTESIAN_POINT('Ctrl Pts',(7.34432802670357,-0.357619387966788,
-0.298300241969282));
#13526=CARTESIAN_POINT('Ctrl Pts',(7.07100604610717,-0.150844201317933,
-0.314000254704507));
#13527=CARTESIAN_POINT('Ctrl Pts',(7.0926961017409,0.191194425984153,-0.329700267439732));
#13528=CARTESIAN_POINT('Ctrl Pts',(7.38994851031558,0.361787178163918,-0.345400280174957));
#13529=CARTESIAN_POINT('Ctrl Pts',(7.69621418650062,0.207961896411083,-0.361100292910183));
#13530=CARTESIAN_POINT('Ctrl Pts',(7.73686175971175,-0.132344812727946,
-0.376800305645408));
#13531=CARTESIAN_POINT('Ctrl Pts',(7.47544216137711,-0.353976658748332,
-0.392500318380634));
#13532=CARTESIAN_POINT('Ctrl Pts',(7.14637285313081,-0.258194238908191,
-0.408200331115859));
#13533=CARTESIAN_POINT('Ctrl Pts',(7.04473344069191,0.0691134319201361,
-0.423900343851084));
#13534=CARTESIAN_POINT('Ctrl Pts',(7.26166496025002,0.334446425349789,-0.43960035658631));
#13535=CARTESIAN_POINT('Ctrl Pts',(7.60264283707619,0.299878100557217,-0.455300369321535));
#13536=CARTESIAN_POINT('Ctrl Pts',(7.76190893784147,-0.00359379375923244,
-0.47100038205676));
#13537=CARTESIAN_POINT('Ctrl Pts',(7.59664782201734,-0.303843099024022,
-0.486700394791986));
#13538=CARTESIAN_POINT('Ctrl Pts',(7.25505071769875,-0.33163338187372,-0.502400407527211));
#13539=CARTESIAN_POINT('Ctrl Pts',(7.0434310252735,-0.0620448308224301,
-0.518100420262436));
#13540=CARTESIAN_POINT('Ctrl Pts',(7.1515501535093,0.263179917621393,-0.533800432997662));
#13541=CARTESIAN_POINT('Ctrl Pts',(7.4824566420967,0.352408704334569,-0.549500445732887));
#13542=CARTESIAN_POINT('Ctrl Pts',(7.73942346970471,0.125629234627381,-0.565200458468113));
#13543=CARTESIAN_POINT('Ctrl Pts',(7.69202601364555,-0.213803194390989,
-0.580900471203338));
#13544=CARTESIAN_POINT('Ctrl Pts',(7.38276603381877,-0.361516208756931,
-0.596600483938563));
#13545=CARTESIAN_POINT('Ctrl Pts',(7.08895990825159,-0.185054249380952,
-0.612300496673788));
#13546=CARTESIAN_POINT('Ctrl Pts',(7.07406643418487,0.157347789847665,-0.628000509409014));
#13547=CARTESIAN_POINT('Ctrl Pts',(7.35144068066377,0.358654235479558,-0.643700522144239));
#13548=CARTESIAN_POINT('Ctrl Pts',(7.67235860481237,0.238352634675404,-0.659400534879465));
#13549=CARTESIAN_POINT('Ctrl Pts',(7.74904981361332,-0.0956833658965494,
-0.675100547614689));
#13550=CARTESIAN_POINT('Ctrl Pts',(7.51274499136877,-0.343916540891515,
-0.690800560349916));
#13551=CARTESIAN_POINT('Ctrl Pts',(7.17534007797001,-0.283761765982407,
-0.70650057308514));
#13552=CARTESIAN_POINT('Ctrl Pts',(7.03939103328141,0.0308556206006142,
-0.722200585820366));
#13553=CARTESIAN_POINT('Ctrl Pts',(7.22680116614257,0.317782866086405,-0.737900598555591));
#13554=CARTESIAN_POINT('Ctrl Pts',(7.56952507950631,0.319794755380677,-0.753600611290817));
#13555=CARTESIAN_POINT('Ctrl Pts',(7.76022470046591,0.0349556943853752,
-0.769300624026041));
#13556=CARTESIAN_POINT('Ctrl Pts',(7.62792656327177,-0.28105104215419,-0.785000636761267));
#13557=CARTESIAN_POINT('Ctrl Pts',(7.29120634442719,-0.345395824214954,
-0.800700649496492));
#13558=CARTESIAN_POINT('Ctrl Pts',(7.0521154661904,-0.099281426297527,-0.816400662231718));
#13559=CARTESIAN_POINT('Ctrl Pts',(7.10071840495542,0.122915673814367,-0.826867337388535));
#13560=CARTESIAN_POINT('Ctrl Pts',(7.16639373423039,0.199730155693067,-0.832100674966943));
#13561=CARTESIAN_POINT('Ctrl Pts',(7.32540671456531,-0.279017756984216,
0.0107002249889811));
#13562=CARTESIAN_POINT('Ctrl Pts',(7.2336600126218,-0.254489970653575,0.00546688741057261));
#13563=CARTESIAN_POINT('Ctrl Pts',(7.07774934610977,-0.108289309731699,
-0.00499978774624428));
#13564=CARTESIAN_POINT('Ctrl Pts',(7.13190033143599,0.20956816348158,-0.0206998004814696));
#13565=CARTESIAN_POINT('Ctrl Pts',(7.42690900130829,0.338970103257324,-0.036399813216695));
#13566=CARTESIAN_POINT('Ctrl Pts',(7.69756736844791,0.164672171311159,-0.0520998259519203));
#13567=CARTESIAN_POINT('Ctrl Pts',(7.70150352363636,-0.157416067711022,
-0.0677998386871457));
#13568=CARTESIAN_POINT('Ctrl Pts',(7.43502439746233,-0.338284789876139,
-0.0834998514223709));
#13569=CARTESIAN_POINT('Ctrl Pts',(7.13716541833258,-0.215841536068708,
-0.0991998641575964));
#13570=CARTESIAN_POINT('Ctrl Pts',(7.07497941338266,0.10016438201163,-0.114899876892821));
#13571=CARTESIAN_POINT('Ctrl Pts',(7.30424908871668,0.32634425909151,-0.130599889628047));
#13572=CARTESIAN_POINT('Ctrl Pts',(7.61937625157511,0.259891915190496,-0.146299902363272));
#13573=CARTESIAN_POINT('Ctrl Pts',(7.7377882478399,-0.0396098897614143,
-0.161999915098498));
#13574=CARTESIAN_POINT('Ctrl Pts',(7.5533014771244,-0.303592190824794,-0.177699927833723));
#13575=CARTESIAN_POINT('Ctrl Pts',(7.23134820004257,-0.295340925764635,
-0.193399940568948));
#13576=CARTESIAN_POINT('Ctrl Pts',(7.06062641219857,-0.022254389196312,
-0.209099953304174));
#13577=CARTESIAN_POINT('Ctrl Pts',(7.19422427438237,0.270787757632714,-0.224799966039399));
#13578=CARTESIAN_POINT('Ctrl Pts',(7.51234315524245,0.321011980906425,-0.240499978774625));
#13579=CARTESIAN_POINT('Ctrl Pts',(7.72972287512404,0.0833816532233965,
-0.25619999150985));
#13580=CARTESIAN_POINT('Ctrl Pts',(7.65143691771615,-0.22901778893645,-0.271900004245075));
#13581=CARTESIAN_POINT('Ctrl Pts',(7.34768506993906,-0.336054789549182,
-0.2876000169803));
#13582=CARTESIAN_POINT('Ctrl Pts',(7.09084451889762,-0.141748232993789,
-0.303300029715526));
#13583=CARTESIAN_POINT('Ctrl Pts',(7.11122665512001,0.179665322264485,-0.319000042450751));
#13584=CARTESIAN_POINT('Ctrl Pts',(7.39055461934053,0.339971260257174,-0.334700055185976));
#13585=CARTESIAN_POINT('Ctrl Pts',(7.67835234737104,0.195421707223451,-0.350400067921202));
#13586=CARTESIAN_POINT('Ctrl Pts',(7.71654885494523,-0.124364365260158,
-0.366100080656428));
#13587=CARTESIAN_POINT('Ctrl Pts',(7.47089296754535,-0.332631718423613,
-0.381800093391652));
#13588=CARTESIAN_POINT('Ctrl Pts',(7.16166667598849,-0.242625018493576,
-0.397500106126878));
#13589=CARTESIAN_POINT('Ctrl Pts',(7.06615616255898,0.0649458631171862,
-0.413200118862103));
#13590=CARTESIAN_POINT('Ctrl Pts',(7.27000662090844,0.314279166253809,-0.428900131597329));
#13591=CARTESIAN_POINT('Ctrl Pts',(7.59042338938741,0.281795325880159,-0.444600144332553));
#13592=CARTESIAN_POINT('Ctrl Pts',(7.74008567777533,-0.00337708649496984,
-0.46030015706778));
#13593=CARTESIAN_POINT('Ctrl Pts',(7.58478987623982,-0.285521233283839,
-0.476000169803004));
#13594=CARTESIAN_POINT('Ctrl Pts',(7.26379121994478,-0.311635750473927,
-0.491700182538231));
#13595=CARTESIAN_POINT('Ctrl Pts',(7.06493228333412,-0.0583035016171516,
-0.507400195273454));
#13596=CARTESIAN_POINT('Ctrl Pts',(7.16653178299239,0.247310058698613,-0.523100208008682));
#13597=CARTESIAN_POINT('Ctrl Pts',(7.47748447214868,0.331158312315696,-0.538800220743906));
#13598=CARTESIAN_POINT('Ctrl Pts',(7.71895609275597,0.118053739323133,-0.554500233479132));
#13599=CARTESIAN_POINT('Ctrl Pts',(7.67441672308789,-0.200910772496147,
-0.570200246214356));
#13600=CARTESIAN_POINT('Ctrl Pts',(7.3838052491755,-0.339716630418571,-0.585900258949582));
#13601=CARTESIAN_POINT('Ctrl Pts',(7.10771575565814,-0.173895400874276,
-0.601600271684807));
#13602=CARTESIAN_POINT('Ctrl Pts',(7.09372036429638,0.147859652419619,-0.617300284420033));
#13603=CARTESIAN_POINT('Ctrl Pts',(7.35436882789558,0.337027235324834,-0.633000297155258));
#13604=CARTESIAN_POINT('Ctrl Pts',(7.65593526721943,0.223979871280845,-0.648700309890484));
#13605=CARTESIAN_POINT('Ctrl Pts',(7.72800196410744,-0.0899136189806033,
-0.664400322625708));
#13606=CARTESIAN_POINT('Ctrl Pts',(7.5059464213128,-0.323178229874143,-0.680100335360935));
#13607=CARTESIAN_POINT('Ctrl Pts',(7.18888716507469,-0.266650813009551,
-0.695800348096159));
#13608=CARTESIAN_POINT('Ctrl Pts',(7.06113590454605,0.028995013794699,-0.711500360831385));
#13609=CARTESIAN_POINT('Ctrl Pts',(7.23724512814298,0.298620426571841,-0.72720037356661));
#13610=CARTESIAN_POINT('Ctrl Pts',(7.55930264642725,0.300510998101608,-0.742900386301836));
#13611=CARTESIAN_POINT('Ctrl Pts',(7.73850300061676,0.0328478514182617,
-0.758600399037061));
#13612=CARTESIAN_POINT('Ctrl Pts',(7.61418249633623,-0.264103546960032,
-0.774300411772286));
#13613=CARTESIAN_POINT('Ctrl Pts',(7.29776664728478,-0.324568311795507,
-0.790000424507512));
#13614=CARTESIAN_POINT('Ctrl Pts',(7.07309304883756,-0.0932947148370394,
-0.805700437242737));
#13615=CARTESIAN_POINT('Ctrl Pts',(7.118765210101,0.115503807360185,-0.816167112399554));
#13616=CARTESIAN_POINT('Ctrl Pts',(7.18048028959809,0.187686343907877,-0.821400449977962));
#13617=CARTESIAN_POINT('Ctrl Pts',(7.3301933573839,-0.261113218593861,0.0214004499779621));
#13618=CARTESIAN_POINT('Ctrl Pts',(7.24433403108591,-0.2381593775803,0.0161671123995537));
#13619=CARTESIAN_POINT('Ctrl Pts',(7.09842813467957,-0.10134039678683,0.00570043724273678));
#13620=CARTESIAN_POINT('Ctrl Pts',(7.1491042573084,0.196120197771411,-0.00999957549248853));
#13621=CARTESIAN_POINT('Ctrl Pts',(7.42518225369131,0.317218429483757,-0.0256995882277139));
#13622=CARTESIAN_POINT('Ctrl Pts',(7.67847250355587,0.154105176418319,-0.0413996009629392));
#13623=CARTESIAN_POINT('Ctrl Pts',(7.68215607610427,-0.147314696178063,
-0.0570996136981647));
#13624=CARTESIAN_POINT('Ctrl Pts',(7.43277688577798,-0.316577092585917,
-0.0727996264333898));
#13625=CARTESIAN_POINT('Ctrl Pts',(7.15403148416523,-0.201991008738314,
-0.0884996391686153));
#13626=CARTESIAN_POINT('Ctrl Pts',(7.09583594822706,0.093736844773651,-0.104199651903841));
#13627=CARTESIAN_POINT('Ctrl Pts',(7.31039341402957,0.305402784331873,-0.119899664639066));
#13628=CARTESIAN_POINT('Ctrl Pts',(7.60529890194435,0.243214679937923,-0.135599677374291));
#13629=CARTESIAN_POINT('Ctrl Pts',(7.71611241359684,-0.0370681275469361,
-0.151299690109517));
#13630=CARTESIAN_POINT('Ctrl Pts',(7.54346413841113,-0.284110713751843,
-0.166999702844742));
#13631=CARTESIAN_POINT('Ctrl Pts',(7.24217056726241,-0.276388931451618,
-0.182699715579967));
#13632=CARTESIAN_POINT('Ctrl Pts',(7.0824039775304,-0.020826327520145,-0.198399728315193));
#13633=CARTESIAN_POINT('Ctrl Pts',(7.20742887977719,0.253411337384138,-0.214099741050418));
#13634=CARTESIAN_POINT('Ctrl Pts',(7.50513410748264,0.300412677844047,-0.229799753785643));
#13635=CARTESIAN_POINT('Ctrl Pts',(7.70856459494988,0.0780310618225991,
-0.245499766520869));
#13636=CARTESIAN_POINT('Ctrl Pts',(7.63530223870985,-0.214321742927024,
-0.261199779256094));
#13637=CARTESIAN_POINT('Ctrl Pts',(7.35104211317455,-0.314490191131576,
-0.276899791991319));
#13638=CARTESIAN_POINT('Ctrl Pts',(7.11068299168808,-0.132652264669645,
-0.292599804726545));
#13639=CARTESIAN_POINT('Ctrl Pts',(7.12975720849912,0.168136218544819,-0.30829981746177));
#13640=CARTESIAN_POINT('Ctrl Pts',(7.39116072836547,0.318155342350428,-0.323999830196996));
#13641=CARTESIAN_POINT('Ctrl Pts',(7.66049050824145,0.182881518035819,-0.339699842932221));
#13642=CARTESIAN_POINT('Ctrl Pts',(7.6962359501787,-0.11638391779237,-0.355399855667446));
#13643=CARTESIAN_POINT('Ctrl Pts',(7.4663437737136,-0.311286778098894,-0.371099868402672));
#13644=CARTESIAN_POINT('Ctrl Pts',(7.17696049884618,-0.227055798078962,
-0.386799881137897));
#13645=CARTESIAN_POINT('Ctrl Pts',(7.08757888442605,0.0607782943142372,
-0.402499893873122));
#13646=CARTESIAN_POINT('Ctrl Pts',(7.27834828156687,0.294111907157829,-0.418199906608348));
#13647=CARTESIAN_POINT('Ctrl Pts',(7.57820394169864,0.263712551203101,-0.433899919343573));
#13648=CARTESIAN_POINT('Ctrl Pts',(7.71826241770918,-0.00316037923070726,
-0.449599932078799));
#13649=CARTESIAN_POINT('Ctrl Pts',(7.57293193046229,-0.267199367543656,
-0.465299944814024));
#13650=CARTESIAN_POINT('Ctrl Pts',(7.27253172219081,-0.291638119074134,
-0.480999957549249));
#13651=CARTESIAN_POINT('Ctrl Pts',(7.08643354139474,-0.0545621724118729,
-0.496699970284474));
#13652=CARTESIAN_POINT('Ctrl Pts',(7.18151341247548,0.231440199775832,-0.5123999830197));
#13653=CARTESIAN_POINT('Ctrl Pts',(7.47251230220066,0.309907920296823,-0.528099995754925));
#13654=CARTESIAN_POINT('Ctrl Pts',(7.69848871580723,0.110478244018884,-0.543800008490151));
#13655=CARTESIAN_POINT('Ctrl Pts',(7.65680743253023,-0.188018350601305,
-0.559500021225375));
#13656=CARTESIAN_POINT('Ctrl Pts',(7.38484446453224,-0.31791705208021,-0.575200033960601));
#13657=CARTESIAN_POINT('Ctrl Pts',(7.1264716030647,-0.162736552367599,-0.590900046695826));
#13658=CARTESIAN_POINT('Ctrl Pts',(7.11337429440789,0.138371514991572,-0.606600059431052));
#13659=CARTESIAN_POINT('Ctrl Pts',(7.35729697512741,0.31540023517011,-0.622300072166276));
#13660=CARTESIAN_POINT('Ctrl Pts',(7.63951192962648,0.209607107886287,-0.638000084901503));
#13661=CARTESIAN_POINT('Ctrl Pts',(7.70695411460156,-0.0841438720646569,
-0.653700097636727));
#13662=CARTESIAN_POINT('Ctrl Pts',(7.49914785125683,-0.302439918856771,
-0.669400110371954));
#13663=CARTESIAN_POINT('Ctrl Pts',(7.20243425217937,-0.249539860036695,
-0.685100123107178));
#13664=CARTESIAN_POINT('Ctrl Pts',(7.08288077581068,0.0271344069887835,
-0.700800135842404));
#13665=CARTESIAN_POINT('Ctrl Pts',(7.24768909014338,0.279457987057277,-0.716500148577629));
#13666=CARTESIAN_POINT('Ctrl Pts',(7.54908021334818,0.281227240822539,-0.732200161312854));
#13667=CARTESIAN_POINT('Ctrl Pts',(7.71678130076761,0.0307400084511485,
-0.74790017404808));
#13668=CARTESIAN_POINT('Ctrl Pts',(7.6004384294007,-0.247156051765875,-0.763600186783306));
#13669=CARTESIAN_POINT('Ctrl Pts',(7.30432695014238,-0.303740799376059,
-0.77930019951853));
#13670=CARTESIAN_POINT('Ctrl Pts',(7.09407063148472,-0.0873080033765519,
-0.795000212253756));
#13671=CARTESIAN_POINT('Ctrl Pts',(7.13681201524657,0.108091940906003,-0.805466887410573));
#13672=CARTESIAN_POINT('Ctrl Pts',(7.19456684496579,0.175642532122687,-0.810700224988981));
#13673=CARTESIAN_POINT('Ctrl Pts',(7.33498000020249,-0.243208680203507,
0.0321006749669432));
#13674=CARTESIAN_POINT('Ctrl Pts',(7.25500804955002,-0.221828784507026,
0.0268673373885347));
#13675=CARTESIAN_POINT('Ctrl Pts',(7.11910692324936,-0.0943914838419598,
0.0164006622317178));
#13676=CARTESIAN_POINT('Ctrl Pts',(7.16630818318082,0.182672232061242,0.000700649496492524));
#13677=CARTESIAN_POINT('Ctrl Pts',(7.42345550607431,0.295466755710189,-0.0149993632387329));
#13678=CARTESIAN_POINT('Ctrl Pts',(7.65937763866384,0.143538181525481,-0.0306993759739581));
#13679=CARTESIAN_POINT('Ctrl Pts',(7.66280862857218,-0.137213324645103,
-0.0463993887091836));
#13680=CARTESIAN_POINT('Ctrl Pts',(7.43052937409362,-0.294869395295694,
-0.0620994014444088));
#13681=CARTESIAN_POINT('Ctrl Pts',(7.1708975499979,-0.18814048140792,-0.0777994141796343));
#13682=CARTESIAN_POINT('Ctrl Pts',(7.11669248307145,0.0873093075356722,
-0.0934994269148595));
#13683=CARTESIAN_POINT('Ctrl Pts',(7.31653773934246,0.284461309572235,-0.109199439650085));
#13684=CARTESIAN_POINT('Ctrl Pts',(7.59122155231358,0.22653744468535,-0.12489945238531));
#13685=CARTESIAN_POINT('Ctrl Pts',(7.69443657935378,-0.0345263653324579,
-0.140599465120536));
#13686=CARTESIAN_POINT('Ctrl Pts',(7.53362679969785,-0.264629236678892,
-0.156299477855761));
#13687=CARTESIAN_POINT('Ctrl Pts',(7.25299293448225,-0.257436937138601,
-0.171999490590986));
#13688=CARTESIAN_POINT('Ctrl Pts',(7.10418154286223,-0.0193982658439779,
-0.187699503326212));
#13689=CARTESIAN_POINT('Ctrl Pts',(7.220633485172,0.236034917135561,-0.203399516061437));
#13690=CARTESIAN_POINT('Ctrl Pts',(7.49792505972285,0.27981337478167,-0.219099528796662));
#13691=CARTESIAN_POINT('Ctrl Pts',(7.68740631477572,0.0726804704218018,
-0.234799541531887));
#13692=CARTESIAN_POINT('Ctrl Pts',(7.61916755970354,-0.199625696917599,
-0.250499554267113));
#13693=CARTESIAN_POINT('Ctrl Pts',(7.35439915641003,-0.29292559271397,-0.266199567002338));
#13694=CARTESIAN_POINT('Ctrl Pts',(7.13052146447854,-0.123556296345501,
-0.281899579737564));
#13695=CARTESIAN_POINT('Ctrl Pts',(7.14828776187822,0.156607114825152,-0.297599592472789));
#13696=CARTESIAN_POINT('Ctrl Pts',(7.39176683739043,0.296339424443684,-0.313299605208015));
#13697=CARTESIAN_POINT('Ctrl Pts',(7.64262866911187,0.170341328848187,-0.32899961794324));
#13698=CARTESIAN_POINT('Ctrl Pts',(7.67592304541218,-0.108403470324582,
-0.344699630678465));
#13699=CARTESIAN_POINT('Ctrl Pts',(7.46179457988185,-0.289941837774174,
-0.360399643413691));
#13700=CARTESIAN_POINT('Ctrl Pts',(7.19225432170386,-0.211486577664347,
-0.376099656148916));
#13701=CARTESIAN_POINT('Ctrl Pts',(7.10900160629311,0.0566107255112876,
-0.391799668884141));
#13702=CARTESIAN_POINT('Ctrl Pts',(7.28668994222529,0.273944648061849,-0.407499681619367));
#13703=CARTESIAN_POINT('Ctrl Pts',(7.56598449400986,0.245629776526043,-0.423199694354592));
#13704=CARTESIAN_POINT('Ctrl Pts',(7.69643915764304,-0.00294367196644475,
-0.438899707089818));
#13705=CARTESIAN_POINT('Ctrl Pts',(7.56107398468478,-0.248877501803473,
-0.454599719825042));
#13706=CARTESIAN_POINT('Ctrl Pts',(7.28127222443683,-0.271640487674342,
-0.470299732560268));
#13707=CARTESIAN_POINT('Ctrl Pts',(7.10793479945536,-0.0508208432065944,
-0.485999745295493));
#13708=CARTESIAN_POINT('Ctrl Pts',(7.19649504195857,0.215570340853052,-0.501699758030719));
#13709=CARTESIAN_POINT('Ctrl Pts',(7.46754013225262,0.28865752827795,-0.517399770765943));
#13710=CARTESIAN_POINT('Ctrl Pts',(7.67802133885851,0.102902748714636,-0.53309978350117));
#13711=CARTESIAN_POINT('Ctrl Pts',(7.63919814197256,-0.175125928706463,
-0.548799796236394));
#13712=CARTESIAN_POINT('Ctrl Pts',(7.38588367988897,-0.29611747374185,-0.564499808971621));
#13713=CARTESIAN_POINT('Ctrl Pts',(7.14522745047125,-0.151577703860923,
-0.580199821706845));
#13714=CARTESIAN_POINT('Ctrl Pts',(7.13302822451941,0.128883377563526,-0.595899834442072));
#13715=CARTESIAN_POINT('Ctrl Pts',(7.36022512235921,0.293773235015386,-0.611599847177295));
#13716=CARTESIAN_POINT('Ctrl Pts',(7.62308859203355,0.195234344491729,-0.627299859912523));
#13717=CARTESIAN_POINT('Ctrl Pts',(7.68590626509567,-0.0783741251487107,
-0.642999872647746));
#13718=CARTESIAN_POINT('Ctrl Pts',(7.49234928120087,-0.281701607839398,
-0.658699885382973));
#13719=CARTESIAN_POINT('Ctrl Pts',(7.21598133928404,-0.232428907063839,
-0.674399898118197));
#13720=CARTESIAN_POINT('Ctrl Pts',(7.10462564707531,0.0252738001828684,
-0.690099910853423));
#13721=CARTESIAN_POINT('Ctrl Pts',(7.25813305214379,0.260295547542712,-0.705799923588648));
#13722=CARTESIAN_POINT('Ctrl Pts',(7.53885778026912,0.26194348354347,-0.721499936323873));
#13723=CARTESIAN_POINT('Ctrl Pts',(7.69505960091847,0.0286321654840352,
-0.737199949059099));
#13724=CARTESIAN_POINT('Ctrl Pts',(7.58669436246517,-0.230208556571718,
-0.752899961794324));
#13725=CARTESIAN_POINT('Ctrl Pts',(7.31088725299997,-0.282913286956612,
-0.768599974529549));
#13726=CARTESIAN_POINT('Ctrl Pts',(7.11504821413188,-0.0813212919160645,
-0.784299987264775));
#13727=CARTESIAN_POINT('Ctrl Pts',(7.15485882039215,0.10068007445182,-0.794766662421592));
#13728=CARTESIAN_POINT('Ctrl Pts',(7.2086534003335,0.163598720337497,-0.8));
#13729=CARTESIAN_POINT('Ctrl Pts',(7.14840641220525,0.000201202115797984,
-0.0887416697508019));
#13730=CARTESIAN_POINT('Ctrl Pts',(7.14821094317882,0.0253219375521799,
-0.0903275888054877));
#13731=CARTESIAN_POINT('Ctrl Pts',(7.15167836398483,0.0503900083073383,
-0.0919135078601736));
#13732=CARTESIAN_POINT('Ctrl Pts',(7.15903420360436,0.0742596763845007,
-0.0934994269148595));
#13733=CARTESIAN_POINT('Ctrl Pts',(7.18330756849512,0.15302664154786,-0.098732764493268));
#13734=CARTESIAN_POINT('Ctrl Pts',(7.24992265391879,0.218743975560048,-0.103966102071676));
#13735=CARTESIAN_POINT('Ctrl Pts',(7.32901083212581,0.241948665084994,-0.109199439650085));
#13736=CARTESIAN_POINT('Ctrl Pts',(7.40809901033283,0.26515335460994,-0.114432777228493));
#13737=CARTESIAN_POINT('Ctrl Pts',(7.49966028132321,0.245845399647645,-0.119666114806902));
#13738=CARTESIAN_POINT('Ctrl Pts',(7.5626434213251,0.19268078716353,-0.12489945238531));
#13739=CARTESIAN_POINT('Ctrl Pts',(7.62562656132698,0.139516174679414,-0.130132789963719));
#13740=CARTESIAN_POINT('Ctrl Pts',(7.66003157034038,0.0524949046734784,
-0.135366127542127));
#13741=CARTESIAN_POINT('Ctrl Pts',(7.65043244490443,-0.0293662088872284,
-0.140599465120536));
#13742=CARTESIAN_POINT('Ctrl Pts',(7.64083331946847,-0.111227322447936,
-0.145832802698944));
#13743=CARTESIAN_POINT('Ctrl Pts',(7.58723005958316,-0.187928279563414,
-0.151066140277352));
#13744=CARTESIAN_POINT('Ctrl Pts',(7.51365611877124,-0.225080041531105,
-0.156299477855761));
#13745=CARTESIAN_POINT('Ctrl Pts',(7.44008217795932,-0.262231803498795,
-0.161532815434169));
#13746=CARTESIAN_POINT('Ctrl Pts',(7.34653755622078,-0.259834370318698,
-0.166766153012578));
#13747=CARTESIAN_POINT('Ctrl Pts',(7.27496334674818,-0.218962541846212,
-0.171999490590986));
#13748=CARTESIAN_POINT('Ctrl Pts',(7.20338913727558,-0.178090713373726,
-0.177232828169395));
#13749=CARTESIAN_POINT('Ctrl Pts',(7.1537853400689,-0.0987444896088522,
-0.182466165747803));
#13750=CARTESIAN_POINT('Ctrl Pts',(7.14839209851719,-0.0164991805631585,
-0.187699503326212));
#13751=CARTESIAN_POINT('Ctrl Pts',(7.14803409528754,-0.0110397391529513,
-0.188046892134408));
#13752=CARTESIAN_POINT('Ctrl Pts',(7.14787089706648,-0.00556752350083036,
-0.188394280942605));
#13753=CARTESIAN_POINT('Ctrl Pts',(7.14789741337032,-9.36993803829212E-5,
-0.188741669750802));
#13754=CARTESIAN_POINT('Ctrl Pts',(7.32062007174671,-0.29692229537457,0.));
#13755=CARTESIAN_POINT('Ctrl Pts',(7.30380884409489,-0.290772673204267,
-8.6947763400151E-19));
#13756=CARTESIAN_POINT('Ctrl Pts',(7.28766915137083,-0.28307124049188,-5.12459696186606E-17));
#13757=CARTESIAN_POINT('Ctrl Pts',(7.27233060098557,-0.274000231430978,
-4.7271214720368E-17));
#13758=CARTESIAN_POINT('Ctrl Pts',(7.26235488632148,-0.26810073011996,-4.46861581322844E-17));
#13759=CARTESIAN_POINT('Ctrl Pts',(7.25271848455557,-0.261620831522484,
6.78577354371941E-18));
#13760=CARTESIAN_POINT('Ctrl Pts',(7.24346467188118,-0.254602044943363,
0.));
#13761=CARTESIAN_POINT('Ctrl Pts',(7.23605088975924,-0.24897887573852,-5.43648854284865E-18));
#13762=CARTESIAN_POINT('Ctrl Pts',(7.22888277290176,-0.243009665080752,
-2.33933283858092E-17));
#13763=CARTESIAN_POINT('Ctrl Pts',(7.22198623884541,-0.236713795342446,
-2.68882138776405E-17));
#13764=CARTESIAN_POINT('Ctrl Pts',(7.21845932875887,-0.233494066953934,
-2.86755097557909E-17));
#13765=CARTESIAN_POINT('Ctrl Pts',(7.21500977674086,-0.230194526695087,
3.15297170846717E-17));
#13766=CARTESIAN_POINT('Ctrl Pts',(7.21164329955151,-0.226821462504723,
3.20923843055709E-17));
#13767=CARTESIAN_POINT('Ctrl Pts',(7.19928407775938,-0.214438058102124,
3.41580834287554E-17));
#13768=CARTESIAN_POINT('Ctrl Pts',(7.18802725117541,-0.201052984273089,
5.78707788030305E-17));
#13769=CARTESIAN_POINT('Ctrl Pts',(7.17802303391905,-0.186814057526815,
8.32667268468867E-17));
#13770=CARTESIAN_POINT('Ctrl Pts',(7.17173408520147,-0.177863044388453,
9.92313756334403E-17));
#13771=CARTESIAN_POINT('Ctrl Pts',(7.16594094488153,-0.16857400717693,1.38900089258037E-17));
#13772=CARTESIAN_POINT('Ctrl Pts',(7.16069111243859,-0.15898037881098,6.93889390390723E-18));
#13773=CARTESIAN_POINT('Ctrl Pts',(7.15844635045079,-0.154878264597813,
3.96668499180442E-18));
#13774=CARTESIAN_POINT('Ctrl Pts',(7.15630103067416,-0.150720445577065,
4.11107772410956E-17));
#13775=CARTESIAN_POINT('Ctrl Pts',(7.15425938021799,-0.146509500605675,
4.16333634234434E-17));
#13776=CARTESIAN_POINT('Ctrl Pts',(7.15231306464394,-0.14249518573874,4.21315474404055E-17));
#13777=CARTESIAN_POINT('Ctrl Pts',(7.15046487911057,-0.138440587136871,
2.62921600658027E-17));
#13778=CARTESIAN_POINT('Ctrl Pts',(7.14871822055084,-0.134350184983525,
2.77555756156289E-17));
#13779=CARTESIAN_POINT('Ctrl Pts',(7.14246237732693,-0.119699975043201,
3.29969539034211E-17));
#13780=CARTESIAN_POINT('Ctrl Pts',(7.13750157461332,-0.1045828565666,7.60800602575303E-18));
#13781=CARTESIAN_POINT('Ctrl Pts',(7.13397523077828,-0.0891087999794577,
6.93889390390723E-18));
#13782=CARTESIAN_POINT('Ctrl Pts',(7.13145831420858,-0.0780642418629789,
6.30212507089961E-18));
#13783=CARTESIAN_POINT('Ctrl Pts',(7.12967323652615,-0.0668374439349906,
-2.87387945550391E-17));
#13784=CARTESIAN_POINT('Ctrl Pts',(7.12860812217214,-0.0554971960327241,
-4.16333634234434E-17));
#13785=CARTESIAN_POINT('Ctrl Pts',(7.12819480164633,-0.051096581950223,
-4.66371359898912E-17));
#13786=CARTESIAN_POINT('Ctrl Pts',(7.12789000373709,-0.046678913727008,
-5.89876804906217E-18));
#13787=CARTESIAN_POINT('Ctrl Pts',(7.1276934258001,-0.0422483700808671,
-1.04083408558608E-17));
#13788=CARTESIAN_POINT('Ctrl Pts',(7.12749092575898,-0.0376843519398602,
-1.50537689888955E-17));
#13789=CARTESIAN_POINT('Ctrl Pts',(7.12740372610782,-0.0331164650875104,
1.05127888270269E-18));
#13790=CARTESIAN_POINT('Ctrl Pts',(7.12743015237759,-0.0285512580926939,
3.46944695195361E-18));
#13791=CARTESIAN_POINT('Ctrl Pts',(7.12752823277688,-0.0116076134235948,
1.24444135990454E-17));
#13792=CARTESIAN_POINT('Ctrl Pts',(7.12918689135693,0.00531003058111619,
3.46252004887064E-17));
#13793=CARTESIAN_POINT('Ctrl Pts',(7.13235152789467,0.0219706470489435,
6.59194920871187E-17));
#13794=CARTESIAN_POINT('Ctrl Pts',(7.13400565404307,0.0306789966553936,
8.22767278743674E-17));
#13795=CARTESIAN_POINT('Ctrl Pts',(7.13607212944229,0.0393168936655102,
2.69042433030263E-17));
#13796=CARTESIAN_POINT('Ctrl Pts',(7.13854854623344,0.0478483384877713,
3.12250225675825E-17));
#13797=CARTESIAN_POINT('Ctrl Pts',(7.13999886673045,0.0528448032747235,
3.37554991629673E-17));
#13798=CARTESIAN_POINT('Ctrl Pts',(7.14159044784196,0.0578063658571401,
-8.00558532562018E-17));
#13799=CARTESIAN_POINT('Ctrl Pts',(7.1433214609991,0.0627200384290504,-5.89805981832114E-17));
#13800=CARTESIAN_POINT('Ctrl Pts',(7.1486420056914,0.0778229938366053,5.79755561356752E-18));
#13801=CARTESIAN_POINT('Ctrl Pts',(7.15525121899922,0.0924060906234471,
2.3609484991885E-18));
#13802=CARTESIAN_POINT('Ctrl Pts',(7.16312552449122,0.106254752470274,3.46944695195361E-17));
#13803=CARTESIAN_POINT('Ctrl Pts',(7.16719213282866,0.113406758927964,5.139280136525E-17));
#13804=CARTESIAN_POINT('Ctrl Pts',(7.171600828714,0.120367188403168,6.62813824659908E-17));
#13805=CARTESIAN_POINT('Ctrl Pts',(7.17633091943804,0.127074857793874,3.81639164714898E-17));
#13806=CARTESIAN_POINT('Ctrl Pts',(7.18357704399351,0.137350476321644,-4.90981565480567E-18));
#13807=CARTESIAN_POINT('Ctrl Pts',(7.19158181099666,0.14704579400106,-4.84899983333435E-17));
#13808=CARTESIAN_POINT('Ctrl Pts',(7.20034135671288,0.156042628024828,-4.16333634234434E-17));
#13809=CARTESIAN_POINT('Ctrl Pts',(7.20292789437632,0.15869923269453,-3.96087213913729E-17));
#13810=CARTESIAN_POINT('Ctrl Pts',(7.20558033511274,0.16129479584369,-2.29970654385668E-17));
#13811=CARTESIAN_POINT('Ctrl Pts',(7.20829596415884,0.163828130483802,-2.08166817117217E-17));
#13812=CARTESIAN_POINT('Origin',(0.,7.4,0.220842344717745));
#13813=CARTESIAN_POINT('Ctrl Pts',(-0.307720586104713,7.40015430359934,
-0.0291576552822542));
#13814=CARTESIAN_POINT('Ctrl Pts',(-0.307784268539838,7.41004356083263,
-0.0296715621794888));
#13815=CARTESIAN_POINT('Ctrl Pts',(-0.302900304337239,7.52057842373192,
-0.0354188066551319));
#13816=CARTESIAN_POINT('Ctrl Pts',(-0.169525066073537,7.71979475374946,
-0.0463993887091835));
#13817=CARTESIAN_POINT('Ctrl Pts',(0.173198823302611,7.71778284450742,-0.0620994014444088));
#13818=CARTESIAN_POINT('Ctrl Pts',(0.360608951848397,7.43085562333351,-0.0777994141796342));
#13819=CARTESIAN_POINT('Ctrl Pts',(0.224659911311872,7.11623824447284,-0.0934994269148595));
#13820=CARTESIAN_POINT('Ctrl Pts',(-0.112744986006889,7.05608347580814,
-0.109199439650085));
#13821=CARTESIAN_POINT('Ctrl Pts',(-0.291645285757027,7.24401442263803,
-0.12108551577255));
#13822=CARTESIAN_POINT('Ctrl Pts',(-0.307476655132152,7.37231065231555,
-0.127738254316606));
#13823=CARTESIAN_POINT('Ctrl Pts',(-0.307245619935592,7.39973933390828,
-0.129157655282254));
#13824=CARTESIAN_POINT('Ctrl Pts',(-0.30701976654778,7.39969382919393,-0.0208423447177451));
#13825=CARTESIAN_POINT('Ctrl Pts',(-0.306554866839469,7.46778804886732,
-0.0243615716353136));
#13826=CARTESIAN_POINT('Ctrl Pts',(-0.251028091428161,7.63805053601396,
-0.0331141361312906));
#13827=CARTESIAN_POINT('Ctrl Pts',(0.0286357548570192,7.76072194419717,
-0.047100038205676));
#13828=CARTESIAN_POINT('Ctrl Pts',(0.316662279094702,7.57523911945597,-0.0628000509409012));
#13829=CARTESIAN_POINT('Ctrl Pts',(0.320851004579023,7.23248257807725,-0.0785000636761267));
#13830=CARTESIAN_POINT('Ctrl Pts',(0.037271918951097,7.04000744673753,-0.094200076411352));
#13831=CARTESIAN_POINT('Ctrl Pts',(-0.247682056237118,7.15714576429466,
-0.108314170091891));
#13832=CARTESIAN_POINT('Ctrl Pts',(-0.306610241848052,7.32971128185523,
-0.117194926194023));
#13833=CARTESIAN_POINT('Ctrl Pts',(-0.307159081926734,7.40024563889874,
-0.120842344717745));
#13834=CARTESIAN_POINT('Ctrl Pts',(0.191346599666507,7.56359872033749,5.55111512312578E-17));
#13835=CARTESIAN_POINT('Ctrl Pts',(0.245141179607854,7.50068007445182,-0.00523333757840839));
#13836=CARTESIAN_POINT('Ctrl Pts',(0.284951890218192,7.31867881897261,-0.0157000127352253));
#13837=CARTESIAN_POINT('Ctrl Pts',(0.0891126990759621,7.11708667871666,
-0.0314000254704506));
#13838=CARTESIAN_POINT('Ctrl Pts',(-0.186694333111318,7.1697914830401,-0.047100038205676));
#13839=CARTESIAN_POINT('Ctrl Pts',(-0.295059597649767,7.42863214647761,
-0.0628000509409013));
#13840=CARTESIAN_POINT('Ctrl Pts',(-0.138857769266351,7.66194348220735,
-0.0785000636761267));
#13841=CARTESIAN_POINT('Ctrl Pts',(0.141866939210777,7.66029552986739,-0.094200076411352));
#13842=CARTESIAN_POINT('Ctrl Pts',(0.295374340744539,7.42527380242139,-0.109900089146577));
#13843=CARTESIAN_POINT('Ctrl Pts',(0.184018651936761,7.16757110150004,-0.125600101881803));
#13844=CARTESIAN_POINT('Ctrl Pts',(-0.0923492768089616,7.11829840583927,
-0.141300114617028));
#13845=CARTESIAN_POINT('Ctrl Pts',(-0.28590625237283,7.32162587781138,-0.157000127352254));
#13846=CARTESIAN_POINT('Ctrl Pts',(-0.223088581960643,7.59523433602638,
-0.172700140087479));
#13847=CARTESIAN_POINT('Ctrl Pts',(0.0397748758287548,7.69377322166141,
-0.188400152822704));
#13848=CARTESIAN_POINT('Ctrl Pts',(0.266971763504157,7.52888337186213,-0.204100165557929));
#13849=CARTESIAN_POINT('Ctrl Pts',(0.254772538082208,7.24842230290007,-0.219800178293155));
#13850=CARTESIAN_POINT('Ctrl Pts',(0.0141163194798009,7.10388253957977,
-0.23550019102838));
#13851=CARTESIAN_POINT('Ctrl Pts',(-0.239198131232389,7.22487407914503,
-0.251200203763606));
#13852=CARTESIAN_POINT('Ctrl Pts',(-0.278021326373094,7.50290274410036,
-0.266900216498831));
#13853=CARTESIAN_POINT('Ctrl Pts',(-0.0675401292199379,7.68865751531201,
-0.282600229234056));
#13854=CARTESIAN_POINT('Ctrl Pts',(0.20350494890297,7.61557033117447,-0.298300241969282));
#13855=CARTESIAN_POINT('Ctrl Pts',(0.292065187429107,7.34917915907462,-0.314000254704507));
#13856=CARTESIAN_POINT('Ctrl Pts',(0.118727770231601,7.12835952452443,-0.329700267439732));
#13857=CARTESIAN_POINT('Ctrl Pts',(-0.161073977451607,7.15112250937237,
-0.345400280174958));
#13858=CARTESIAN_POINT('Ctrl Pts',(-0.296439144331143,7.39705632816588,
-0.361100292910182));
#13859=CARTESIAN_POINT('Ctrl Pts',(-0.165984486556164,7.64562976549573,
-0.376800305645409));
#13860=CARTESIAN_POINT('Ctrl Pts',(0.113310052686424,7.67394463576013,-0.392500318380633));
#13861=CARTESIAN_POINT('Ctrl Pts',(0.29099838063931,7.4566107229691,-0.408200331115859));
#13862=CARTESIAN_POINT('Ctrl Pts',(0.207745668967121,7.18851343183269,-0.423900343851084));
#13863=CARTESIAN_POINT('Ctrl Pts',(-0.0617945771069258,7.11005817524592,
-0.43960035658631));
#13864=CARTESIAN_POINT('Ctrl Pts',(-0.275923033021548,7.29159653454344,
-0.455300369321535));
#13865=CARTESIAN_POINT('Ctrl Pts',(-0.242628658216455,7.57034132119874,
-0.471000382056761));
#13866=CARTESIAN_POINT('Ctrl Pts',(0.00823316223999692,7.69633941113648,
-0.486700394791986));
#13867=CARTESIAN_POINT('Ctrl Pts',(0.251712226818136,7.55660710779213,-0.502400407527211));
#13868=CARTESIAN_POINT('Ctrl Pts',(0.269478523420751,7.27644370920372,-0.518100420262436));
#13869=CARTESIAN_POINT('Ctrl Pts',(0.045600841541278,7.10707442043858,-0.533800432997662));
#13870=CARTESIAN_POINT('Ctrl Pts',(-0.219167549859846,7.20037431204982,
-0.549500445732887));
#13871=CARTESIAN_POINT('Ctrl Pts',(-0.287406301872761,7.4726804671522,-0.565200458468112));
#13872=CARTESIAN_POINT('Ctrl Pts',(-0.097925055319246,7.67981336222756,
-0.580900471203338));
#13873=CARTESIAN_POINT('Ctrl Pts',(0.179366506761887,7.63603490651475,-0.596600483938563));
#13874=CARTESIAN_POINT('Ctrl Pts',(0.295818443874949,7.38060173506806,-0.612300496673788));
#13875=CARTESIAN_POINT('Ctrl Pts',(0.147007058877446,7.14256307434387,-0.628000509409014));
#13876=CARTESIAN_POINT('Ctrl Pts',(-0.133626793626916,7.13537077535256,
-0.643700522144239));
#13877=CARTESIAN_POINT('Ctrl Pts',(-0.294436566257555,7.36547363593814,
-0.659400534879464));
#13878=CARTESIAN_POINT('Ctrl Pts',(-0.191221543505373,7.6265374350392,-0.67510054761469));
#13879=CARTESIAN_POINT('Ctrl Pts',(0.0834622565287631,7.68446129581186,
-0.690800560349915));
#13880=CARTESIAN_POINT('Ctrl Pts',(0.283307504842672,7.48730930545105,-0.706500573085141));
#13881=CARTESIAN_POINT('Ctrl Pts',(0.229102438696414,7.21185952364665,-0.722200585820366));
#13882=CARTESIAN_POINT('Ctrl Pts',(-0.0305293712063166,7.10513062416771,
-0.737900598555592));
#13883=CARTESIAN_POINT('Ctrl Pts',(-0.262808618747949,7.26278667022359,
-0.753600611290816));
#13884=CARTESIAN_POINT('Ctrl Pts',(-0.259377625204068,7.54353819533719,
-0.769300624026042));
#13885=CARTESIAN_POINT('Ctrl Pts',(-0.0234555043215238,7.69546670643878,
-0.785000636761267));
#13886=CARTESIAN_POINT('Ctrl Pts',(0.233691796768955,7.58267228749613,-0.800700649496493));
#13887=CARTESIAN_POINT('Ctrl Pts',(0.28089309993379,7.30560836566625,-0.816400662231718));
#13888=CARTESIAN_POINT('Ctrl Pts',(0.144991950449973,7.17817121549297,-0.826867337388535));
#13889=CARTESIAN_POINT('Ctrl Pts',(0.0650199997975051,7.15679131979649,
-0.832100674966943));
#13890=CARTESIAN_POINT('Ctrl Pts',(0.20543315503421,7.57564253212268,0.0107002249889811));
#13891=CARTESIAN_POINT('Ctrl Pts',(0.26318798475343,7.508091940906,0.00546688741057267));
#13892=CARTESIAN_POINT('Ctrl Pts',(0.305929480547396,7.31269211567552,-0.00499978774624422));
#13893=CARTESIAN_POINT('Ctrl Pts',(0.0956729984054867,7.09625916377015,
-0.0206998004814696));
#13894=CARTESIAN_POINT('Ctrl Pts',(-0.200438397885882,7.15284399076208,
-0.0363998132166949));
#13895=CARTESIAN_POINT('Ctrl Pts',(-0.316781297258277,7.43073998804551,
-0.0520998259519203));
#13896=CARTESIAN_POINT('Ctrl Pts',(-0.149080201535413,7.68122723938805,
-0.0677998386871456));
#13897=CARTESIAN_POINT('Ctrl Pts',(0.152310900574722,7.67945796808074,-0.083499851422371));
#13898=CARTESIAN_POINT('Ctrl Pts',(0.317119211112491,7.42713440939209,-0.0991998641575964));
#13899=CARTESIAN_POINT('Ctrl Pts',(0.197565738395132,7.15046014915765,-0.114899876892822));
#13900=CARTESIAN_POINT('Ctrl Pts',(-0.0991478465416041,7.09756009582889,
-0.130599889628047));
#13901=CARTESIAN_POINT('Ctrl Pts',(-0.306954100942084,7.31585613111335,
-0.146299902363272));
#13902=CARTESIAN_POINT('Ctrl Pts',(-0.239511918812032,7.60960709879773,
-0.161999915098498));
#13903=CARTESIAN_POINT('Ctrl Pts',(0.0427030229271706,7.71540022083304,
-0.177699927833723));
#13904=CARTESIAN_POINT('Ctrl Pts',(0.28662569273399,7.53837150887044,-0.193399940568948));
#13905=CARTESIAN_POINT('Ctrl Pts',(0.273528384646088,7.23726345489113,-0.209099953304174));
#13906=CARTESIAN_POINT('Ctrl Pts',(0.0151555347900653,7.08208296222211,
-0.224799966039399));
#13907=CARTESIAN_POINT('Ctrl Pts',(-0.256807420999381,7.21198165782819,
-0.240499978774624));
#13908=CARTESIAN_POINT('Ctrl Pts',(-0.298488702402679,7.51047823906491,
-0.25619999150985));
#13909=CARTESIAN_POINT('Ctrl Pts',(-0.0725122989447028,7.70990790637636,
-0.271900004245075));
#13910=CARTESIAN_POINT('Ctrl Pts',(0.218486577713304,7.63144018938473,-0.287600016980301));
#13911=CARTESIAN_POINT('Ctrl Pts',(0.313566444524186,7.34543783003727,-0.303300029715526));
#13912=CARTESIAN_POINT('Ctrl Pts',(0.127468272085129,7.10836189402269,-0.319000042450751));
#13913=CARTESIAN_POINT('Ctrl Pts',(-0.172931922696637,7.13280064445492,
-0.334700055185977));
#13914=CARTESIAN_POINT('Ctrl Pts',(-0.318262403417289,7.39683962091136,
-0.350400067921201));
#13915=CARTESIAN_POINT('Ctrl Pts',(-0.178203933696214,7.66371253936076,
-0.366100080656428));
#13916=CARTESIAN_POINT('Ctrl Pts',(0.121651712970258,7.69411189395048,-0.381800093391652));
#13917=CARTESIAN_POINT('Ctrl Pts',(0.312421101544368,7.4607782915849,-0.397500106126878));
#13918=CARTESIAN_POINT('Ctrl Pts',(0.223039491138021,7.17294421211722,-0.413200118862104));
#13919=CARTESIAN_POINT('Ctrl Pts',(-0.0663437707343935,7.08871323587971,
-0.428900131597328));
#13920=CARTESIAN_POINT('Ctrl Pts',(-0.296235936875898,7.28361608743404,
-0.444600144332554));
#13921=CARTESIAN_POINT('Ctrl Pts',(-0.260490496543942,7.58288150982323,
-0.460300157067779));
#13922=CARTESIAN_POINT('Ctrl Pts',(0.0088392712377377,7.71815532806358,
-0.476000169803004));
#13923=CARTESIAN_POINT('Ctrl Pts',(0.270242779365091,7.56813621099405,-0.49170018253823));
#13924=CARTESIAN_POINT('Ctrl Pts',(0.289316995320379,7.2673477412881,-0.507400195273455));
#13925=CARTESIAN_POINT('Ctrl Pts',(0.0489578846259453,7.08550982298924,
-0.523100208008681));
#13926=CARTESIAN_POINT('Ctrl Pts',(-0.235302228141484,7.18567826670055,
-0.538800220743906));
#13927=CARTESIAN_POINT('Ctrl Pts',(-0.308564581097026,7.4780310583123,-0.554500233479132));
#13928=CARTESIAN_POINT('Ctrl Pts',(-0.105134102754863,7.70041266436573,
-0.570200246214357));
#13929=CARTESIAN_POINT('Ctrl Pts',(0.192571111562895,7.65341132598145,-0.585900258949582));
#13930=CARTESIAN_POINT('Ctrl Pts',(0.31759600823039,7.37917367345902,-0.601600271684807));
#13931=CARTESIAN_POINT('Ctrl Pts',(0.157829425608444,7.12361108087618,-0.617300284420032));
#13932=CARTESIAN_POINT('Ctrl Pts',(-0.14346413189326,7.11588929916533,-0.633000297155258));
#13933=CARTESIAN_POINT('Ctrl Pts',(-0.316112399536496,7.36293187381722,
-0.648700309890483));
#13934=CARTESIAN_POINT('Ctrl Pts',(-0.205298892487695,7.64321466958163,
-0.664400322625709));
#13935=CARTESIAN_POINT('Ctrl Pts',(0.0896065815376993,7.70540276955849,
-0.680100335360935));
#13936=CARTESIAN_POINT('Ctrl Pts',(0.304164038797326,7.49373684253556,-0.695800348096159));
#13937=CARTESIAN_POINT('Ctrl Pts',(0.245968503696772,7.19800899668837,-0.711500360831385));
#13938=CARTESIAN_POINT('Ctrl Pts',(-0.0327768826781086,7.08342292831035,
-0.72720037356661));
#13939=CARTESIAN_POINT('Ctrl Pts',(-0.282156065556801,7.25268529831287,
-0.742900386301836));
#13940=CARTESIAN_POINT('Ctrl Pts',(-0.278472489105221,7.55410519124682,
-0.75860039903706));
#13941=CARTESIAN_POINT('Ctrl Pts',(-0.025182251809477,7.71721837658509,
-0.774300411772287));
#13942=CARTESIAN_POINT('Ctrl Pts',(0.250895721165319,7.5961202572873,-0.790000424507511));
#13943=CARTESIAN_POINT('Ctrl Pts',(0.30157189021028,7.29865944164248,-0.805700437242738));
#13944=CARTESIAN_POINT('Ctrl Pts',(0.155665968914083,7.1618406224197,-0.816167112399554));
#13945=CARTESIAN_POINT('Ctrl Pts',(0.0698066426160968,7.13888678140614,
-0.821400449977962));
#13946=CARTESIAN_POINT('Ctrl Pts',(0.219519710401913,7.58768634390787,0.0214004499779622));
#13947=CARTESIAN_POINT('Ctrl Pts',(0.281234789899007,7.51550380736018,0.0161671123995537));
#13948=CARTESIAN_POINT('Ctrl Pts',(0.3269070708766,7.30670541237844,0.00570043724273685));
#13949=CARTESIAN_POINT('Ctrl Pts',(0.102233297735012,7.07543164882364,-0.00999957549248853));
#13950=CARTESIAN_POINT('Ctrl Pts',(-0.214182462660446,7.13589649848406,
-0.0256995882277138));
#13951=CARTESIAN_POINT('Ctrl Pts',(-0.338502996866787,7.43284782961341,
-0.0413996009629392));
#13952=CARTESIAN_POINT('Ctrl Pts',(-0.159302633804475,7.70051099656875,
-0.0570996136981645));
#13953=CARTESIAN_POINT('Ctrl Pts',(0.162754861938666,7.69862040629408,-0.0727996264333899));
#13954=CARTESIAN_POINT('Ctrl Pts',(0.338864081480445,7.4289950163628,-0.0884996391686152));
#13955=CARTESIAN_POINT('Ctrl Pts',(0.211112824853502,7.13334919681524,-0.104199651903841));
#13956=CARTESIAN_POINT('Ctrl Pts',(-0.105946416274246,7.07682178581851,
-0.119899664639066));
#13957=CARTESIAN_POINT('Ctrl Pts',(-0.328001949511339,7.31008638441533,
-0.135599677374291));
#13958=CARTESIAN_POINT('Ctrl Pts',(-0.255935255663421,7.62397986156908,
-0.151299690109517));
#13959=CARTESIAN_POINT('Ctrl Pts',(0.0456311700255866,7.73702722000468,
-0.166999702844742));
#13960=CARTESIAN_POINT('Ctrl Pts',(0.306279621963823,7.54785964587876,-0.182699715579967));
#13961=CARTESIAN_POINT('Ctrl Pts',(0.292284231209968,7.22610460688219,-0.198399728315193));
#13962=CARTESIAN_POINT('Ctrl Pts',(0.0161947501003294,7.06028338486446,
-0.214099741050418));
#13963=CARTESIAN_POINT('Ctrl Pts',(-0.274416710766373,7.19908923651137,
-0.229799753785644));
#13964=CARTESIAN_POINT('Ctrl Pts',(-0.318956078432264,7.51805373402946,
-0.245499766520868));
#13965=CARTESIAN_POINT('Ctrl Pts',(-0.0774844686694676,7.73115829744071,
-0.261199779256094));
#13966=CARTESIAN_POINT('Ctrl Pts',(0.233468206523639,7.64731004759499,-0.276899791991319));
#13967=CARTESIAN_POINT('Ctrl Pts',(0.335067701619265,7.34169650099994,-0.292599804726545));
#13968=CARTESIAN_POINT('Ctrl Pts',(0.136208773938657,7.08836426352094,-0.30829981746177));
#13969=CARTESIAN_POINT('Ctrl Pts',(-0.184789867941668,7.11447877953749,
-0.323999830196996));
#13970=CARTESIAN_POINT('Ctrl Pts',(-0.340085662503434,7.39662291365683,
-0.33969984293222));
#13971=CARTESIAN_POINT('Ctrl Pts',(-0.190423380836264,7.68179531322579,
-0.355399855667447));
#13972=CARTESIAN_POINT('Ctrl Pts',(0.129993373254091,7.71427915214083,-0.371099868402671));
#13973=CARTESIAN_POINT('Ctrl Pts',(0.333843822449427,7.4649458602007,-0.386799881137897));
#13974=CARTESIAN_POINT('Ctrl Pts',(0.23833331330892,7.15737499240176,-0.402499893873122));
#13975=CARTESIAN_POINT('Ctrl Pts',(-0.0708929643618612,7.06736829651351,
-0.418199906608347));
#13976=CARTESIAN_POINT('Ctrl Pts',(-0.316548840730248,7.27563564032462,
-0.433899919343573));
#13977=CARTESIAN_POINT('Ctrl Pts',(-0.27835233487143,7.59542169844773,-0.449599932078798));
#13978=CARTESIAN_POINT('Ctrl Pts',(0.00944538023547856,7.73997124499067,
-0.465299944814023));
#13979=CARTESIAN_POINT('Ctrl Pts',(0.288773331912047,7.57966531419596,-0.48099995754925));
#13980=CARTESIAN_POINT('Ctrl Pts',(0.309155467220007,7.25825177337248,-0.496699970284473));
#13981=CARTESIAN_POINT('Ctrl Pts',(0.0523149277106133,7.0639452255399,-0.512399983019701));
#13982=CARTESIAN_POINT('Ctrl Pts',(-0.251436906423123,7.17098222135129,
-0.528099995754924));
#13983=CARTESIAN_POINT('Ctrl Pts',(-0.329722860321289,7.48338164947239,
-0.543800008490151));
#13984=CARTESIAN_POINT('Ctrl Pts',(-0.112343150190481,7.72101196650389,
-0.559500021225375));
#13985=CARTESIAN_POINT('Ctrl Pts',(0.205775716363902,7.67078774544814,-0.575200033960602));
#13986=CARTESIAN_POINT('Ctrl Pts',(0.339373572585832,7.37774561185,-0.590900046695826));
#13987=CARTESIAN_POINT('Ctrl Pts',(0.168651792339442,7.10465908740848,-0.606600059431052));
#13988=CARTESIAN_POINT('Ctrl Pts',(-0.153301470159604,7.09640782297811,
-0.622300072166277));
#13989=CARTESIAN_POINT('Ctrl Pts',(-0.337788232815437,7.36039011169628,
-0.638000084901502));
#13990=CARTESIAN_POINT('Ctrl Pts',(-0.219376241470017,7.65989190412407,
-0.653700097636728));
#13991=CARTESIAN_POINT('Ctrl Pts',(0.0957509065466354,7.72634424330511,
-0.669400110371953));
#13992=CARTESIAN_POINT('Ctrl Pts',(0.325020572751981,7.50016437962007,-0.685100123107179));
#13993=CARTESIAN_POINT('Ctrl Pts',(0.26283456869713,7.18415846973008,-0.700800135842403));
#13994=CARTESIAN_POINT('Ctrl Pts',(-0.0350243941499009,7.06171523245298,
-0.71650014857763));
#13995=CARTESIAN_POINT('Ctrl Pts',(-0.301503512365654,7.24258392640215,
-0.732200161312854));
#13996=CARTESIAN_POINT('Ctrl Pts',(-0.297567353006375,7.56467218715645,
-0.74790017404808));
#13997=CARTESIAN_POINT('Ctrl Pts',(-0.0269089992974306,7.73897004673138,
-0.763600186783305));
#13998=CARTESIAN_POINT('Ctrl Pts',(0.268099645561683,7.60956822707849,-0.779300199518531));
#13999=CARTESIAN_POINT('Ctrl Pts',(0.32225068048677,7.2917105176187,-0.795000212253756));
#14000=CARTESIAN_POINT('Ctrl Pts',(0.166339987378192,7.14551002934642,-0.805466887410573));
#14001=CARTESIAN_POINT('Ctrl Pts',(0.0745932854346885,7.12098224301578,
-0.810700224988981));
#14002=CARTESIAN_POINT('Ctrl Pts',(0.233606265769617,7.59973015569306,0.0321006749669432));
#14003=CARTESIAN_POINT('Ctrl Pts',(0.299281595044583,7.52291567381436,0.0268673373885348));
#14004=CARTESIAN_POINT('Ctrl Pts',(0.347884661205805,7.30071870908135,0.0164006622317179));
#14005=CARTESIAN_POINT('Ctrl Pts',(0.108793597064536,7.05460413387712,0.000700649496492544));
#14006=CARTESIAN_POINT('Ctrl Pts',(-0.227926527435009,7.11894900620605,
-0.0149993632387328));
#14007=CARTESIAN_POINT('Ctrl Pts',(-0.360224696475297,7.43495567118131,
-0.0306993759739581));
#14008=CARTESIAN_POINT('Ctrl Pts',(-0.169525066073537,7.71979475374946,
-0.0463993887091835));
#14009=CARTESIAN_POINT('Ctrl Pts',(0.173198823302611,7.71778284450742,-0.0620994014444088));
#14010=CARTESIAN_POINT('Ctrl Pts',(0.360608951848397,7.43085562333351,-0.0777994141796342));
#14011=CARTESIAN_POINT('Ctrl Pts',(0.224659911311872,7.11623824447284,-0.0934994269148595));
#14012=CARTESIAN_POINT('Ctrl Pts',(-0.112744986006889,7.05608347580814,
-0.109199439650085));
#14013=CARTESIAN_POINT('Ctrl Pts',(-0.349049798080593,7.30431663771729,
-0.12489945238531));
#14014=CARTESIAN_POINT('Ctrl Pts',(-0.272358592514811,7.63835262434044,
-0.140599465120536));
#14015=CARTESIAN_POINT('Ctrl Pts',(0.0485593171240025,7.7586542191763,-0.156299477855761));
#14016=CARTESIAN_POINT('Ctrl Pts',(0.325933551193656,7.55734778288709,-0.171999490590986));
#14017=CARTESIAN_POINT('Ctrl Pts',(0.311040077773849,7.21494575887322,-0.187699503326212));
#14018=CARTESIAN_POINT('Ctrl Pts',(0.0172339654105937,7.03848380750682,
-0.203399516061437));
#14019=CARTESIAN_POINT('Ctrl Pts',(-0.292026000533365,7.18619681519453,
-0.219099528796662));
#14020=CARTESIAN_POINT('Ctrl Pts',(-0.339423454461849,7.52562922899402,
-0.234799541531887));
#14021=CARTESIAN_POINT('Ctrl Pts',(-0.0824566383942325,7.75240868850505,
-0.250499554267113));
#14022=CARTESIAN_POINT('Ctrl Pts',(0.248449835333973,7.66317990580525,-0.266199567002338));
#14023=CARTESIAN_POINT('Ctrl Pts',(0.356568958714344,7.3379551719626,-0.281899579737564));
#14024=CARTESIAN_POINT('Ctrl Pts',(0.144949275792185,7.0683666330192,-0.297599592472788));
#14025=CARTESIAN_POINT('Ctrl Pts',(-0.196647813186698,7.09615691462004,
-0.313299605208015));
#14026=CARTESIAN_POINT('Ctrl Pts',(-0.36190892158958,7.39640620640232,-0.328999617943239));
#14027=CARTESIAN_POINT('Ctrl Pts',(-0.202642827976314,7.69987808709081,
-0.344699630678466));
#14028=CARTESIAN_POINT('Ctrl Pts',(0.138335033537924,7.73444641033119,-0.36039964341369));
#14029=CARTESIAN_POINT('Ctrl Pts',(0.355266543354486,7.46911342881649,-0.376099656148916));
#14030=CARTESIAN_POINT('Ctrl Pts',(0.25362713547982,7.1418057726863,-0.391799668884141));
#14031=CARTESIAN_POINT('Ctrl Pts',(-0.0754421579893288,7.0460233571473,
-0.407499681619367));
#14032=CARTESIAN_POINT('Ctrl Pts',(-0.336861744584598,7.26765519321521,
-0.423199694354592));
#14033=CARTESIAN_POINT('Ctrl Pts',(-0.296214173198918,7.60796188707222,
-0.438899707089817));
#14034=CARTESIAN_POINT('Ctrl Pts',(0.0100514892332193,7.76178716191776,
-0.454599719825043));
#14035=CARTESIAN_POINT('Ctrl Pts',(0.307303884459003,7.59119441739787,-0.470299732560268));
#14036=CARTESIAN_POINT('Ctrl Pts',(0.328993939119635,7.24915580545685,-0.485999745295493));
#14037=CARTESIAN_POINT('Ctrl Pts',(0.0556719707952805,7.04238062809055,
-0.501699758030718));
#14038=CARTESIAN_POINT('Ctrl Pts',(-0.267571584704761,7.15628617600203,
-0.517399770765944));
#14039=CARTESIAN_POINT('Ctrl Pts',(-0.350881139545554,7.48873224063248,
-0.533099783501169));
#14040=CARTESIAN_POINT('Ctrl Pts',(-0.119552197626099,7.74161126864207,
-0.548799796236395));
#14041=CARTESIAN_POINT('Ctrl Pts',(0.21898032116491,7.68816416491483,-0.56449980897162));
#14042=CARTESIAN_POINT('Ctrl Pts',(0.361151136941273,7.37631755024098,-0.580199821706846));
#14043=CARTESIAN_POINT('Ctrl Pts',(0.17947415907044,7.08570709394078,-0.59589983444207));
#14044=CARTESIAN_POINT('Ctrl Pts',(-0.163138808425949,7.0769263467909,-0.611599847177296));
#14045=CARTESIAN_POINT('Ctrl Pts',(-0.359464066094377,7.35784834957533,
-0.627299859912521));
#14046=CARTESIAN_POINT('Ctrl Pts',(-0.23345359045234,7.67656913866652,-0.642999872647747));
#14047=CARTESIAN_POINT('Ctrl Pts',(0.101895231555572,7.74728571705174,-0.658699885382972));
#14048=CARTESIAN_POINT('Ctrl Pts',(0.345877106706635,7.50659191670458,-0.674399898118198));
#14049=CARTESIAN_POINT('Ctrl Pts',(0.279700633697489,7.17030794277179,-0.690099910853422));
#14050=CARTESIAN_POINT('Ctrl Pts',(-0.0372719056216933,7.04000753659561,
-0.705799923588649));
#14051=CARTESIAN_POINT('Ctrl Pts',(-0.320850959174506,7.23248255449144,
-0.721499936323873));
#14052=CARTESIAN_POINT('Ctrl Pts',(-0.316662216907529,7.57523918306608,
-0.737199949059099));
#14053=CARTESIAN_POINT('Ctrl Pts',(-0.0286357467853838,7.76072171687769,
-0.752899961794324));
#14054=CARTESIAN_POINT('Ctrl Pts',(0.285303569958047,7.62301619686966,-0.76859997452955));
#14055=CARTESIAN_POINT('Ctrl Pts',(0.342929470763259,7.28476159359493,-0.784299987264775));
#14056=CARTESIAN_POINT('Ctrl Pts',(0.177014005842301,7.12917943627315,-0.794766662421592));
#14057=CARTESIAN_POINT('Ctrl Pts',(0.0793799282532802,7.10307770462543,
-0.8));
#14058=CARTESIAN_POINT('Ctrl Pts',(0.191346599666507,7.56359872033749,5.55111512312578E-17));
#14059=CARTESIAN_POINT('Ctrl Pts',(0.202509826020292,7.55310802872158,6.16763785454856E-17));
#14060=CARTESIAN_POINT('Ctrl Pts',(0.212570047977324,7.54158673074805,8.87136279239473E-17));
#14061=CARTESIAN_POINT('Ctrl Pts',(0.221522330388386,7.52925232800775,7.37257477290143E-17));
#14062=CARTESIAN_POINT('Ctrl Pts',(0.229528850137145,7.51822099157367,6.03212601064505E-17));
#14063=CARTESIAN_POINT('Ctrl Pts',(0.236649183304017,7.50653794848467,5.97068861804943E-17));
#14064=CARTESIAN_POINT('Ctrl Pts',(0.242860378108039,7.49433128865099,4.9439619065339E-17));
#14065=CARTESIAN_POINT('Ctrl Pts',(0.244940778165198,7.49024274584772,4.60006634751179E-17));
#14066=CARTESIAN_POINT('Ctrl Pts',(0.246919664339563,7.48609381169182,9.01432872076705E-17));
#14067=CARTESIAN_POINT('Ctrl Pts',(0.248793550657622,7.48189349080544,8.67361737988404E-17));
#14068=CARTESIAN_POINT('Ctrl Pts',(0.255493781437556,7.46687490669106,7.4553766620469E-17));
#14069=CARTESIAN_POINT('Ctrl Pts',(0.26081112509558,7.45130222640364,9.16174316001598E-17));
#14070=CARTESIAN_POINT('Ctrl Pts',(0.264722870572182,7.43540153025387,7.11236625150491E-17));
#14071=CARTESIAN_POINT('Ctrl Pts',(0.267427619696875,7.42440710481122,5.69533888287461E-17));
#14072=CARTESIAN_POINT('Ctrl Pts',(0.269459688552597,7.41325478922081,4.6972572244459E-17));
#14073=CARTESIAN_POINT('Ctrl Pts',(0.27079974443572,7.40201099931185,3.29597460435593E-17));
#14074=CARTESIAN_POINT('Ctrl Pts',(0.271554695341832,7.39567655498994,2.50653022589546E-17));
#14075=CARTESIAN_POINT('Ctrl Pts',(0.27208982123207,7.38931298403657,1.01541313543095E-16));
#14076=CARTESIAN_POINT('Ctrl Pts',(0.272400071186847,7.38293173498231,1.14491749414469E-16));
#14077=CARTESIAN_POINT('Ctrl Pts',(0.272610339929182,7.37860690852382,1.23268775233286E-16));
#14078=CARTESIAN_POINT('Ctrl Pts',(0.272716817601982,7.37428302936599,7.71694655557428E-17));
#14079=CARTESIAN_POINT('Ctrl Pts',(0.272719010540345,7.36996555954461,7.63278329429795E-17));
#14080=CARTESIAN_POINT('Ctrl Pts',(0.27272701832973,7.35419977716697,7.3254505933478E-17));
#14081=CARTESIAN_POINT('Ctrl Pts',(0.271347675050127,7.33851331166065,5.02512909736644E-18));
#14082=CARTESIAN_POINT('Ctrl Pts',(0.268538219226134,7.32308196703815,-6.93889390390723E-18));
#14083=CARTESIAN_POINT('Ctrl Pts',(0.266219736693056,7.31034736460601,-1.6812114944404E-17));
#14084=CARTESIAN_POINT('Ctrl Pts',(0.262926834287202,7.29778580690884,6.55929388800579E-17));
#14085=CARTESIAN_POINT('Ctrl Pts',(0.25873271504902,7.2854645892766,5.89805981832114E-17));
#14086=CARTESIAN_POINT('Ctrl Pts',(0.256787879633764,7.279751175077,5.59144206058319E-17));
#14087=CARTESIAN_POINT('Ctrl Pts',(0.254646960594001,7.27408549701033,9.6934502491867E-17));
#14088=CARTESIAN_POINT('Ctrl Pts',(0.252327976440821,7.26850105163772,9.71445146547012E-17));
#14089=CARTESIAN_POINT('Ctrl Pts',(0.245813541691288,7.25281336142979,9.77344757932954E-17));
#14090=CARTESIAN_POINT('Ctrl Pts',(0.237886985486038,7.23772772890658,5.31942244547902E-17));
#14091=CARTESIAN_POINT('Ctrl Pts',(0.228725953446014,7.22338664087012,2.42861286636753E-17));
#14092=CARTESIAN_POINT('Ctrl Pts',(0.223374596687987,7.21500938838961,7.3996541815834E-18));
#14093=CARTESIAN_POINT('Ctrl Pts',(0.217600970276322,7.20688618729852,1.2717535362053E-16));
#14094=CARTESIAN_POINT('Ctrl Pts',(0.211432869234838,7.19904719786575,1.35308431126191E-16));
#14095=CARTESIAN_POINT('Ctrl Pts',(0.207420256499723,7.19394760098548,1.40599344837786E-16));
#14096=CARTESIAN_POINT('Ctrl Pts',(0.203240590920077,7.18896831877402,8.31322120915072E-17));
#14097=CARTESIAN_POINT('Ctrl Pts',(0.198900453572221,7.18411827831884,8.32667268468867E-17));
#14098=CARTESIAN_POINT('Ctrl Pts',(0.195670954353016,7.18050935984282,8.33668193699228E-17));
#14099=CARTESIAN_POINT('Ctrl Pts',(0.192355312382397,7.17697524795826,4.32686351463275E-17));
#14100=CARTESIAN_POINT('Ctrl Pts',(0.188962380915405,7.17352497672425,3.81639164714898E-17));
#14101=CARTESIAN_POINT('Ctrl Pts',(0.17975235020419,7.16415929859711,2.43072806317295E-17));
#14102=CARTESIAN_POINT('Ctrl Pts',(0.169962167438026,7.15539778977274,5.97745424410255E-17));
#14103=CARTESIAN_POINT('Ctrl Pts',(0.159655188940229,7.14730762660204,4.5102810375397E-17));
#14104=CARTESIAN_POINT('Ctrl Pts',(0.154921336855726,7.14359192701095,3.83642875932839E-17));
#14105=CARTESIAN_POINT('Ctrl Pts',(0.150078290017851,7.14001794308044,6.33235573476612E-17));
#14106=CARTESIAN_POINT('Ctrl Pts',(0.145131356394006,7.13659282212682,6.24500451351651E-17));
#14107=CARTESIAN_POINT('Ctrl Pts',(0.139972270742195,7.13302081293665,6.15390718606404E-17));
#14108=CARTESIAN_POINT('Ctrl Pts',(0.134706655684311,7.12961533000732,6.44888900829108E-17));
#14109=CARTESIAN_POINT('Ctrl Pts',(0.129346139120924,7.12638655487346,6.24500451351651E-17));
#14110=CARTESIAN_POINT('Ctrl Pts',(0.117404508126543,7.11919380754091,5.79081071087007E-17));
#14111=CARTESIAN_POINT('Ctrl Pts',(0.104985462890608,7.11287199690184,1.81867207105765E-17));
#14112=CARTESIAN_POINT('Ctrl Pts',(0.0921567668402144,7.10750685206111,
-6.93889390390723E-18));
#14113=CARTESIAN_POINT('Ctrl Pts',(0.0880066571319542,7.10577121660741,
-2.89761322741409E-17));
#14114=CARTESIAN_POINT('Ctrl Pts',(0.0838135816987372,7.10413581036214,
-6.25245253825226E-20));
#14115=CARTESIAN_POINT('Ctrl Pts',(0.0795808873001328,7.10259971193733,
0.));
#14116=CARTESIAN_POINT('Ctrl Pts',(-0.251664502419995,7.39978648873079,
-0.161258330249198));
#14117=CARTESIAN_POINT('Ctrl Pts',(-0.251853743060092,7.37731968999655,
-0.15983892928355));
#14118=CARTESIAN_POINT('Ctrl Pts',(-0.249087060170416,7.35489869942726,
-0.158419528317902));
#14119=CARTESIAN_POINT('Ctrl Pts',(-0.243177144710154,7.33333937551853,
-0.157000127352253));
#14120=CARTESIAN_POINT('Ctrl Pts',(-0.221387260518207,7.25385005382068,
-0.151766789773845));
#14121=CARTESIAN_POINT('Ctrl Pts',(-0.156868268663584,7.18607422982997,
-0.146533452195437));
#14122=CARTESIAN_POINT('Ctrl Pts',(-0.0785474512786524,7.16039843377808,
-0.141300114617028));
#14123=CARTESIAN_POINT('Ctrl Pts',(-0.00022663389372081,7.13472263772619,
-0.13606677703862));
#14124=CARTESIAN_POINT('Ctrl Pts',(0.0918960090215198,7.15114686961312,
-0.130833439460211));
#14125=CARTESIAN_POINT('Ctrl Pts',(0.156516611947103,7.20230943571013,-0.125600101881803));
#14126=CARTESIAN_POINT('Ctrl Pts',(0.221137214872687,7.25347200180715,-0.120366764303394));
#14127=CARTESIAN_POINT('Ctrl Pts',(0.258255777808613,7.33937290211427,-0.115133426724986));
#14128=CARTESIAN_POINT('Ctrl Pts',(0.251230492354282,7.42149364017549,-0.109900089146577));
#14129=CARTESIAN_POINT('Ctrl Pts',(0.244205206899952,7.50361437823672,-0.104666751568169));
#14130=CARTESIAN_POINT('Ctrl Pts',(0.193036073055365,7.58195495405205,-0.0994334139897605));
#14131=CARTESIAN_POINT('Ctrl Pts',(0.120664054720216,7.62139990068305,-0.0942000764113521));
#14132=CARTESIAN_POINT('Ctrl Pts',(0.0482920363850678,7.66084484731404,
-0.0889667388329436));
#14133=CARTESIAN_POINT('Ctrl Pts',(-0.0452828664406417,7.66139416476069,
-0.0837334012545352));
#14134=CARTESIAN_POINT('Ctrl Pts',(-0.118103955917399,7.6227836008624,-0.0785000636761267));
#14135=CARTESIAN_POINT('Ctrl Pts',(-0.190925045394156,7.5841730369641,-0.0732667260977183));
#14136=CARTESIAN_POINT('Ctrl Pts',(-0.242992321521962,7.50640259172086,
-0.0680333885193098));
#14137=CARTESIAN_POINT('Ctrl Pts',(-0.25096508216279,7.42437725852632,-0.0628000509409014));
#14138=CARTESIAN_POINT('Ctrl Pts',(-0.251747996817527,7.41632247821737,
-0.0622861440436668));
#14139=CARTESIAN_POINT('Ctrl Pts',(-0.252105708816997,7.40822666809701,
-0.0617722371464322));
#14140=CARTESIAN_POINT('Ctrl Pts',(-0.252053546614158,7.40012638988493,
-0.0612583302491975));
#14141=CARTESIAN_POINT('Ctrl Pts',(-0.0793799282532879,7.10307770462543,
5.55111512312578E-17));
#14142=CARTESIAN_POINT('Ctrl Pts',(-0.177014005842308,7.12917943627315,
-0.00523333757840839));
#14143=CARTESIAN_POINT('Ctrl Pts',(-0.342929363773459,7.28476228830982,
-0.0157000127352253));
#14144=CARTESIAN_POINT('Ctrl Pts',(-0.285303662486741,7.6230159413608,-0.0314000254704506));
#14145=CARTESIAN_POINT('Ctrl Pts',(0.0286357548570192,7.76072194419717,
-0.047100038205676));
#14146=CARTESIAN_POINT('Ctrl Pts',(0.316662279094702,7.57523911945597,-0.0628000509409012));
#14147=CARTESIAN_POINT('Ctrl Pts',(0.320851004579023,7.23248257807725,-0.0785000636761267));
#14148=CARTESIAN_POINT('Ctrl Pts',(0.037271918951097,7.04000744673753,-0.094200076411352));
#14149=CARTESIAN_POINT('Ctrl Pts',(-0.279700685926573,7.17030791937543,
-0.109900089146577));
#14150=CARTESIAN_POINT('Ctrl Pts',(-0.345877162555279,7.50659192636033,
-0.125600101881803));
#14151=CARTESIAN_POINT('Ctrl Pts',(-0.101895250628719,7.74728578061798,
-0.141300114617028));
#14152=CARTESIAN_POINT('Ctrl Pts',(0.233453631148172,7.67656918324398,-0.157000127352253));
#14153=CARTESIAN_POINT('Ctrl Pts',(0.359464126606772,7.35784834370038,-0.172700140087479));
#14154=CARTESIAN_POINT('Ctrl Pts',(0.163138836475842,7.07692629120202,-0.188400152822704));
#14155=CARTESIAN_POINT('Ctrl Pts',(-0.179474189751402,7.08570704088486,
-0.20410016555793));
#14156=CARTESIAN_POINT('Ctrl Pts',(-0.361151198222271,7.37631754602761,
-0.219800178293155));
#14157=CARTESIAN_POINT('Ctrl Pts',(-0.218980358434117,7.68816421398779,
-0.23550019102838));
#14158=CARTESIAN_POINT('Ctrl Pts',(0.119552217972776,7.7416113266484,-0.251200203763606));
#14159=CARTESIAN_POINT('Ctrl Pts',(0.350881199163606,7.48873225573956,-0.266900216498831));
#14160=CARTESIAN_POINT('Ctrl Pts',(0.267571630187383,7.15628613456826,-0.282600229234056));
#14161=CARTESIAN_POINT('Ctrl Pts',(-0.0556719802611724,7.04238056731933,
-0.298300241969282));
#14162=CARTESIAN_POINT('Ctrl Pts',(-0.328993995030839,7.24915577981674,
-0.314000254704507));
#14163=CARTESIAN_POINT('Ctrl Pts',(-0.307303936687348,7.59119444989383,
-0.329700267439732));
#14164=CARTESIAN_POINT('Ctrl Pts',(-0.0100514909408711,7.76178722340353,
-0.345400280174958));
#14165=CARTESIAN_POINT('Ctrl Pts',(0.296214223541038,7.60796192241644,-0.361100292910183));
#14166=CARTESIAN_POINT('Ctrl Pts',(0.336861801835373,7.26765517072256,-0.376800305645408));
#14167=CARTESIAN_POINT('Ctrl Pts',(0.0754421708108413,7.04602329698811,
-0.392500318380633));
#14168=CARTESIAN_POINT('Ctrl Pts',(-0.253627178584431,7.14180572880535,
-0.408200331115859));
#14169=CARTESIAN_POINT('Ctrl Pts',(-0.355266603733067,7.46911344056264,
-0.423900343851084));
#14170=CARTESIAN_POINT('Ctrl Pts',(-0.138335057048331,7.73444646717113,
-0.43960035658631));
#14171=CARTESIAN_POINT('Ctrl Pts',(0.202642862416027,7.69987813805627,-0.455300369321535));
#14172=CARTESIAN_POINT('Ctrl Pts',(0.361908983097054,7.39640620579093,-0.47100038205676));
#14173=CARTESIAN_POINT('Ctrl Pts',(0.196647846607491,7.09615686298222,-0.486700394791986));
#14174=CARTESIAN_POINT('Ctrl Pts',(-0.144949300426615,7.06836657665492,
-0.502400407527211));
#14175=CARTESIAN_POINT('Ctrl Pts',(-0.356569019314508,7.33795516142226,
-0.518100420262437));
#14176=CARTESIAN_POINT('Ctrl Pts',(-0.248449877558159,7.66317995052507,
-0.533800432997661));
#14177=CARTESIAN_POINT('Ctrl Pts',(0.0824566524067525,7.75240874841395,
-0.549500445732887));
#14178=CARTESIAN_POINT('Ctrl Pts',(0.339423512150486,7.52562925031437,-0.565200458468112));
#14179=CARTESIAN_POINT('Ctrl Pts',(0.292026050158285,7.1861967789166,-0.580900471203337));
#14180=CARTESIAN_POINT('Ctrl Pts',(-0.0172339683272763,7.03848374595487,
-0.596600483938563));
#14181=CARTESIAN_POINT('Ctrl Pts',(-0.311040130662272,7.21494572763339,
-0.612300496673788));
#14182=CARTESIAN_POINT('Ctrl Pts',(-0.325933606530968,7.55734780923163,
-0.628000509409014));
#14183=CARTESIAN_POINT('Ctrl Pts',(-0.0485593254958618,7.75865428087583,
-0.643700522144239));
#14184=CARTESIAN_POINT('Ctrl Pts',(0.27235863905538,7.63835266345873,-0.659400534879465));
#14185=CARTESIAN_POINT('Ctrl Pts',(0.349049856868627,7.30431662403272,-0.67510054761469));
#14186=CARTESIAN_POINT('Ctrl Pts',(0.112745006295209,7.05608341261925,-0.690800560349915));
#14187=CARTESIAN_POINT('Ctrl Pts',(-0.224659951867446,7.11623820488055,
-0.70650057308514));
#14188=CARTESIAN_POINT('Ctrl Pts',(-0.360609008143163,7.4308556130298,-0.722200585820366));
#14189=CARTESIAN_POINT('Ctrl Pts',(-0.173198863217152,7.71778292610997,
-0.73790059855559));
#14190=CARTESIAN_POINT('Ctrl Pts',(0.169525116851479,7.71979476003134,-0.753600611290817));
#14191=CARTESIAN_POINT('Ctrl Pts',(0.360224711692468,7.43495575882791,-0.769300624026041));
#14192=CARTESIAN_POINT('Ctrl Pts',(0.227926662850033,7.11894882344372,-0.785000636761268));
#14193=CARTESIAN_POINT('Ctrl Pts',(-0.108793818048451,7.05460429203039,
-0.800700649496493));
#14194=CARTESIAN_POINT('Ctrl Pts',(-0.34788417951995,7.30071819716892,-0.816400662231718));
#14195=CARTESIAN_POINT('Ctrl Pts',(-0.29928159504458,7.52291567381437,-0.826867337388535));
#14196=CARTESIAN_POINT('Ctrl Pts',(-0.233606265769613,7.59973015569307,
-0.832100674966943));
#14197=CARTESIAN_POINT('Ctrl Pts',(-0.0745932854346959,7.12098224301579,
0.0107002249889811));
#14198=CARTESIAN_POINT('Ctrl Pts',(-0.166339987378199,7.14551002934643,
0.00546688741057267));
#14199=CARTESIAN_POINT('Ctrl Pts',(-0.322250579948499,7.291711170442,-0.00499978774624421));
#14200=CARTESIAN_POINT('Ctrl Pts',(-0.268099732510858,7.60956798697692,
-0.0206998004814696));
#14201=CARTESIAN_POINT('Ctrl Pts',(0.026909006882343,7.73897026034341,-0.0363998132166949));
#14202=CARTESIAN_POINT('Ctrl Pts',(0.297567411443636,7.56467212738206,-0.0520998259519203));
#14203=CARTESIAN_POINT('Ctrl Pts',(0.301503555032259,7.24258394856573,-0.0677998386871455));
#14204=CARTESIAN_POINT('Ctrl Pts',(0.0350244066755359,7.06171514801338,
-0.083499851422371));
#14205=CARTESIAN_POINT('Ctrl Pts',(-0.262834617776779,7.18415844774452,
-0.0991998641575963));
#14206=CARTESIAN_POINT('Ctrl Pts',(-0.325020625232928,7.50016438869357,
-0.114899876892822));
#14207=CARTESIAN_POINT('Ctrl Pts',(-0.0957509244696644,7.72634430303828,
-0.130599889628047));
#14208=CARTESIAN_POINT('Ctrl Pts',(0.219376279711874,7.6598919460135,-0.146299902363272));
#14209=CARTESIAN_POINT('Ctrl Pts',(0.337788289678909,7.36039010617557,-0.161999915098498));
#14210=CARTESIAN_POINT('Ctrl Pts',(0.153301496518078,7.09640777074127,-0.177699927833723));
#14211=CARTESIAN_POINT('Ctrl Pts',(-0.168651821170329,7.10465903755185,
-0.193399940568948));
#14212=CARTESIAN_POINT('Ctrl Pts',(-0.33937363017156,7.3777456078907,-0.209099953304174));
#14213=CARTESIAN_POINT('Ctrl Pts',(-0.20577575138576,7.67078779156197,-0.224799966039399));
#14214=CARTESIAN_POINT('Ctrl Pts',(0.112343169310245,7.72101202101242,-0.240499978774624));
#14215=CARTESIAN_POINT('Ctrl Pts',(0.329722916344349,7.48338166366851,-0.25619999150985));
#14216=CARTESIAN_POINT('Ctrl Pts',(0.251436949163123,7.17098218241599,-0.271900004245075));
#14217=CARTESIAN_POINT('Ctrl Pts',(-0.052314936605708,7.06394516843321,
-0.287600016980301));
#14218=CARTESIAN_POINT('Ctrl Pts',(-0.309155519759742,7.25825174927847,
-0.303300029715525));
#14219=CARTESIAN_POINT('Ctrl Pts',(-0.288773380991002,7.5796653447324,-0.319000042450752));
#14220=CARTESIAN_POINT('Ctrl Pts',(-0.00944538184015792,7.73997130276882,
-0.334700055185976));
#14221=CARTESIAN_POINT('Ctrl Pts',(0.278352382177899,7.59542173166067,-0.350400067921202));
#14222=CARTESIAN_POINT('Ctrl Pts',(0.316548894528777,7.27563561918828,-0.366100080656427));
#14223=CARTESIAN_POINT('Ctrl Pts',(0.0708929764102307,7.06736823998195,
-0.381800093391652));
#14224=CARTESIAN_POINT('Ctrl Pts',(-0.238333353814305,7.15737495116686,
-0.397500106126878));
#14225=CARTESIAN_POINT('Ctrl Pts',(-0.333843879187155,7.46494587123854,
-0.413200118862103));
#14226=CARTESIAN_POINT('Ctrl Pts',(-0.12999339534681,7.71427920555331,-0.428900131597329));
#14227=CARTESIAN_POINT('Ctrl Pts',(0.190423413199248,7.68179536111799,-0.444600144332554));
#14228=CARTESIAN_POINT('Ctrl Pts',(0.340085720301983,7.39662291308232,-0.460300157067779));
#14229=CARTESIAN_POINT('Ctrl Pts',(0.184789899347173,7.11447873101343,-0.476000169803005));
#14230=CARTESIAN_POINT('Ctrl Pts',(-0.136208797087621,7.08836421055545,
-0.49170018253823));
#14231=CARTESIAN_POINT('Ctrl Pts',(-0.335067758565214,7.34169649109518,
-0.507400195273455));
#14232=CARTESIAN_POINT('Ctrl Pts',(-0.233468246201688,7.64731008961818,
-0.523100208008681));
#14233=CARTESIAN_POINT('Ctrl Pts',(0.0774844818370269,7.73115835373707,
-0.538800220743906));
#14234=CARTESIAN_POINT('Ctrl Pts',(0.318956132642252,7.51805375406419,-0.554500233479132));
#14235=CARTESIAN_POINT('Ctrl Pts',(0.274416757398889,7.199089202421,-0.570200246214356));
#14236=CARTESIAN_POINT('Ctrl Pts',(-0.016194752841135,7.06028332702413,
-0.585900258949582));
#14237=CARTESIAN_POINT('Ctrl Pts',(-0.292284280909198,7.22610457752611,
-0.601600271684807));
#14238=CARTESIAN_POINT('Ctrl Pts',(-0.306279673964272,7.54785967063472,
-0.617300284420033));
#14239=CARTESIAN_POINT('Ctrl Pts',(-0.0456311778926191,7.7370272779837,
-0.633000297155258));
#14240=CARTESIAN_POINT('Ctrl Pts',(0.255935299397576,7.62397989832853,-0.648700309890484));
#14241=CARTESIAN_POINT('Ctrl Pts',(0.328002004754429,7.31008637155593,-0.664400322625709));
#14242=CARTESIAN_POINT('Ctrl Pts',(0.105946435339172,7.07682172643994,-0.680100335360934));
#14243=CARTESIAN_POINT('Ctrl Pts',(-0.211112862963559,7.13334915961038,
-0.695800348096159));
#14244=CARTESIAN_POINT('Ctrl Pts',(-0.338864134380612,7.42899500668041,
-0.711500360831385));
#14245=CARTESIAN_POINT('Ctrl Pts',(-0.162754899446344,7.69862048297595,
-0.72720037356661));
#14246=CARTESIAN_POINT('Ctrl Pts',(0.159302681520486,7.70051100247185,-0.742900386301834));
#14247=CARTESIAN_POINT('Ctrl Pts',(0.338503011166357,7.43284791197487,-0.758600399037062));
#14248=CARTESIAN_POINT('Ctrl Pts',(0.214182589909887,7.13589632674239,-0.774300411772284));
#14249=CARTESIAN_POINT('Ctrl Pts',(-0.102233505393505,7.07543179744019,
-0.790000424507513));
#14250=CARTESIAN_POINT('Ctrl Pts',(-0.326906618236604,7.30670493133454,
-0.805700437242736));
#14251=CARTESIAN_POINT('Ctrl Pts',(-0.281234789899004,7.51550380736019,
-0.816167112399554));
#14252=CARTESIAN_POINT('Ctrl Pts',(-0.21951971040191,7.58768634390788,-0.821400449977962));
#14253=CARTESIAN_POINT('Ctrl Pts',(-0.0698066426161039,7.13888678140614,
0.0214004499779622));
#14254=CARTESIAN_POINT('Ctrl Pts',(-0.155665968914089,7.1618406224197,0.0161671123995537));
#14255=CARTESIAN_POINT('Ctrl Pts',(-0.301571796123539,7.29866005257418,
0.00570043724273684));
#14256=CARTESIAN_POINT('Ctrl Pts',(-0.250895802534975,7.59612003259303,
-0.00999957549248849));
#14257=CARTESIAN_POINT('Ctrl Pts',(0.0251822589076668,7.71721857648964,
-0.0256995882277138));
#14258=CARTESIAN_POINT('Ctrl Pts',(0.27847254379257,7.55410513530815,-0.0413996009629392));
#14259=CARTESIAN_POINT('Ctrl Pts',(0.282156105485495,7.25268531905421,-0.0570996136981645));
#14260=CARTESIAN_POINT('Ctrl Pts',(0.0327768943999749,7.08342284928922,
-0.0727996264333899));
#14261=CARTESIAN_POINT('Ctrl Pts',(-0.245968549626985,7.19800897611362,
-0.0884996391686152));
#14262=CARTESIAN_POINT('Ctrl Pts',(-0.304164087910577,7.49373685102681,
-0.104199651903841));
#14263=CARTESIAN_POINT('Ctrl Pts',(-0.089606598310609,7.70540282545859,
-0.119899664639066));
#14264=CARTESIAN_POINT('Ctrl Pts',(0.205298928275576,7.64321470878302,-0.135599677374291));
#14265=CARTESIAN_POINT('Ctrl Pts',(0.316112452751045,7.36293186865078,-0.151299690109517));
#14266=CARTESIAN_POINT('Ctrl Pts',(0.143464156560313,7.11588925028052,-0.166999702844742));
#14267=CARTESIAN_POINT('Ctrl Pts',(-0.157829452589257,7.12361103421885,
-0.182699715579967));
#14268=CARTESIAN_POINT('Ctrl Pts',(-0.317596062120848,7.3791736697538,-0.198399728315193));
#14269=CARTESIAN_POINT('Ctrl Pts',(-0.192571144337404,7.65341136913615,
-0.214099741050418));
#14270=CARTESIAN_POINT('Ctrl Pts',(0.105134120647715,7.70041271537645,-0.229799753785644));
#14271=CARTESIAN_POINT('Ctrl Pts',(0.308564633525091,7.47803107159744,-0.245499766520869));
#14272=CARTESIAN_POINT('Ctrl Pts',(0.235302268138864,7.18567823026373,-0.261199779256094));
#14273=CARTESIAN_POINT('Ctrl Pts',(-0.0489578929502435,7.08550976954708,
-0.276899791991319));
#14274=CARTESIAN_POINT('Ctrl Pts',(-0.289317044488645,7.26734771874021,
-0.292599804726545));
#14275=CARTESIAN_POINT('Ctrl Pts',(-0.270242825294655,7.56813623957097,
-0.30829981746177));
#14276=CARTESIAN_POINT('Ctrl Pts',(-0.00883927273944482,7.71815538213412,
-0.323999830196996));
#14277=CARTESIAN_POINT('Ctrl Pts',(0.260490540814761,7.5828815409049,-0.33969984293222));
#14278=CARTESIAN_POINT('Ctrl Pts',(0.296235987222181,7.28361606765402,-0.355399855667446));
#14279=CARTESIAN_POINT('Ctrl Pts',(0.0663437820096206,7.08871318297577,
-0.371099868402671));
#14280=CARTESIAN_POINT('Ctrl Pts',(-0.22303952904418,7.17294417352836,-0.386799881137897));
#14281=CARTESIAN_POINT('Ctrl Pts',(-0.312421154641242,7.46077830191444,
-0.402499893873122));
#14282=CARTESIAN_POINT('Ctrl Pts',(-0.12165173364529,7.69411194393548,-0.418199906608348));
#14283=CARTESIAN_POINT('Ctrl Pts',(0.178203963982469,7.66371258417972,-0.433899919343573));
#14284=CARTESIAN_POINT('Ctrl Pts',(0.31826245750691,7.39683962037371,-0.449599932078798));
#14285=CARTESIAN_POINT('Ctrl Pts',(0.172931952086855,7.13280059904465,-0.465299944814023));
#14286=CARTESIAN_POINT('Ctrl Pts',(-0.127468293748627,7.108361844456,-0.480999957549249));
#14287=CARTESIAN_POINT('Ctrl Pts',(-0.31356649781592,7.3454378207681,-0.496699970284474));
#14288=CARTESIAN_POINT('Ctrl Pts',(-0.218486614845218,7.63144022871131,
-0.512399983019699));
#14289=CARTESIAN_POINT('Ctrl Pts',(0.0725123112673016,7.70990795906018,
-0.528099995754925));
#14290=CARTESIAN_POINT('Ctrl Pts',(0.298488753134019,7.51047825781402,-0.54380000849015));
#14291=CARTESIAN_POINT('Ctrl Pts',(0.256807464639494,7.2119816259254,-0.559500021225375));
#14292=CARTESIAN_POINT('Ctrl Pts',(-0.0151555373549939,7.08208290809339,
-0.575200033960601));
#14293=CARTESIAN_POINT('Ctrl Pts',(-0.273528431156123,7.23726342741883,
-0.590900046695826));
#14294=CARTESIAN_POINT('Ctrl Pts',(-0.286625741397577,7.53837153203782,
-0.606600059431052));
#14295=CARTESIAN_POINT('Ctrl Pts',(-0.0427030302893763,7.71540027509155,
-0.622300072166277));
#14296=CARTESIAN_POINT('Ctrl Pts',(0.23951195973977,7.60960713319833,-0.638000084901503));
#14297=CARTESIAN_POINT('Ctrl Pts',(0.306954152640232,7.31585611907914,-0.653700097636727));
#14298=CARTESIAN_POINT('Ctrl Pts',(0.0991478643831351,7.09756004026064,
-0.669400110371954));
#14299=CARTESIAN_POINT('Ctrl Pts',(-0.19756577405967,7.15046011434021,-0.685100123107178));
#14300=CARTESIAN_POINT('Ctrl Pts',(-0.317119260618062,7.42713440033102,
-0.700800135842404));
#14301=CARTESIAN_POINT('Ctrl Pts',(-0.152310935675535,7.67945803984195,
-0.716500148577629));
#14302=CARTESIAN_POINT('Ctrl Pts',(0.149080246189493,7.68122724491234,-0.732200161312854));
#14303=CARTESIAN_POINT('Ctrl Pts',(0.316781310640245,7.43074006512186,-0.74790017404808));
#14304=CARTESIAN_POINT('Ctrl Pts',(0.20043851696974,7.15284383004104,-0.763600186783305));
#14305=CARTESIAN_POINT('Ctrl Pts',(-0.0956731927385576,7.09625930285,-0.779300199518531));
#14306=CARTESIAN_POINT('Ctrl Pts',(-0.305929056953258,7.31269166550016,
-0.795000212253756));
#14307=CARTESIAN_POINT('Ctrl Pts',(-0.263187984753428,7.508091940906,-0.805466887410573));
#14308=CARTESIAN_POINT('Ctrl Pts',(-0.205433155034207,7.57564253212269,
-0.810700224988981));
#14309=CARTESIAN_POINT('Ctrl Pts',(-0.065019999797512,7.15679131979649,
0.0321006749669432));
#14310=CARTESIAN_POINT('Ctrl Pts',(-0.14499195044998,7.17817121549298,0.0268673373885348));
#14311=CARTESIAN_POINT('Ctrl Pts',(-0.280893012298579,7.30560893470636,
0.0164006622317179));
#14312=CARTESIAN_POINT('Ctrl Pts',(-0.233691872559092,7.58267207820915,
0.000700649496492578));
#14313=CARTESIAN_POINT('Ctrl Pts',(0.0234555109329906,7.69546689263588,
-0.0149993632387328));
#14314=CARTESIAN_POINT('Ctrl Pts',(0.259377676141504,7.54353814323423,-0.0306993759739581));
#14315=CARTESIAN_POINT('Ctrl Pts',(0.262808655938731,7.26278668954269,-0.0463993887091835));
#14316=CARTESIAN_POINT('Ctrl Pts',(0.0305293821244139,7.10513055056507,
-0.0620994014444087));
#14317=CARTESIAN_POINT('Ctrl Pts',(-0.229102481477192,7.21185950448272,
-0.0777994141796342));
#14318=CARTESIAN_POINT('Ctrl Pts',(-0.283307550588226,7.48730931336005,
-0.0934994269148594));
#14319=CARTESIAN_POINT('Ctrl Pts',(-0.083462272151554,7.68446134787889,
-0.109199439650085));
#14320=CARTESIAN_POINT('Ctrl Pts',(0.191221576839279,7.62653747155253,-0.12489945238531));
#14321=CARTESIAN_POINT('Ctrl Pts',(0.294436615823181,7.36547363112598,-0.140599465120536));
#14322=CARTESIAN_POINT('Ctrl Pts',(0.133626816602548,7.13537072981977,-0.156299477855761));
#14323=CARTESIAN_POINT('Ctrl Pts',(-0.147007084008184,7.14256303088585,
-0.171999490590986));
#14324=CARTESIAN_POINT('Ctrl Pts',(-0.295818494070137,7.38060173161688,
-0.187699503326212));
#14325=CARTESIAN_POINT('Ctrl Pts',(-0.179366537289048,7.63603494671035,
-0.203399516061437));
#14326=CARTESIAN_POINT('Ctrl Pts',(0.0979250719851847,7.67981340974047,
-0.219099528796663));
#14327=CARTESIAN_POINT('Ctrl Pts',(0.287406350705833,7.47268047952639,-0.234799541531887));
#14328=CARTESIAN_POINT('Ctrl Pts',(0.219167587114604,7.20037427811147,-0.250499554267113));
#14329=CARTESIAN_POINT('Ctrl Pts',(-0.045600849294779,7.10707437066095,
-0.266199567002338));
#14330=CARTESIAN_POINT('Ctrl Pts',(-0.269478569217549,7.27644368820193,
-0.281899579737564));
#14331=CARTESIAN_POINT('Ctrl Pts',(-0.251712269598308,7.55660713440954,
-0.297599592472789));
#14332=CARTESIAN_POINT('Ctrl Pts',(-0.00823316363873174,7.6963394614994,
-0.313299605208015));
#14333=CARTESIAN_POINT('Ctrl Pts',(0.242628699451623,7.57034135014914,-0.328999617943239));
#14334=CARTESIAN_POINT('Ctrl Pts',(0.275923079915585,7.29159651611974,-0.344699630678465));
#14335=CARTESIAN_POINT('Ctrl Pts',(0.0617945876090101,7.11005812596961,
-0.36039964341369));
#14336=CARTESIAN_POINT('Ctrl Pts',(-0.207745704274054,7.18851339588986,
-0.376099656148916));
#14337=CARTESIAN_POINT('Ctrl Pts',(-0.290998430095329,7.45661073259035,
-0.391799668884141));
#14338=CARTESIAN_POINT('Ctrl Pts',(-0.113310071943769,7.67394468231766,
-0.407499681619367));
#14339=CARTESIAN_POINT('Ctrl Pts',(0.16598451476569,7.64562980724146,-0.423199694354591));
#14340=CARTESIAN_POINT('Ctrl Pts',(0.296439194711838,7.39705632766509,-0.438899707089818));
#14341=CARTESIAN_POINT('Ctrl Pts',(0.161074004826536,7.15112246707589,-0.454599719825042));
#14342=CARTESIAN_POINT('Ctrl Pts',(-0.118727790409632,7.12835947835651,
-0.470299732560268));
#14343=CARTESIAN_POINT('Ctrl Pts',(-0.292065237066626,7.34917915044104,
-0.485999745295493));
#14344=CARTESIAN_POINT('Ctrl Pts',(-0.203504983488747,7.61557036780441,
-0.501699758030719));
#14345=CARTESIAN_POINT('Ctrl Pts',(0.0675401406975761,7.68865756438332,
-0.517399770765944));
#14346=CARTESIAN_POINT('Ctrl Pts',(0.278021373625785,7.50290276156383,-0.533099783501169));
#14347=CARTESIAN_POINT('Ctrl Pts',(0.239198171880098,7.22487404942981,-0.548799796236395));
#14348=CARTESIAN_POINT('Ctrl Pts',(-0.0141163218688527,7.10388248916265,
-0.56449980897162));
#14349=CARTESIAN_POINT('Ctrl Pts',(-0.254772581403049,7.24842227731155,
-0.580199821706845));
#14350=CARTESIAN_POINT('Ctrl Pts',(-0.266971808830881,7.52888339344091,
-0.595899834442071));
#14351=CARTESIAN_POINT('Ctrl Pts',(-0.0397748826861335,7.69377327219942,
-0.611599847177295));
#14352=CARTESIAN_POINT('Ctrl Pts',(0.223088620081966,7.59523436806812,-0.627299859912522));
#14353=CARTESIAN_POINT('Ctrl Pts',(0.285906300526035,7.32162586660236,-0.642999872647746));
#14354=CARTESIAN_POINT('Ctrl Pts',(0.0923492934270986,7.11829835408133,
-0.658699885382973));
#14355=CARTESIAN_POINT('Ctrl Pts',(-0.184018685155783,7.16757106907005,
-0.674399898118197));
#14356=CARTESIAN_POINT('Ctrl Pts',(-0.295374386855511,7.42527379398162,
-0.690099910853423));
#14357=CARTESIAN_POINT('Ctrl Pts',(-0.141866971904727,7.66029559670794,
-0.705799923588648));
#14358=CARTESIAN_POINT('Ctrl Pts',(0.1388578108585,7.66194348735283,-0.721499936323873));
#14359=CARTESIAN_POINT('Ctrl Pts',(0.295059610114134,7.42863221826883,-0.737199949059098));
#14360=CARTESIAN_POINT('Ctrl Pts',(0.186694444029594,7.1697913333397,-0.752899961794324));
#14361=CARTESIAN_POINT('Ctrl Pts',(-0.0891128800836106,7.11708680825981,
-0.76859997452955));
#14362=CARTESIAN_POINT('Ctrl Pts',(-0.284951495669912,7.31867839966577,
-0.784299987264775));
#14363=CARTESIAN_POINT('Ctrl Pts',(-0.245141179607851,7.50068007445182,
-0.794766662421592));
#14364=CARTESIAN_POINT('Ctrl Pts',(-0.191346599666504,7.5635987203375,-0.8));
#14365=CARTESIAN_POINT('Ctrl Pts',(-0.25159361924534,7.40020120251426,-0.088741669750802));
#14366=CARTESIAN_POINT('Ctrl Pts',(-0.251789088068147,7.4253219403653,-0.0903275888054879));
#14367=CARTESIAN_POINT('Ctrl Pts',(-0.248321666625649,7.45039001357577,
-0.0919135078601738));
#14368=CARTESIAN_POINT('Ctrl Pts',(-0.240965825996942,7.4742596843003,-0.0934994269148597));
#14369=CARTESIAN_POINT('Ctrl Pts',(-0.216692457776002,7.55302665819966,
-0.0987327644932681));
#14370=CARTESIAN_POINT('Ctrl Pts',(-0.150077364963778,7.61874400303928,
-0.103966102071677));
#14371=CARTESIAN_POINT('Ctrl Pts',(-0.070989177059194,7.64194869607136,
-0.109199439650085));
#14372=CARTESIAN_POINT('Ctrl Pts',(0.00809901084539029,7.66515338910344,
-0.114432777228493));
#14373=CARTESIAN_POINT('Ctrl Pts',(0.0996602938423346,7.64584543032799,
-0.119666114806902));
#14374=CARTESIAN_POINT('Ctrl Pts',(0.162643441838124,7.59268081086917,-0.12489945238531));
#14375=CARTESIAN_POINT('Ctrl Pts',(0.225626589833913,7.53951619141035,-0.130132789963719));
#14376=CARTESIAN_POINT('Ctrl Pts',(0.260031602828547,7.45249491126816,-0.135366127542127));
#14377=CARTESIAN_POINT('Ctrl Pts',(0.250432476122426,7.37063378764604,-0.140599465120536));
#14378=CARTESIAN_POINT('Ctrl Pts',(0.240833349416304,7.28877266402391,-0.145832802698944));
#14379=CARTESIAN_POINT('Ctrl Pts',(0.187230083009426,7.21207169692184,-0.151066140277353));
#14380=CARTESIAN_POINT('Ctrl Pts',(0.113656133037532,7.17491993021515,-0.156299477855761));
#14381=CARTESIAN_POINT('Ctrl Pts',(0.0400821830656374,7.13776816350846,
-0.161532815434169));
#14382=CARTESIAN_POINT('Ctrl Pts',(-0.0534624504712735,7.14016559719716,
-0.166766153012578));
#14383=CARTESIAN_POINT('Ctrl Pts',(-0.125036668916721,7.18103743083001,
-0.171999490590986));
#14384=CARTESIAN_POINT('Ctrl Pts',(-0.196610887362169,7.22190926446286,
-0.177232828169395));
#14385=CARTESIAN_POINT('Ctrl Pts',(-0.246214690716153,7.30125549803987,
-0.182466165747803));
#14386=CARTESIAN_POINT('Ctrl Pts',(-0.25160793292963,7.38350081734395,-0.187699503326212));
#14387=CARTESIAN_POINT('Ctrl Pts',(-0.251965936203217,7.38896025943511,
-0.188046892134409));
#14388=CARTESIAN_POINT('Ctrl Pts',(-0.252129134444029,7.39443247577015,
-0.188394280942605));
#14389=CARTESIAN_POINT('Ctrl Pts',(-0.252102618136395,7.39990630057405,
-0.188741669750802));
#14390=CARTESIAN_POINT('Ctrl Pts',(-0.0793799282532879,7.10307770462543,
5.55111512312578E-17));
#14391=CARTESIAN_POINT('Ctrl Pts',(-0.0961911438687228,7.10922732239277,
6.3088022331286E-17));
#14392=CARTESIAN_POINT('Ctrl Pts',(-0.112330824293046,7.11692875641727,
7.51298486027343E-17));
#14393=CARTESIAN_POINT('Ctrl Pts',(-0.127669362876862,7.1259997700432,8.37004077158809E-17));
#14394=CARTESIAN_POINT('Ctrl Pts',(-0.137645054815231,7.13189926542253,
8.92744235835032E-17));
#14395=CARTESIAN_POINT('Ctrl Pts',(-0.147281435088536,7.1383791577173,7.60600198292336E-17));
#14396=CARTESIAN_POINT('Ctrl Pts',(-0.156535227934782,7.14539793713334,
8.06646416329215E-17));
#14397=CARTESIAN_POINT('Ctrl Pts',(-0.16394892482158,7.15102104799938,8.43536447150178E-17));
#14398=CARTESIAN_POINT('Ctrl Pts',(-0.171116962103292,7.15699019329351,
4.93210431432864E-17));
#14399=CARTESIAN_POINT('Ctrl Pts',(-0.178013423245633,7.16328599091072,
3.46944695195361E-17));
#14400=CARTESIAN_POINT('Ctrl Pts',(-0.181540425610593,7.16650580069822,
2.72141171043684E-17));
#14401=CARTESIAN_POINT('Ctrl Pts',(-0.184990066957579,7.16980542739394,
7.26266936595826E-17));
#14402=CARTESIAN_POINT('Ctrl Pts',(-0.188356628917223,7.17317858145051,
7.28583859910259E-17));
#14403=CARTESIAN_POINT('Ctrl Pts',(-0.200715855331018,7.18556200858287,
7.37089682814972E-17));
#14404=CARTESIAN_POINT('Ctrl Pts',(-0.211972685909792,7.19894710696887,
9.45510976419299E-17));
#14405=CARTESIAN_POINT('Ctrl Pts',(-0.22197690688827,7.21318605721376,1.07552855510562E-16));
#14406=CARTESIAN_POINT('Ctrl Pts',(-0.228265864693712,7.22213709472849,
1.15726156241153E-16));
#14407=CARTESIAN_POINT('Ctrl Pts',(-0.234059012930639,7.23142615662503,
5.59373896742589E-17));
#14408=CARTESIAN_POINT('Ctrl Pts',(-0.239308852044784,7.24101980913937,
5.20417042793042E-17));
#14409=CARTESIAN_POINT('Ctrl Pts',(-0.241553615206904,7.24512193061131,
5.03759596963439E-17));
#14410=CARTESIAN_POINT('Ctrl Pts',(-0.243698936078229,7.24927975670907,
3.19182285479356E-17));
#14411=CARTESIAN_POINT('Ctrl Pts',(-0.245740587550779,7.25349070851309,
3.46944695195361E-17));
#14412=CARTESIAN_POINT('Ctrl Pts',(-0.247686902746868,7.25750502711564,
3.73410720683434E-17));
#14413=CARTESIAN_POINT('Ctrl Pts',(-0.249535087968469,7.26155962917014,
8.85331702759656E-17));
#14414=CARTESIAN_POINT('Ctrl Pts',(-0.251281746281186,7.26565003442524,
8.84708972748172E-17));
#14415=CARTESIAN_POINT('Ctrl Pts',(-0.257537589409274,7.28030025732224,
8.82478598762239E-17));
#14416=CARTESIAN_POINT('Ctrl Pts',(-0.262498392567991,7.29541738447504,
6.01328869974533E-17));
#14417=CARTESIAN_POINT('Ctrl Pts',(-0.266024737720578,7.31089144318791,
6.93889390390723E-17));
#14418=CARTESIAN_POINT('Ctrl Pts',(-0.268541655860434,7.32193600558507,
7.60750141973437E-17));
#14419=CARTESIAN_POINT('Ctrl Pts',(-0.270326735192568,7.33316280454067,
8.51582814892351E-17));
#14420=CARTESIAN_POINT('Ctrl Pts',(-0.27139185115298,7.34450305084133,9.36750677027476E-17));
#14421=CARTESIAN_POINT('Ctrl Pts',(-0.271805172843737,7.34890367006852,
9.69800341180657E-17));
#14422=CARTESIAN_POINT('Ctrl Pts',(-0.272109971626923,7.35332134308501,
7.35479546497213E-17));
#14423=CARTESIAN_POINT('Ctrl Pts',(-0.272306550140188,7.35775189119246,
7.63278329429795E-17));
#14424=CARTESIAN_POINT('Ctrl Pts',(-0.272509050092771,7.36231589855408,
7.91914481633018E-17));
#14425=CARTESIAN_POINT('Ctrl Pts',(-0.27259625011216,7.3668837741178,8.11349244050912E-17));
#14426=CARTESIAN_POINT('Ctrl Pts',(-0.272569824655828,7.37144896955051,
8.32667268468867E-17));
#14427=CARTESIAN_POINT('Ctrl Pts',(-0.27247174711454,7.38839259912947,9.11788680556787E-17));
#14428=CARTESIAN_POINT('Ctrl Pts',(-0.270813092352919,7.40531022346617,
1.04217775009023E-16));
#14429=CARTESIAN_POINT('Ctrl Pts',(-0.267648460108694,7.42197081815956,
1.14491749414469E-16));
#14430=CARTESIAN_POINT('Ctrl Pts',(-0.265994317828667,7.43067925312638,
1.19861920144093E-16));
#14431=CARTESIAN_POINT('Ctrl Pts',(-0.263927817272562,7.43931723336003,
9.45136624417438E-17));
#14432=CARTESIAN_POINT('Ctrl Pts',(-0.261451366292174,7.44784875840811,
8.67361737988404E-17));
#14433=CARTESIAN_POINT('Ctrl Pts',(-0.260001054064173,7.45284517271178,
8.21813544338432E-17));
#14434=CARTESIAN_POINT('Ctrl Pts',(-0.25840948354909,7.45780668536454,3.82362151915691E-17));
#14435=CARTESIAN_POINT('Ctrl Pts',(-0.25667848349565,7.4627203082836,3.81639164714898E-17));
#14436=CARTESIAN_POINT('Ctrl Pts',(-0.251357933337885,7.47782324091796,
3.79416929274988E-17));
#14437=CARTESIAN_POINT('Ctrl Pts',(-0.244748714237808,7.49240631417947,
4.33000400033759E-17));
#14438=CARTESIAN_POINT('Ctrl Pts',(-0.23687440208594,7.50625495367809,4.16333634234434E-17));
#14439=CARTESIAN_POINT('Ctrl Pts',(-0.232807824863395,7.51340688782321,
4.07726318590114E-17));
#14440=CARTESIAN_POINT('Ctrl Pts',(-0.228399165702,7.52036724850155,8.09844648225997E-17));
#14441=CARTESIAN_POINT('Ctrl Pts',(-0.223669116907964,7.52707485423541,
6.24500451351651E-17));
#14442=CARTESIAN_POINT('Ctrl Pts',(-0.216422990525043,7.53735046892582,
3.40565225020369E-17));
#14443=CARTESIAN_POINT('Ctrl Pts',(-0.208418220052085,7.54704578415416,
-1.68665796639332E-17));
#14444=CARTESIAN_POINT('Ctrl Pts',(-0.199658669018713,7.55604261798761,
-1.38777878078145E-17));
#14445=CARTESIAN_POINT('Ctrl Pts',(-0.197072131758363,7.55869922057452,
-1.99860593395901E-17));
#14446=CARTESIAN_POINT('Ctrl Pts',(-0.194419691364069,7.56129478193143,
-1.04514705227716E-17));
#14447=CARTESIAN_POINT('Ctrl Pts',(-0.191704062602121,7.56382811505057,
-1.38777878078145E-17));
#14448=CARTESIAN_POINT('Origin',(-7.4,0.,-0.45));
#14449=CARTESIAN_POINT('Origin',(7.4,0.,-0.45));
#14450=CARTESIAN_POINT('Origin',(0.,7.4,-0.45));
#14451=CARTESIAN_POINT('Origin',(0.,-7.4,-0.45));
#14452=CARTESIAN_POINT('Origin',(-4.,0.,-2.7));
#14453=CARTESIAN_POINT('',(-4.35,4.28626379701574E-17,-2.4));
#14454=CARTESIAN_POINT('Origin',(-4.,0.,-2.4));
#14455=CARTESIAN_POINT('',(-4.35,4.28626379701574E-17,-3.));
#14456=CARTESIAN_POINT('',(-4.35,4.28626379701574E-17,-2.7));
#14457=CARTESIAN_POINT('Origin',(-4.,0.,-3.));
#14458=CARTESIAN_POINT('Origin',(4.,0.,-2.7));
#14459=CARTESIAN_POINT('',(3.65,4.28626379701574E-17,-2.4));
#14460=CARTESIAN_POINT('Origin',(4.,0.,-2.4));
#14461=CARTESIAN_POINT('',(3.65,4.28626379701574E-17,-3.));
#14462=CARTESIAN_POINT('',(3.65,4.28626379701574E-17,-2.7));
#14463=CARTESIAN_POINT('Origin',(4.,0.,-3.));
#14464=CARTESIAN_POINT('Origin',(0.,4.,-2.7));
#14465=CARTESIAN_POINT('',(-0.35,4.,-2.4));
#14466=CARTESIAN_POINT('Origin',(0.,4.,-2.4));
#14467=CARTESIAN_POINT('',(-0.35,4.,-3.));
#14468=CARTESIAN_POINT('',(-0.35,4.,-2.7));
#14469=CARTESIAN_POINT('Origin',(0.,4.,-3.));
#14470=CARTESIAN_POINT('Origin',(0.,-4.,-2.7));
#14471=CARTESIAN_POINT('',(-0.35,-4.,-2.4));
#14472=CARTESIAN_POINT('Origin',(0.,-4.,-2.4));
#14473=CARTESIAN_POINT('',(-0.35,-4.,-3.));
#14474=CARTESIAN_POINT('',(-0.35,-4.,-2.7));
#14475=CARTESIAN_POINT('Origin',(0.,-4.,-3.));
#14476=CARTESIAN_POINT('Origin',(0.,0.,-2.4));
#14477=CARTESIAN_POINT('',(-4.8,-5.8783046359073E-16,-2.4));
#14478=CARTESIAN_POINT('Origin',(0.,0.,-2.4));
#14479=CARTESIAN_POINT('',(-3.5,-4.28626379701574E-16,-2.4));
#14480=CARTESIAN_POINT('Origin',(0.,0.,-2.4));
#14481=CARTESIAN_POINT('Origin',(0.,0.,-3.));
#14482=CARTESIAN_POINT('',(-4.8,-5.8783046359073E-16,-3.));
#14483=CARTESIAN_POINT('',(-4.8,-5.8783046359073E-16,-3.));
#14484=CARTESIAN_POINT('Origin',(0.,0.,-3.));
#14485=CARTESIAN_POINT('Origin',(0.,0.,-3.));
#14486=CARTESIAN_POINT('',(-2.7,-3.30654635769785E-16,-3.));
#14487=CARTESIAN_POINT('Origin',(0.,0.,-3.));
#14488=CARTESIAN_POINT('Origin',(0.,0.,-2.4));
#14489=CARTESIAN_POINT('',(-3.5,-4.28626379701574E-16,-2.4));
#14490=CARTESIAN_POINT('Origin',(-1.29641016151378,-1.44544826719043,-0.8));
#14491=CARTESIAN_POINT('',(-1.68151315379565,-2.11246621596943,-0.8));
#14492=CARTESIAN_POINT('',(-1.68151315379565,-2.11246621596943,-0.8));
#14493=CARTESIAN_POINT('',(-1.37718656791819,-1.58535710713571,-0.8));
#14494=CARTESIAN_POINT('',(-1.37718656791819,-1.58535710713571,-0.8));
#14495=CARTESIAN_POINT('',(-1.29641016151378,-1.44544826719043,-0.8));
#14496=CARTESIAN_POINT('Origin',(-1.20358983848623,-2.88467875173176,-0.8));
#14497=CARTESIAN_POINT('',(-0.988692830768095,-2.51246621596944,-0.8));
#14498=CARTESIAN_POINT('',(-0.988692830768095,-2.51246621596944,-0.8));
#14499=CARTESIAN_POINT('',(-0.684366244890641,-1.98535710713571,-0.8));
#14500=CARTESIAN_POINT('',(-1.20358983848623,-2.88467875173176,-0.8));
#14501=CARTESIAN_POINT('',(-0.684366244890641,-1.98535710713571,-0.8));
#14502=CARTESIAN_POINT('Origin',(-0.603589838486224,1.84544826719043,-0.8));
#14503=CARTESIAN_POINT('',(-0.988692830768093,2.51246621596944,-0.8));
#14504=CARTESIAN_POINT('',(-0.988692830768093,2.51246621596944,-0.8));
#14505=CARTESIAN_POINT('',(-0.684366244890639,1.98535710713571,-0.8));
#14506=CARTESIAN_POINT('',(-0.684366244890639,1.98535710713571,-0.8));
#14507=CARTESIAN_POINT('',(-0.603589838486224,1.84544826719043,-0.8));
#14508=CARTESIAN_POINT('Origin',(-1.89641016151378,2.48467875173176,-0.8));
#14509=CARTESIAN_POINT('',(-1.68151315379564,2.11246621596944,-0.8));
#14510=CARTESIAN_POINT('',(-1.68151315379564,2.11246621596944,-0.8));
#14511=CARTESIAN_POINT('',(-1.37718656791819,1.58535710713571,-0.8));
#14512=CARTESIAN_POINT('',(-1.89641016151378,2.48467875173176,-0.8));
#14513=CARTESIAN_POINT('',(-1.37718656791819,1.58535710713571,-0.8));
#14514=CARTESIAN_POINT('Origin',(0.,0.,-0.8));
#14515=CARTESIAN_POINT('',(2.67020598456374,-0.4,-0.8));
#14516=CARTESIAN_POINT('',(2.67020598456374,-0.4,-0.8));
#14517=CARTESIAN_POINT('',(2.67020598456374,0.4,-0.8));
#14518=CARTESIAN_POINT('Origin',(0.,0.,-0.8));
#14519=CARTESIAN_POINT('',(2.67020598456374,0.4,-0.8));
#14520=CARTESIAN_POINT('Origin',(0.,0.,-0.8));
#14521=CARTESIAN_POINT('',(-2.7,-3.30654635769785E-16,-0.8));
#14522=CARTESIAN_POINT('Origin',(0.,0.,-0.8));
#14523=CARTESIAN_POINT('Origin',(0.,0.,-0.8));
#14524=CARTESIAN_POINT('',(2.06155281280883,-0.4,-0.8));
#14525=CARTESIAN_POINT('',(1.9,-0.4,-0.8));
#14526=CARTESIAN_POINT('Origin',(0.,0.,-0.8));
#14527=CARTESIAN_POINT('Origin',(0.,0.,-0.8));
#14528=CARTESIAN_POINT('',(2.06155281280883,0.4,-0.8));
#14529=CARTESIAN_POINT('Origin',(0.,0.,-0.8));
#14530=CARTESIAN_POINT('',(3.1,0.4,-0.8));
#14531=CARTESIAN_POINT('',(-1.7,-2.0818995585505E-16,-0.8));
#14532=CARTESIAN_POINT('Origin',(0.,0.,-0.8));
#14533=CARTESIAN_POINT('Origin',(0.,0.,-0.8));
#14534=CARTESIAN_POINT('',(2.06155281280883,0.4,-0.8));
#14535=CARTESIAN_POINT('Origin',(0.,0.,-0.8));
#14536=CARTESIAN_POINT('Origin',(0.,0.,-0.8));
#14537=CARTESIAN_POINT('',(-1.7,-2.0818995585505E-16,-0.8));
#14538=CARTESIAN_POINT('Origin',(0.,0.,-0.8));
#14539=CARTESIAN_POINT('',(2.06155281280883,-0.4,-0.8));
#14540=CARTESIAN_POINT('Origin',(3.1,0.4,-0.8));
#14541=CARTESIAN_POINT('Origin',(0.,0.,0.));
#14542=CARTESIAN_POINT('',(-8.2,-1.00421037530083E-15,0.));
#14543=CARTESIAN_POINT('Origin',(0.,0.,0.));
#14544=CARTESIAN_POINT('Origin',(1.9,-0.4,-0.8));
#14545=CARTESIAN_POINT('Origin',(0.,0.,-0.8));
#14546=CARTESIAN_POINT('',(-8.2,-1.00421037530083E-15,-0.8));
#16651=UNCERTAINTY_MEASURE_WITH_UNIT(LENGTH_MEASURE(0.001),#16688,
'DISTANCE_ACCURACY_VALUE',
'Maximum model space distance between geometric entities at asserted c
onnectivities');
#16666=UNCERTAINTY_MEASURE_WITH_UNIT(LENGTH_MEASURE(0.001),#16688,
'DISTANCE_ACCURACY_VALUE',
'Maximum model space distance between geometric entities at asserted c
onnectivities');
#16672=(
GEOMETRIC_REPRESENTATION_CONTEXT(3)
GLOBAL_UNCERTAINTY_ASSIGNED_CONTEXT((#16651))
GLOBAL_UNIT_ASSIGNED_CONTEXT((#16688,#16690,#16691))
REPRESENTATION_CONTEXT('','3D')
);
#16687=(
GEOMETRIC_REPRESENTATION_CONTEXT(3)
GLOBAL_UNCERTAINTY_ASSIGNED_CONTEXT((#16666))
GLOBAL_UNIT_ASSIGNED_CONTEXT((#16688,#16690,#16691))
REPRESENTATION_CONTEXT('','3D')
);
#16688=(
LENGTH_UNIT()
NAMED_UNIT(*)
SI_UNIT(.CENTI.,.METRE.)
);
#16690=(
NAMED_UNIT(*)
PLANE_ANGLE_UNIT()
SI_UNIT($,.RADIAN.)
);
#16691=(
NAMED_UNIT(*)
SI_UNIT($,.STERADIAN.)
SOLID_ANGLE_UNIT()
);
#16697=SHAPE_DEFINITION_REPRESENTATION(#16717,#16768);
#16717=PRODUCT_DEFINITION_SHAPE('',$,#16789);
#16768=SHAPE_REPRESENTATION('',(#6562),#16672);
#16783=PRODUCT_DEFINITION_CONTEXT('part definition',#16845,'design');
#16789=PRODUCT_DEFINITION('Inlet head','Inlet head',#16809,#16783);
#16809=PRODUCT_DEFINITION_FORMATION('',$,#16852);
#16845=APPLICATION_CONTEXT(
'Core Data for Automotive Mechanical Design Process');
#16846=PRODUCT_CONTEXT('part definition',#16845,'mechanical');
#16852=PRODUCT('Inlet head','Inlet head',$,(#16846));
#16869=PRESENTATION_STYLE_ASSIGNMENT((#16884));
#16884=SURFACE_STYLE_USAGE(.BOTH.,#16899);
#16899=SURFACE_SIDE_STYLE('',(#16914));
#16914=SURFACE_STYLE_FILL_AREA(#16929);
#16929=FILL_AREA_STYLE('Sky blue',(#16944));
#16944=FILL_AREA_STYLE_COLOUR('Sky blue',#16959);
#16959=COLOUR_RGB('Sky blue',0.317647058823529,0.686274509803922,0.890196078431372);
ENDSEC;
END-ISO-10303-21;
